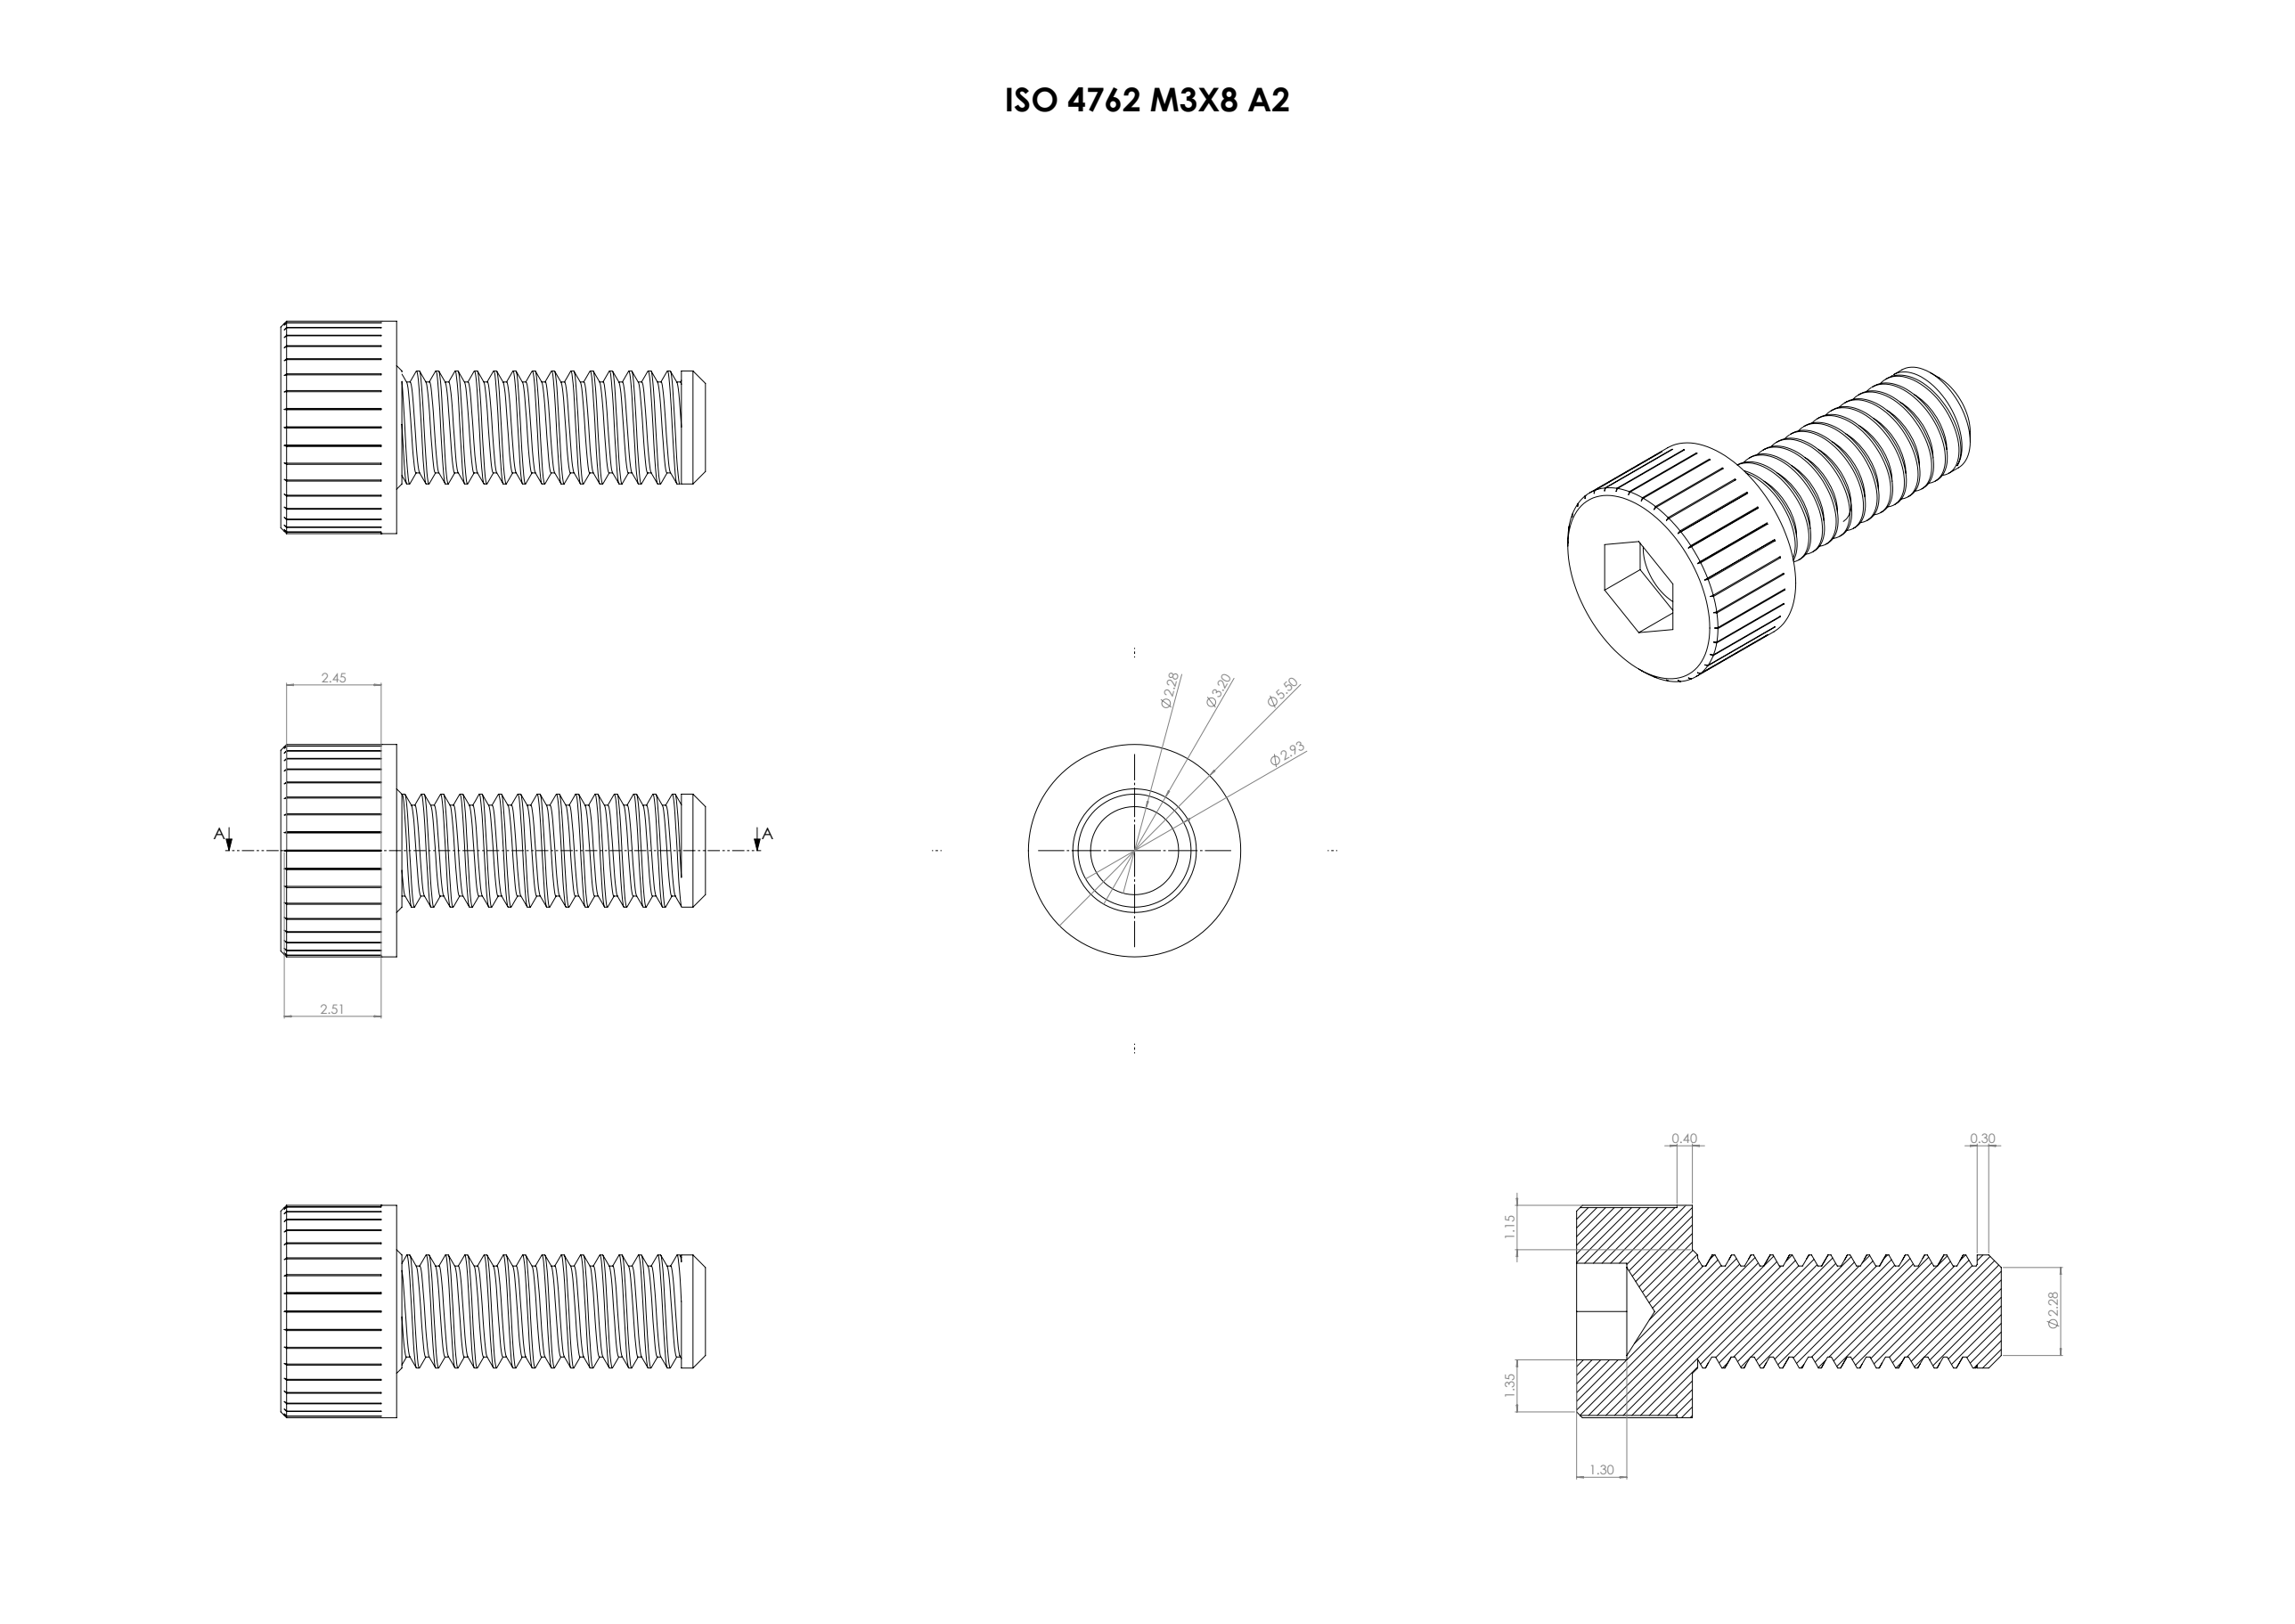
ISO-10303-21;
HEADER;
/* Generated by software containing ST-Developer
 * from STEP Tools, Inc. (www.steptools.com) 
 */

FILE_DESCRIPTION(
/* description */ (''),
/* implementation_level */ '2;1');

FILE_NAME(
/* name */ '14_ISO_4762_M3x8_A2.step',
/* time_stamp */ '2026-10-19T22:59:19-07:00',
/* author */ (''),
/* organization */ (''),
/* preprocessor_version */ 'ST-DEVELOPER v20.2',
/* originating_system */ 'Autodesk Translation Framework v15.15.0.0',
/* authorisation */ '');

FILE_SCHEMA (('AUTOMOTIVE_DESIGN { 1 0 10303 214 3 1 1 }'));
ENDSEC;

DATA;
#10=MECHANICAL_DESIGN_GEOMETRIC_PRESENTATION_REPRESENTATION('',(#924),#53650);
#147=(
BOUNDED_CURVE()
B_SPLINE_CURVE(2,(#40816,#40817,#40818),.UNSPECIFIED.,.F.,.F.)
B_SPLINE_CURVE_WITH_KNOTS((3,3),(0.,0.00848409808460555),.UNSPECIFIED.)
CURVE()
GEOMETRIC_REPRESENTATION_ITEM()
RATIONAL_B_SPLINE_CURVE((1.,1.00016582969981,1.00020138402525))
REPRESENTATION_ITEM('')
);
#148=(
BOUNDED_CURVE()
B_SPLINE_CURVE(2,(#40822,#40823,#40824),.UNSPECIFIED.,.F.,.F.)
B_SPLINE_CURVE_WITH_KNOTS((3,3),(0.0131150022108642,0.0215991002954745),
 .UNSPECIFIED.)
CURVE()
GEOMETRIC_REPRESENTATION_ITEM()
RATIONAL_B_SPLINE_CURVE((1.0002013840307,1.00016582970429,1.))
REPRESENTATION_ITEM('')
);
#149=(
BOUNDED_CURVE()
B_SPLINE_CURVE(2,(#40837,#40838,#40839),.UNSPECIFIED.,.F.,.F.)
B_SPLINE_CURVE_WITH_KNOTS((3,3),(0.,0.0084840980845983),.UNSPECIFIED.)
CURVE()
GEOMETRIC_REPRESENTATION_ITEM()
RATIONAL_B_SPLINE_CURVE((1.,1.00016582970166,1.00020138402749))
REPRESENTATION_ITEM('')
);
#150=(
BOUNDED_CURVE()
B_SPLINE_CURVE(2,(#40843,#40844,#40845),.UNSPECIFIED.,.F.,.F.)
B_SPLINE_CURVE_WITH_KNOTS((3,3),(0.0131150022108621,0.0215991002954745),
 .UNSPECIFIED.)
CURVE()
GEOMETRIC_REPRESENTATION_ITEM()
RATIONAL_B_SPLINE_CURVE((1.00020138404061,1.00016582971246,1.))
REPRESENTATION_ITEM('')
);
#151=(
BOUNDED_CURVE()
B_SPLINE_CURVE(2,(#40858,#40859,#40860),.UNSPECIFIED.,.F.,.F.)
B_SPLINE_CURVE_WITH_KNOTS((3,3),(0.,0.0084840980847528),.UNSPECIFIED.)
CURVE()
GEOMETRIC_REPRESENTATION_ITEM()
RATIONAL_B_SPLINE_CURVE((1.,1.00016582970549,1.00020138403215))
REPRESENTATION_ITEM('')
);
#152=(
BOUNDED_CURVE()
B_SPLINE_CURVE(2,(#40864,#40865,#40866),.UNSPECIFIED.,.F.,.F.)
B_SPLINE_CURVE_WITH_KNOTS((3,3),(0.0131150022108369,0.0215991002954744),
 .UNSPECIFIED.)
CURVE()
GEOMETRIC_REPRESENTATION_ITEM()
RATIONAL_B_SPLINE_CURVE((1.00020138403309,1.00016582970627,1.))
REPRESENTATION_ITEM('')
);
#153=(
BOUNDED_CURVE()
B_SPLINE_CURVE(2,(#40879,#40880,#40881),.UNSPECIFIED.,.F.,.F.)
B_SPLINE_CURVE_WITH_KNOTS((3,3),(0.,0.00848409808456441),.UNSPECIFIED.)
CURVE()
GEOMETRIC_REPRESENTATION_ITEM()
RATIONAL_B_SPLINE_CURVE((1.,1.00016582971128,1.00020138403918))
REPRESENTATION_ITEM('')
);
#154=(
BOUNDED_CURVE()
B_SPLINE_CURVE(2,(#40885,#40886,#40887),.UNSPECIFIED.,.F.,.F.)
B_SPLINE_CURVE_WITH_KNOTS((3,3),(0.0131150022107445,0.0215991002954745),
 .UNSPECIFIED.)
CURVE()
GEOMETRIC_REPRESENTATION_ITEM()
RATIONAL_B_SPLINE_CURVE((1.00020138401994,1.00016582969544,1.))
REPRESENTATION_ITEM('')
);
#155=(
BOUNDED_CURVE()
B_SPLINE_CURVE(2,(#40900,#40901,#40902),.UNSPECIFIED.,.F.,.F.)
B_SPLINE_CURVE_WITH_KNOTS((3,3),(0.,0.00848409808454028),.UNSPECIFIED.)
CURVE()
GEOMETRIC_REPRESENTATION_ITEM()
RATIONAL_B_SPLINE_CURVE((1.,1.00016582970383,1.00020138403013))
REPRESENTATION_ITEM('')
);
#156=(
BOUNDED_CURVE()
B_SPLINE_CURVE(2,(#40906,#40907,#40908),.UNSPECIFIED.,.F.,.F.)
B_SPLINE_CURVE_WITH_KNOTS((3,3),(0.0131150022108609,0.0215991002954744),
 .UNSPECIFIED.)
CURVE()
GEOMETRIC_REPRESENTATION_ITEM()
RATIONAL_B_SPLINE_CURVE((1.00020138403313,1.0001658297063,1.))
REPRESENTATION_ITEM('')
);
#157=(
BOUNDED_CURVE()
B_SPLINE_CURVE(2,(#40921,#40922,#40923),.UNSPECIFIED.,.F.,.F.)
B_SPLINE_CURVE_WITH_KNOTS((3,3),(0.,0.00848409808447202),.UNSPECIFIED.)
CURVE()
GEOMETRIC_REPRESENTATION_ITEM()
RATIONAL_B_SPLINE_CURVE((1.,1.00016582970768,1.00020138403481))
REPRESENTATION_ITEM('')
);
#158=(
BOUNDED_CURVE()
B_SPLINE_CURVE(2,(#40927,#40928,#40929),.UNSPECIFIED.,.F.,.F.)
B_SPLINE_CURVE_WITH_KNOTS((3,3),(0.0131150022108224,0.0215991002954744),
 .UNSPECIFIED.)
CURVE()
GEOMETRIC_REPRESENTATION_ITEM()
RATIONAL_B_SPLINE_CURVE((1.00020138403609,1.00016582970874,1.))
REPRESENTATION_ITEM('')
);
#159=(
BOUNDED_CURVE()
B_SPLINE_CURVE(2,(#40942,#40943,#40944),.UNSPECIFIED.,.F.,.F.)
B_SPLINE_CURVE_WITH_KNOTS((3,3),(0.,0.00848409808427833),.UNSPECIFIED.)
CURVE()
GEOMETRIC_REPRESENTATION_ITEM()
RATIONAL_B_SPLINE_CURVE((1.,1.00016582970634,1.00020138403319))
REPRESENTATION_ITEM('')
);
#160=(
BOUNDED_CURVE()
B_SPLINE_CURVE(2,(#40948,#40949,#40950),.UNSPECIFIED.,.F.,.F.)
B_SPLINE_CURVE_WITH_KNOTS((3,3),(0.013115002210556,0.0215991002954744),
 .UNSPECIFIED.)
CURVE()
GEOMETRIC_REPRESENTATION_ITEM()
RATIONAL_B_SPLINE_CURVE((1.00020138403007,1.00016582970378,1.))
REPRESENTATION_ITEM('')
);
#161=(
BOUNDED_CURVE()
B_SPLINE_CURVE(2,(#40963,#40964,#40965),.UNSPECIFIED.,.F.,.F.)
B_SPLINE_CURVE_WITH_KNOTS((3,3),(0.,0.00848409808441644),.UNSPECIFIED.)
CURVE()
GEOMETRIC_REPRESENTATION_ITEM()
RATIONAL_B_SPLINE_CURVE((1.,1.00016582971078,1.00020138403858))
REPRESENTATION_ITEM('')
);
#162=(
BOUNDED_CURVE()
B_SPLINE_CURVE(2,(#40969,#40970,#40971),.UNSPECIFIED.,.F.,.F.)
B_SPLINE_CURVE_WITH_KNOTS((3,3),(0.0131150022111809,0.0215991002954744),
 .UNSPECIFIED.)
CURVE()
GEOMETRIC_REPRESENTATION_ITEM()
RATIONAL_B_SPLINE_CURVE((1.00020138403856,1.00016582971077,1.))
REPRESENTATION_ITEM('')
);
#163=(
BOUNDED_CURVE()
B_SPLINE_CURVE(2,(#40984,#40985,#40986),.UNSPECIFIED.,.F.,.F.)
B_SPLINE_CURVE_WITH_KNOTS((3,3),(0.,0.00848409808461716),.UNSPECIFIED.)
CURVE()
GEOMETRIC_REPRESENTATION_ITEM()
RATIONAL_B_SPLINE_CURVE((1.,1.00016582970495,1.00020138403149))
REPRESENTATION_ITEM('')
);
#164=(
BOUNDED_CURVE()
B_SPLINE_CURVE(2,(#40990,#40991,#40992),.UNSPECIFIED.,.F.,.F.)
B_SPLINE_CURVE_WITH_KNOTS((3,3),(0.0131150022109262,0.0215991002954744),
 .UNSPECIFIED.)
CURVE()
GEOMETRIC_REPRESENTATION_ITEM()
RATIONAL_B_SPLINE_CURVE((1.00020138404239,1.00016582971392,1.))
REPRESENTATION_ITEM('')
);
#165=(
BOUNDED_CURVE()
B_SPLINE_CURVE(2,(#41005,#41006,#41007),.UNSPECIFIED.,.F.,.F.)
B_SPLINE_CURVE_WITH_KNOTS((3,3),(0.,0.00848409808431464),.UNSPECIFIED.)
CURVE()
GEOMETRIC_REPRESENTATION_ITEM()
RATIONAL_B_SPLINE_CURVE((1.,1.00016582970871,1.00020138403606))
REPRESENTATION_ITEM('')
);
#166=(
BOUNDED_CURVE()
B_SPLINE_CURVE(2,(#41011,#41012,#41013),.UNSPECIFIED.,.F.,.F.)
B_SPLINE_CURVE_WITH_KNOTS((3,3),(0.0131150022106601,0.0215991002954745),
 .UNSPECIFIED.)
CURVE()
GEOMETRIC_REPRESENTATION_ITEM()
RATIONAL_B_SPLINE_CURVE((1.00020138402617,1.00016582970057,1.))
REPRESENTATION_ITEM('')
);
#167=(
BOUNDED_CURVE()
B_SPLINE_CURVE(2,(#41026,#41027,#41028),.UNSPECIFIED.,.F.,.F.)
B_SPLINE_CURVE_WITH_KNOTS((3,3),(0.,0.00848409808479875),.UNSPECIFIED.)
CURVE()
GEOMETRIC_REPRESENTATION_ITEM()
RATIONAL_B_SPLINE_CURVE((1.,1.00016582970535,1.00020138403197))
REPRESENTATION_ITEM('')
);
#168=(
BOUNDED_CURVE()
B_SPLINE_CURVE(2,(#41032,#41033,#41034),.UNSPECIFIED.,.F.,.F.)
B_SPLINE_CURVE_WITH_KNOTS((3,3),(0.0131150022108306,0.0215991002954744),
 .UNSPECIFIED.)
CURVE()
GEOMETRIC_REPRESENTATION_ITEM()
RATIONAL_B_SPLINE_CURVE((1.00020138403405,1.00016582970706,1.))
REPRESENTATION_ITEM('')
);
#169=(
BOUNDED_CURVE()
B_SPLINE_CURVE(2,(#41047,#41048,#41049),.UNSPECIFIED.,.F.,.F.)
B_SPLINE_CURVE_WITH_KNOTS((3,3),(0.,0.0084840980847528),.UNSPECIFIED.)
CURVE()
GEOMETRIC_REPRESENTATION_ITEM()
RATIONAL_B_SPLINE_CURVE((1.,1.00016582970549,1.00020138403215))
REPRESENTATION_ITEM('')
);
#170=(
BOUNDED_CURVE()
B_SPLINE_CURVE(2,(#41053,#41054,#41055),.UNSPECIFIED.,.F.,.F.)
B_SPLINE_CURVE_WITH_KNOTS((3,3),(0.0131150022108369,0.0215991002954744),
 .UNSPECIFIED.)
CURVE()
GEOMETRIC_REPRESENTATION_ITEM()
RATIONAL_B_SPLINE_CURVE((1.00020138403309,1.00016582970627,1.))
REPRESENTATION_ITEM('')
);
#171=(
BOUNDED_CURVE()
B_SPLINE_CURVE(2,(#41068,#41069,#41070),.UNSPECIFIED.,.F.,.F.)
B_SPLINE_CURVE_WITH_KNOTS((3,3),(0.,0.0084840980842322),.UNSPECIFIED.)
CURVE()
GEOMETRIC_REPRESENTATION_ITEM()
RATIONAL_B_SPLINE_CURVE((1.,1.00016582971394,1.00020138404241))
REPRESENTATION_ITEM('')
);
#172=(
BOUNDED_CURVE()
B_SPLINE_CURVE(2,(#41074,#41075,#41076),.UNSPECIFIED.,.F.,.F.)
B_SPLINE_CURVE_WITH_KNOTS((3,3),(0.0131150022105481,0.0215991002954744),
 .UNSPECIFIED.)
CURVE()
GEOMETRIC_REPRESENTATION_ITEM()
RATIONAL_B_SPLINE_CURVE((1.00020138402709,1.00016582970133,1.))
REPRESENTATION_ITEM('')
);
#173=(
BOUNDED_CURVE()
B_SPLINE_CURVE(2,(#41089,#41090,#41091),.UNSPECIFIED.,.F.,.F.)
B_SPLINE_CURVE_WITH_KNOTS((3,3),(0.,0.00848409808414784),.UNSPECIFIED.)
CURVE()
GEOMETRIC_REPRESENTATION_ITEM()
RATIONAL_B_SPLINE_CURVE((1.,1.00016582970969,1.00020138403725))
REPRESENTATION_ITEM('')
);
#174=(
BOUNDED_CURVE()
B_SPLINE_CURVE(2,(#41095,#41096,#41097),.UNSPECIFIED.,.F.,.F.)
B_SPLINE_CURVE_WITH_KNOTS((3,3),(0.0131150022106295,0.0215991002954744),
 .UNSPECIFIED.)
CURVE()
GEOMETRIC_REPRESENTATION_ITEM()
RATIONAL_B_SPLINE_CURVE((1.00020138402686,1.00016582970114,1.))
REPRESENTATION_ITEM('')
);
#175=(
BOUNDED_CURVE()
B_SPLINE_CURVE(2,(#41110,#41111,#41112),.UNSPECIFIED.,.F.,.F.)
B_SPLINE_CURVE_WITH_KNOTS((3,3),(0.,0.00848409808445945),.UNSPECIFIED.)
CURVE()
GEOMETRIC_REPRESENTATION_ITEM()
RATIONAL_B_SPLINE_CURVE((1.,1.00016582971029,1.00020138403798))
REPRESENTATION_ITEM('')
);
#176=(
BOUNDED_CURVE()
B_SPLINE_CURVE(2,(#41116,#41117,#41118),.UNSPECIFIED.,.F.,.F.)
B_SPLINE_CURVE_WITH_KNOTS((3,3),(0.0131150022108553,0.0215991002954744),
 .UNSPECIFIED.)
CURVE()
GEOMETRIC_REPRESENTATION_ITEM()
RATIONAL_B_SPLINE_CURVE((1.00020138402807,1.00016582970213,1.))
REPRESENTATION_ITEM('')
);
#177=(
BOUNDED_CURVE()
B_SPLINE_CURVE(2,(#41131,#41132,#41133),.UNSPECIFIED.,.F.,.F.)
B_SPLINE_CURVE_WITH_KNOTS((3,3),(0.,0.00848409808448244),.UNSPECIFIED.)
CURVE()
GEOMETRIC_REPRESENTATION_ITEM()
RATIONAL_B_SPLINE_CURVE((1.,1.00016582970044,1.00020138402602))
REPRESENTATION_ITEM('')
);
#178=(
BOUNDED_CURVE()
B_SPLINE_CURVE(2,(#41137,#41138,#41139),.UNSPECIFIED.,.F.,.F.)
B_SPLINE_CURVE_WITH_KNOTS((3,3),(0.0131150022107,0.0215991002954745),
 .UNSPECIFIED.)
CURVE()
GEOMETRIC_REPRESENTATION_ITEM()
RATIONAL_B_SPLINE_CURVE((1.00020138402745,1.00016582970163,1.))
REPRESENTATION_ITEM('')
);
#179=(
BOUNDED_CURVE()
B_SPLINE_CURVE(2,(#41152,#41153,#41154),.UNSPECIFIED.,.F.,.F.)
B_SPLINE_CURVE_WITH_KNOTS((3,3),(0.,0.0084840980844404),.UNSPECIFIED.)
CURVE()
GEOMETRIC_REPRESENTATION_ITEM()
RATIONAL_B_SPLINE_CURVE((1.,1.00016582969984,1.00020138402529))
REPRESENTATION_ITEM('')
);
#180=(
BOUNDED_CURVE()
B_SPLINE_CURVE(2,(#41158,#41159,#41160),.UNSPECIFIED.,.F.,.F.)
B_SPLINE_CURVE_WITH_KNOTS((3,3),(0.0131150022109728,0.0215991002954744),
 .UNSPECIFIED.)
CURVE()
GEOMETRIC_REPRESENTATION_ITEM()
RATIONAL_B_SPLINE_CURVE((1.00020138403593,1.0001658297086,1.))
REPRESENTATION_ITEM('')
);
#181=(
BOUNDED_CURVE()
B_SPLINE_CURVE(2,(#41175,#41176,#41177),.UNSPECIFIED.,.F.,.F.)
B_SPLINE_CURVE_WITH_KNOTS((3,3),(0.,0.00848409808461716),.UNSPECIFIED.)
CURVE()
GEOMETRIC_REPRESENTATION_ITEM()
RATIONAL_B_SPLINE_CURVE((1.,1.00016582970494,1.00020138403149))
REPRESENTATION_ITEM('')
);
#182=(
BOUNDED_CURVE()
B_SPLINE_CURVE(2,(#41181,#41182,#41183),.UNSPECIFIED.,.F.,.F.)
B_SPLINE_CURVE_WITH_KNOTS((3,3),(0.0131150022107313,0.0215991002954744),
 .UNSPECIFIED.)
CURVE()
GEOMETRIC_REPRESENTATION_ITEM()
RATIONAL_B_SPLINE_CURVE((1.00020138404435,1.00016582971554,1.))
REPRESENTATION_ITEM('')
);
#183=(
BOUNDED_CURVE()
B_SPLINE_CURVE(2,(#41196,#41197,#41198),.UNSPECIFIED.,.F.,.F.)
B_SPLINE_CURVE_WITH_KNOTS((3,3),(0.,0.0084840980847339),.UNSPECIFIED.)
CURVE()
GEOMETRIC_REPRESENTATION_ITEM()
RATIONAL_B_SPLINE_CURVE((1.,1.00016582970597,1.00020138403273))
REPRESENTATION_ITEM('')
);
#184=(
BOUNDED_CURVE()
B_SPLINE_CURVE(2,(#41202,#41203,#41204),.UNSPECIFIED.,.F.,.F.)
B_SPLINE_CURVE_WITH_KNOTS((3,3),(0.0131150022106966,0.0215991002954744),
 .UNSPECIFIED.)
CURVE()
GEOMETRIC_REPRESENTATION_ITEM()
RATIONAL_B_SPLINE_CURVE((1.00020138403392,1.00016582970695,1.))
REPRESENTATION_ITEM('')
);
#185=(
BOUNDED_CURVE()
B_SPLINE_CURVE(2,(#41217,#41218,#41219),.UNSPECIFIED.,.F.,.F.)
B_SPLINE_CURVE_WITH_KNOTS((3,3),(0.,0.00848409808458664),.UNSPECIFIED.)
CURVE()
GEOMETRIC_REPRESENTATION_ITEM()
RATIONAL_B_SPLINE_CURVE((1.,1.00016582970477,1.00020138403127))
REPRESENTATION_ITEM('')
);
#186=(
BOUNDED_CURVE()
B_SPLINE_CURVE(2,(#41223,#41224,#41225),.UNSPECIFIED.,.F.,.F.)
B_SPLINE_CURVE_WITH_KNOTS((3,3),(0.0131150022108393,0.0215991002954745),
 .UNSPECIFIED.)
CURVE()
GEOMETRIC_REPRESENTATION_ITEM()
RATIONAL_B_SPLINE_CURVE((1.00020138403572,1.00016582970843,1.))
REPRESENTATION_ITEM('')
);
#187=(
BOUNDED_CURVE()
B_SPLINE_CURVE(2,(#41238,#41239,#41240),.UNSPECIFIED.,.F.,.F.)
B_SPLINE_CURVE_WITH_KNOTS((3,3),(0.,0.00848409808463718),.UNSPECIFIED.)
CURVE()
GEOMETRIC_REPRESENTATION_ITEM()
RATIONAL_B_SPLINE_CURVE((1.,1.00016582970055,1.00020138402615))
REPRESENTATION_ITEM('')
);
#188=(
BOUNDED_CURVE()
B_SPLINE_CURVE(2,(#41244,#41245,#41246),.UNSPECIFIED.,.F.,.F.)
B_SPLINE_CURVE_WITH_KNOTS((3,3),(0.013115002211021,0.0215991002954743),
 .UNSPECIFIED.)
CURVE()
GEOMETRIC_REPRESENTATION_ITEM()
RATIONAL_B_SPLINE_CURVE((1.00020138403351,1.00016582970661,1.))
REPRESENTATION_ITEM('')
);
#189=(
BOUNDED_CURVE()
B_SPLINE_CURVE(2,(#41259,#41260,#41261),.UNSPECIFIED.,.F.,.F.)
B_SPLINE_CURVE_WITH_KNOTS((3,3),(0.,0.0084840980842322),.UNSPECIFIED.)
CURVE()
GEOMETRIC_REPRESENTATION_ITEM()
RATIONAL_B_SPLINE_CURVE((1.,1.00016582971394,1.00020138404241))
REPRESENTATION_ITEM('')
);
#190=(
BOUNDED_CURVE()
B_SPLINE_CURVE(2,(#41265,#41266,#41267),.UNSPECIFIED.,.F.,.F.)
B_SPLINE_CURVE_WITH_KNOTS((3,3),(0.0131150022105481,0.0215991002954744),
 .UNSPECIFIED.)
CURVE()
GEOMETRIC_REPRESENTATION_ITEM()
RATIONAL_B_SPLINE_CURVE((1.00020138402709,1.00016582970133,1.))
REPRESENTATION_ITEM('')
);
#191=(
BOUNDED_CURVE()
B_SPLINE_CURVE(2,(#41280,#41281,#41282),.UNSPECIFIED.,.F.,.F.)
B_SPLINE_CURVE_WITH_KNOTS((3,3),(0.,0.00848409808456074),.UNSPECIFIED.)
CURVE()
GEOMETRIC_REPRESENTATION_ITEM()
RATIONAL_B_SPLINE_CURVE((1.,1.00016582970947,1.00020138403699))
REPRESENTATION_ITEM('')
);
#192=(
BOUNDED_CURVE()
B_SPLINE_CURVE(2,(#41286,#41287,#41288),.UNSPECIFIED.,.F.,.F.)
B_SPLINE_CURVE_WITH_KNOTS((3,3),(0.0131150022109338,0.0215991002954745),
 .UNSPECIFIED.)
CURVE()
GEOMETRIC_REPRESENTATION_ITEM()
RATIONAL_B_SPLINE_CURVE((1.00020138403466,1.00016582970756,1.))
REPRESENTATION_ITEM('')
);
#193=(
BOUNDED_CURVE()
B_SPLINE_CURVE(2,(#41301,#41302,#41303),.UNSPECIFIED.,.F.,.F.)
B_SPLINE_CURVE_WITH_KNOTS((3,3),(0.,0.00848409808446819),.UNSPECIFIED.)
CURVE()
GEOMETRIC_REPRESENTATION_ITEM()
RATIONAL_B_SPLINE_CURVE((1.,1.00016582970737,1.00020138403444))
REPRESENTATION_ITEM('')
);
#194=(
BOUNDED_CURVE()
B_SPLINE_CURVE(2,(#41307,#41308,#41309),.UNSPECIFIED.,.F.,.F.)
B_SPLINE_CURVE_WITH_KNOTS((3,3),(0.0131150022107308,0.0215991002954744),
 .UNSPECIFIED.)
CURVE()
GEOMETRIC_REPRESENTATION_ITEM()
RATIONAL_B_SPLINE_CURVE((1.00020138402973,1.0001658297035,1.))
REPRESENTATION_ITEM('')
);
#195=(
BOUNDED_CURVE()
B_SPLINE_CURVE(2,(#41322,#41323,#41324),.UNSPECIFIED.,.F.,.F.)
B_SPLINE_CURVE_WITH_KNOTS((3,3),(0.,0.00848409808448244),.UNSPECIFIED.)
CURVE()
GEOMETRIC_REPRESENTATION_ITEM()
RATIONAL_B_SPLINE_CURVE((1.,1.00016582970044,1.00020138402602))
REPRESENTATION_ITEM('')
);
#196=(
BOUNDED_CURVE()
B_SPLINE_CURVE(2,(#41328,#41329,#41330),.UNSPECIFIED.,.F.,.F.)
B_SPLINE_CURVE_WITH_KNOTS((3,3),(0.0131150022107,0.0215991002954745),
 .UNSPECIFIED.)
CURVE()
GEOMETRIC_REPRESENTATION_ITEM()
RATIONAL_B_SPLINE_CURVE((1.00020138402745,1.00016582970163,1.))
REPRESENTATION_ITEM('')
);
#197=(
BOUNDED_CURVE()
B_SPLINE_CURVE(2,(#41343,#41344,#41345),.UNSPECIFIED.,.F.,.F.)
B_SPLINE_CURVE_WITH_KNOTS((3,3),(0.,0.00848409808441086),.UNSPECIFIED.)
CURVE()
GEOMETRIC_REPRESENTATION_ITEM()
RATIONAL_B_SPLINE_CURVE((1.,1.00016582971069,1.00020138403846))
REPRESENTATION_ITEM('')
);
#198=(
BOUNDED_CURVE()
B_SPLINE_CURVE(2,(#41349,#41350,#41351),.UNSPECIFIED.,.F.,.F.)
B_SPLINE_CURVE_WITH_KNOTS((3,3),(0.0131150022109839,0.0215991002954745),
 .UNSPECIFIED.)
CURVE()
GEOMETRIC_REPRESENTATION_ITEM()
RATIONAL_B_SPLINE_CURVE((1.00020138402514,1.00016582969972,1.))
REPRESENTATION_ITEM('')
);
#199=(
BOUNDED_CURVE()
B_SPLINE_CURVE(2,(#41364,#41365,#41366),.UNSPECIFIED.,.F.,.F.)
B_SPLINE_CURVE_WITH_KNOTS((3,3),(0.,0.00848409808461089),.UNSPECIFIED.)
CURVE()
GEOMETRIC_REPRESENTATION_ITEM()
RATIONAL_B_SPLINE_CURVE((1.,1.00016582970996,1.00020138403757))
REPRESENTATION_ITEM('')
);
#200=(
BOUNDED_CURVE()
B_SPLINE_CURVE(2,(#41370,#41371,#41372),.UNSPECIFIED.,.F.,.F.)
B_SPLINE_CURVE_WITH_KNOTS((3,3),(0.0131150022107081,0.0215991002954744),
 .UNSPECIFIED.)
CURVE()
GEOMETRIC_REPRESENTATION_ITEM()
RATIONAL_B_SPLINE_CURVE((1.00020138403464,1.00016582970754,1.))
REPRESENTATION_ITEM('')
);
#201=(
BOUNDED_CURVE()
B_SPLINE_CURVE(2,(#41385,#41386,#41387),.UNSPECIFIED.,.F.,.F.)
B_SPLINE_CURVE_WITH_KNOTS((3,3),(0.,0.00848409808429742),.UNSPECIFIED.)
CURVE()
GEOMETRIC_REPRESENTATION_ITEM()
RATIONAL_B_SPLINE_CURVE((1.,1.00016582971405,1.00020138404255))
REPRESENTATION_ITEM('')
);
#202=(
BOUNDED_CURVE()
B_SPLINE_CURVE(2,(#41391,#41392,#41393),.UNSPECIFIED.,.F.,.F.)
B_SPLINE_CURVE_WITH_KNOTS((3,3),(0.0131150022109026,0.0215991002954744),
 .UNSPECIFIED.)
CURVE()
GEOMETRIC_REPRESENTATION_ITEM()
RATIONAL_B_SPLINE_CURVE((1.00020138403953,1.00016582971157,1.))
REPRESENTATION_ITEM('')
);
#203=(
BOUNDED_CURVE()
B_SPLINE_CURVE(2,(#41406,#41407,#41408),.UNSPECIFIED.,.F.,.F.)
B_SPLINE_CURVE_WITH_KNOTS((3,3),(0.,0.00848409808458664),.UNSPECIFIED.)
CURVE()
GEOMETRIC_REPRESENTATION_ITEM()
RATIONAL_B_SPLINE_CURVE((1.,1.00016582970477,1.00020138403127))
REPRESENTATION_ITEM('')
);
#204=(
BOUNDED_CURVE()
B_SPLINE_CURVE(2,(#41412,#41413,#41414),.UNSPECIFIED.,.F.,.F.)
B_SPLINE_CURVE_WITH_KNOTS((3,3),(0.0131150022108393,0.0215991002954745),
 .UNSPECIFIED.)
CURVE()
GEOMETRIC_REPRESENTATION_ITEM()
RATIONAL_B_SPLINE_CURVE((1.00020138403572,1.00016582970843,1.))
REPRESENTATION_ITEM('')
);
#205=(
BOUNDED_CURVE()
B_SPLINE_CURVE(2,(#41427,#41428,#41429),.UNSPECIFIED.,.F.,.F.)
B_SPLINE_CURVE_WITH_KNOTS((3,3),(0.,0.00848409808472772),.UNSPECIFIED.)
CURVE()
GEOMETRIC_REPRESENTATION_ITEM()
RATIONAL_B_SPLINE_CURVE((1.,1.00016582970133,1.0002013840271))
REPRESENTATION_ITEM('')
);
#206=(
BOUNDED_CURVE()
B_SPLINE_CURVE(2,(#41433,#41434,#41435),.UNSPECIFIED.,.F.,.F.)
B_SPLINE_CURVE_WITH_KNOTS((3,3),(0.0131150022106421,0.0215991002954744),
 .UNSPECIFIED.)
CURVE()
GEOMETRIC_REPRESENTATION_ITEM()
RATIONAL_B_SPLINE_CURVE((1.00020138403214,1.00016582970549,1.))
REPRESENTATION_ITEM('')
);
#207=(
BOUNDED_CURVE()
B_SPLINE_CURVE(2,(#41448,#41449,#41450),.UNSPECIFIED.,.F.,.F.)
B_SPLINE_CURVE_WITH_KNOTS((3,3),(0.,0.00848409808461495),.UNSPECIFIED.)
CURVE()
GEOMETRIC_REPRESENTATION_ITEM()
RATIONAL_B_SPLINE_CURVE((1.,1.00016582970949,1.000201384037))
REPRESENTATION_ITEM('')
);
#208=(
BOUNDED_CURVE()
B_SPLINE_CURVE(2,(#41454,#41455,#41456),.UNSPECIFIED.,.F.,.F.)
B_SPLINE_CURVE_WITH_KNOTS((3,3),(0.0131150022109445,0.0215991002954744),
 .UNSPECIFIED.)
CURVE()
GEOMETRIC_REPRESENTATION_ITEM()
RATIONAL_B_SPLINE_CURVE((1.00020138402523,1.00016582969979,1.))
REPRESENTATION_ITEM('')
);
#209=(
BOUNDED_CURVE()
B_SPLINE_CURVE(2,(#41469,#41470,#41471),.UNSPECIFIED.,.F.,.F.)
B_SPLINE_CURVE_WITH_KNOTS((3,3),(0.,0.00848409808414784),.UNSPECIFIED.)
CURVE()
GEOMETRIC_REPRESENTATION_ITEM()
RATIONAL_B_SPLINE_CURVE((1.,1.00016582970969,1.00020138403725))
REPRESENTATION_ITEM('')
);
#210=(
BOUNDED_CURVE()
B_SPLINE_CURVE(2,(#41475,#41476,#41477),.UNSPECIFIED.,.F.,.F.)
B_SPLINE_CURVE_WITH_KNOTS((3,3),(0.0131150022106295,0.0215991002954744),
 .UNSPECIFIED.)
CURVE()
GEOMETRIC_REPRESENTATION_ITEM()
RATIONAL_B_SPLINE_CURVE((1.00020138402686,1.00016582970114,1.))
REPRESENTATION_ITEM('')
);
#211=(
BOUNDED_CURVE()
B_SPLINE_CURVE(2,(#41490,#41491,#41492),.UNSPECIFIED.,.F.,.F.)
B_SPLINE_CURVE_WITH_KNOTS((3,3),(0.,0.00848409808467215),.UNSPECIFIED.)
CURVE()
GEOMETRIC_REPRESENTATION_ITEM()
RATIONAL_B_SPLINE_CURVE((1.,1.00016582970831,1.00020138403558))
REPRESENTATION_ITEM('')
);
#212=(
BOUNDED_CURVE()
B_SPLINE_CURVE(2,(#41496,#41497,#41498),.UNSPECIFIED.,.F.,.F.)
B_SPLINE_CURVE_WITH_KNOTS((3,3),(0.0131150022106657,0.0215991002954744),
 .UNSPECIFIED.)
CURVE()
GEOMETRIC_REPRESENTATION_ITEM()
RATIONAL_B_SPLINE_CURVE((1.00020138402665,1.00016582970096,1.))
REPRESENTATION_ITEM('')
);
#213=(
BOUNDED_CURVE()
B_SPLINE_CURVE(2,(#41511,#41512,#41513),.UNSPECIFIED.,.F.,.F.)
B_SPLINE_CURVE_WITH_KNOTS((3,3),(0.,0.00848409808448244),.UNSPECIFIED.)
CURVE()
GEOMETRIC_REPRESENTATION_ITEM()
RATIONAL_B_SPLINE_CURVE((1.,1.00016582970044,1.00020138402602))
REPRESENTATION_ITEM('')
);
#214=(
BOUNDED_CURVE()
B_SPLINE_CURVE(2,(#41517,#41518,#41519),.UNSPECIFIED.,.F.,.F.)
B_SPLINE_CURVE_WITH_KNOTS((3,3),(0.0131150022107,0.0215991002954745),
 .UNSPECIFIED.)
CURVE()
GEOMETRIC_REPRESENTATION_ITEM()
RATIONAL_B_SPLINE_CURVE((1.00020138402745,1.00016582970163,1.))
REPRESENTATION_ITEM('')
);
#215=(
BOUNDED_CURVE()
B_SPLINE_CURVE(2,(#41532,#41533,#41534),.UNSPECIFIED.,.F.,.F.)
B_SPLINE_CURVE_WITH_KNOTS((3,3),(0.,0.00848409808462521),.UNSPECIFIED.)
CURVE()
GEOMETRIC_REPRESENTATION_ITEM()
RATIONAL_B_SPLINE_CURVE((1.,1.00016582970203,1.00020138402795))
REPRESENTATION_ITEM('')
);
#216=(
BOUNDED_CURVE()
B_SPLINE_CURVE(2,(#41538,#41539,#41540),.UNSPECIFIED.,.F.,.F.)
B_SPLINE_CURVE_WITH_KNOTS((3,3),(0.0131150022109901,0.0215991002954744),
 .UNSPECIFIED.)
CURVE()
GEOMETRIC_REPRESENTATION_ITEM()
RATIONAL_B_SPLINE_CURVE((1.00020138403892,1.00016582971107,1.))
REPRESENTATION_ITEM('')
);
#217=(
BOUNDED_CURVE()
B_SPLINE_CURVE(2,(#41593,#41594,#41595),.UNSPECIFIED.,.F.,.F.)
B_SPLINE_CURVE_WITH_KNOTS((3,3),(0.,0.0084840980844225),.UNSPECIFIED.)
CURVE()
GEOMETRIC_REPRESENTATION_ITEM()
RATIONAL_B_SPLINE_CURVE((1.,1.00016582970633,1.00020138403317))
REPRESENTATION_ITEM('')
);
#218=(
BOUNDED_CURVE()
B_SPLINE_CURVE(2,(#41597,#41598,#41599),.UNSPECIFIED.,.F.,.F.)
B_SPLINE_CURVE_WITH_KNOTS((3,3),(0.0131150022108769,0.0215991002954744),
 .UNSPECIFIED.)
CURVE()
GEOMETRIC_REPRESENTATION_ITEM()
RATIONAL_B_SPLINE_CURVE((1.00020138402781,1.00016582970192,1.))
REPRESENTATION_ITEM('')
);
#367=B_SPLINE_SURFACE_WITH_KNOTS('',3,3,((#39875,#39876,#39877,#39878,#39879,
#39880,#39881,#39882,#39883,#39884,#39885,#39886,#39887,#39888,#39889,#39890,
#39891,#39892,#39893,#39894,#39895,#39896,#39897,#39898,#39899,#39900,#39901,
#39902,#39903,#39904,#39905,#39906,#39907,#39908,#39909,#39910,#39911,#39912,
#39913,#39914,#39915,#39916,#39917,#39918,#39919,#39920,#39921,#39922,#39923,
#39924,#39925,#39926,#39927,#39928,#39929,#39930,#39931,#39932,#39933,#39934,
#39935,#39936,#39937,#39938,#39939,#39940,#39941,#39942,#39943,#39944,#39945,
#39946,#39947,#39948,#39949,#39950,#39951,#39952,#39953,#39954,#39955,#39956,
#39957,#39958,#39959,#39960,#39961,#39962,#39963,#39964,#39965,#39966,#39967,
#39968,#39969,#39970,#39971),(#39972,#39973,#39974,#39975,#39976,#39977,
#39978,#39979,#39980,#39981,#39982,#39983,#39984,#39985,#39986,#39987,#39988,
#39989,#39990,#39991,#39992,#39993,#39994,#39995,#39996,#39997,#39998,#39999,
#40000,#40001,#40002,#40003,#40004,#40005,#40006,#40007,#40008,#40009,#40010,
#40011,#40012,#40013,#40014,#40015,#40016,#40017,#40018,#40019,#40020,#40021,
#40022,#40023,#40024,#40025,#40026,#40027,#40028,#40029,#40030,#40031,#40032,
#40033,#40034,#40035,#40036,#40037,#40038,#40039,#40040,#40041,#40042,#40043,
#40044,#40045,#40046,#40047,#40048,#40049,#40050,#40051,#40052,#40053,#40054,
#40055,#40056,#40057,#40058,#40059,#40060,#40061,#40062,#40063,#40064,#40065,
#40066,#40067,#40068),(#40069,#40070,#40071,#40072,#40073,#40074,#40075,
#40076,#40077,#40078,#40079,#40080,#40081,#40082,#40083,#40084,#40085,#40086,
#40087,#40088,#40089,#40090,#40091,#40092,#40093,#40094,#40095,#40096,#40097,
#40098,#40099,#40100,#40101,#40102,#40103,#40104,#40105,#40106,#40107,#40108,
#40109,#40110,#40111,#40112,#40113,#40114,#40115,#40116,#40117,#40118,#40119,
#40120,#40121,#40122,#40123,#40124,#40125,#40126,#40127,#40128,#40129,#40130,
#40131,#40132,#40133,#40134,#40135,#40136,#40137,#40138,#40139,#40140,#40141,
#40142,#40143,#40144,#40145,#40146,#40147,#40148,#40149,#40150,#40151,#40152,
#40153,#40154,#40155,#40156,#40157,#40158,#40159,#40160,#40161,#40162,#40163,
#40164,#40165),(#40166,#40167,#40168,#40169,#40170,#40171,#40172,#40173,
#40174,#40175,#40176,#40177,#40178,#40179,#40180,#40181,#40182,#40183,#40184,
#40185,#40186,#40187,#40188,#40189,#40190,#40191,#40192,#40193,#40194,#40195,
#40196,#40197,#40198,#40199,#40200,#40201,#40202,#40203,#40204,#40205,#40206,
#40207,#40208,#40209,#40210,#40211,#40212,#40213,#40214,#40215,#40216,#40217,
#40218,#40219,#40220,#40221,#40222,#40223,#40224,#40225,#40226,#40227,#40228,
#40229,#40230,#40231,#40232,#40233,#40234,#40235,#40236,#40237,#40238,#40239,
#40240,#40241,#40242,#40243,#40244,#40245,#40246,#40247,#40248,#40249,#40250,
#40251,#40252,#40253,#40254,#40255,#40256,#40257,#40258,#40259,#40260,#40261,
#40262)),.UNSPECIFIED.,.F.,.F.,.F.,(4,4),(4,1,1,1,1,1,1,1,1,1,1,1,1,1,1,
1,1,1,1,1,1,1,1,1,1,1,1,1,1,1,1,1,1,1,1,1,1,1,1,1,1,1,1,1,1,1,1,1,1,1,1,
1,1,1,1,1,1,1,1,1,1,1,1,1,1,1,1,1,1,1,1,1,1,1,1,1,1,1,1,1,1,1,1,1,1,1,1,
1,1,1,1,1,1,1,4),(0.,0.0329955678841871),(12.071947338616,13.0618802739488,
14.0518132092816,15.0417461446143,16.0316790799471,17.0216120152799,18.0115449506126,
19.0014778859454,19.9914108212782,20.981343756611,21.9712766919437,22.9612096272765,
23.9511425626093,24.941075497942,25.9310084332748,26.9209413686076,27.9108743039403,
28.9008072392731,29.8907401746059,30.8806731099386,31.8706060452714,32.8605389806042,
33.8504719159369,34.8404048512697,35.8303377866025,36.8202707219352,37.810203657268,
38.8001365926008,39.7900695279335,40.7800024632663,41.7699353985991,42.7598683339318,
43.7498012692646,44.7397342045974,45.7296671399301,46.7196000752629,47.7095330105957,
48.6994659459284,49.6893988812612,50.679331816594,51.6692647519267,52.6591976872595,
53.6491306225923,54.639063557925,55.6289964932578,56.6189294285906,57.6088623639234,
58.5987952992561,59.5887282345889,60.5786611699216,61.5685941052544,62.5585270405872,
63.54845997592,64.5383929112527,65.5283258465855,66.5182587819182,67.508191717251,
68.4981246525838,69.4880575879166,70.4779905232493,71.4679234585821,72.4578563939149,
73.4477893292476,74.4377222645804,75.4276551999132,76.4175881352459,77.4075210705787,
78.3974540059115,79.3873869412442,80.377319876577,81.3672528119098,82.3571857472425,
83.3471186825753,84.3370516179081,85.3269845532408,86.3169174885736,87.3068504239064,
88.2967833592391,89.2867162945719,90.2766492299047,91.2665821652374,92.2565151005702,
93.246448035903,94.2363809712357,95.2263139065685,96.2162468419013,97.206179777234,
98.1961127125668,99.1860456478996,100.175978583232,101.165911518565,102.155844453898,
103.145777389231,104.135710324563,105.125643259896),.UNSPECIFIED.);
#368=B_SPLINE_SURFACE_WITH_KNOTS('',3,3,((#40400,#40401,#40402,#40403,#40404,
#40405,#40406,#40407,#40408,#40409,#40410,#40411,#40412,#40413,#40414,#40415,
#40416,#40417,#40418,#40419,#40420,#40421,#40422,#40423,#40424,#40425,#40426,
#40427,#40428,#40429,#40430,#40431,#40432,#40433,#40434,#40435,#40436,#40437,
#40438,#40439,#40440,#40441,#40442,#40443,#40444,#40445,#40446,#40447,#40448,
#40449,#40450,#40451,#40452,#40453,#40454,#40455,#40456,#40457,#40458,#40459,
#40460,#40461,#40462,#40463,#40464,#40465,#40466,#40467,#40468,#40469,#40470,
#40471,#40472,#40473,#40474,#40475,#40476,#40477,#40478,#40479,#40480,#40481,
#40482,#40483,#40484,#40485,#40486,#40487,#40488,#40489,#40490,#40491,#40492,
#40493,#40494,#40495,#40496),(#40497,#40498,#40499,#40500,#40501,#40502,
#40503,#40504,#40505,#40506,#40507,#40508,#40509,#40510,#40511,#40512,#40513,
#40514,#40515,#40516,#40517,#40518,#40519,#40520,#40521,#40522,#40523,#40524,
#40525,#40526,#40527,#40528,#40529,#40530,#40531,#40532,#40533,#40534,#40535,
#40536,#40537,#40538,#40539,#40540,#40541,#40542,#40543,#40544,#40545,#40546,
#40547,#40548,#40549,#40550,#40551,#40552,#40553,#40554,#40555,#40556,#40557,
#40558,#40559,#40560,#40561,#40562,#40563,#40564,#40565,#40566,#40567,#40568,
#40569,#40570,#40571,#40572,#40573,#40574,#40575,#40576,#40577,#40578,#40579,
#40580,#40581,#40582,#40583,#40584,#40585,#40586,#40587,#40588,#40589,#40590,
#40591,#40592,#40593),(#40594,#40595,#40596,#40597,#40598,#40599,#40600,
#40601,#40602,#40603,#40604,#40605,#40606,#40607,#40608,#40609,#40610,#40611,
#40612,#40613,#40614,#40615,#40616,#40617,#40618,#40619,#40620,#40621,#40622,
#40623,#40624,#40625,#40626,#40627,#40628,#40629,#40630,#40631,#40632,#40633,
#40634,#40635,#40636,#40637,#40638,#40639,#40640,#40641,#40642,#40643,#40644,
#40645,#40646,#40647,#40648,#40649,#40650,#40651,#40652,#40653,#40654,#40655,
#40656,#40657,#40658,#40659,#40660,#40661,#40662,#40663,#40664,#40665,#40666,
#40667,#40668,#40669,#40670,#40671,#40672,#40673,#40674,#40675,#40676,#40677,
#40678,#40679,#40680,#40681,#40682,#40683,#40684,#40685,#40686,#40687,#40688,
#40689,#40690),(#40691,#40692,#40693,#40694,#40695,#40696,#40697,#40698,
#40699,#40700,#40701,#40702,#40703,#40704,#40705,#40706,#40707,#40708,#40709,
#40710,#40711,#40712,#40713,#40714,#40715,#40716,#40717,#40718,#40719,#40720,
#40721,#40722,#40723,#40724,#40725,#40726,#40727,#40728,#40729,#40730,#40731,
#40732,#40733,#40734,#40735,#40736,#40737,#40738,#40739,#40740,#40741,#40742,
#40743,#40744,#40745,#40746,#40747,#40748,#40749,#40750,#40751,#40752,#40753,
#40754,#40755,#40756,#40757,#40758,#40759,#40760,#40761,#40762,#40763,#40764,
#40765,#40766,#40767,#40768,#40769,#40770,#40771,#40772,#40773,#40774,#40775,
#40776,#40777,#40778,#40779,#40780,#40781,#40782,#40783,#40784,#40785,#40786,
#40787)),.UNSPECIFIED.,.F.,.F.,.F.,(4,4),(4,1,1,1,1,1,1,1,1,1,1,1,1,1,1,
1,1,1,1,1,1,1,1,1,1,1,1,1,1,1,1,1,1,1,1,1,1,1,1,1,1,1,1,1,1,1,1,1,1,1,1,
1,1,1,1,1,1,1,1,1,1,1,1,1,1,1,1,1,1,1,1,1,1,1,1,1,1,1,1,1,1,1,1,1,1,1,1,
1,1,1,1,1,1,1,4),(0.,0.0329955678841871),(15.3858509318081,16.3757838671408,
17.3657168024736,18.3556497378064,19.3455826731391,20.3355156084719,21.3254485438047,
22.3153814791375,23.3053144144702,24.295247349803,25.2851802851358,26.2751132204685,
27.2650461558013,28.2549790911341,29.2449120264668,30.2348449617996,31.2247778971324,
32.2147108324651,33.2046437677979,34.1945767031307,35.1845096384634,36.1744425737962,
37.164375509129,38.1543084444617,39.1442413797945,40.1341743151273,41.12410725046,
42.1140401857928,43.1039731211256,44.0939060564583,45.0838389917911,46.0737719271239,
47.0637048624566,48.0536377977894,49.0435707331222,50.0335036684549,51.0234366037877,
52.0133695391205,53.0033024744532,53.993235409786,54.9831683451188,55.9731012804516,
56.9630342157843,57.9529671511171,58.9429000864499,59.9328330217826,60.9227659571154,
61.9126988924482,62.9026318277809,63.8925647631137,64.8824976984465,65.8724306337792,
66.862363569112,67.8522965044448,68.8422294397775,69.8321623751103,70.8220953104431,
71.8120282457758,72.8019611811086,73.7918941164414,74.7818270517741,75.7717599871069,
76.7616929224397,77.7516258577724,78.7415587931052,79.731491728438,80.7214246637707,
81.7113575991035,82.7012905344363,83.6912234697691,84.6811564051018,85.6710893404346,
86.6610222757674,87.6509552111001,88.6408881464329,89.6308210817657,90.6207540170984,
91.6106869524312,92.600619887764,93.5905528230967,94.5804857584295,95.5704186937623,
96.560351629095,97.5502845644278,98.5402174997606,99.5301504350933,100.520083370426,
101.510016305759,102.499949241092,103.489882176424,104.479815111757,105.46974804709,
106.459680982423,107.449613917755,108.439546853088),.UNSPECIFIED.);
#489=B_SPLINE_CURVE_WITH_KNOTS('',3,(#38711,#38712,#38713,#38714,#38715,
#38716,#38717,#38718,#38719,#38720,#38721,#38722,#38723,#38724,#38725,#38726),
 .UNSPECIFIED.,.F.,.F.,(4,3,3,3,3,4),(-6.60529764332039,-5.93959761199661,
-4.94966467666384,-3.95973174133107,-2.9697988059983,-2.07317267331972),
 .UNSPECIFIED.);
#490=B_SPLINE_CURVE_WITH_KNOTS('',3,(#38734,#38735,#38736,#38737,#38738,
#38739,#38740,#38741,#38742,#38743,#38744,#38745,#38746),.UNSPECIFIED.,
 .F.,.F.,(4,3,3,3,4),(0.,0.989932935332755,1.97986587066553,2.9697988059983,
3.63601592933276),.UNSPECIFIED.);
#491=B_SPLINE_CURVE_WITH_KNOTS('',3,(#38751,#38752,#38753,#38754,#38755,
#38756,#38757,#38758,#38759,#38760,#38761,#38762,#38763,#38764,#38765,#38766,
#38767,#38768,#38769,#38770,#38771,#38772,#38773,#38774,#38775),
 .UNSPECIFIED.,.F.,.F.,(4,3,3,3,3,3,3,3,4),(-12.8884829505,-12.869128159326,
-11.8791952239932,-10.8892622886604,-9.89932935332768,-8.90939641799491,
-7.91946348266214,-6.92953054732937,-6.60529764332039),.UNSPECIFIED.);
#492=B_SPLINE_CURVE_WITH_KNOTS('',3,(#38776,#38777,#38778,#38779,#38780,
#38781,#38782,#38783,#38784,#38785,#38786,#38787,#38788,#38789,#38790,#38791,
#38792,#38793,#38794,#38795,#38796,#38797,#38798,#38799,#38800),
 .UNSPECIFIED.,.F.,.F.,(4,3,3,3,3,3,3,3,4),(3.63601592933276,3.95973174133107,
4.94966467666384,5.93959761199661,6.92953054732937,7.91946348266214,8.90939641799491,
9.89932935332767,9.91920123651235),.UNSPECIFIED.);
#493=B_SPLINE_CURVE_WITH_KNOTS('',3,(#38805,#38806,#38807,#38808,#38809,
#38810,#38811,#38812,#38813,#38814,#38815,#38816,#38817,#38818,#38819,#38820,
#38821,#38822,#38823,#38824,#38825,#38826),.UNSPECIFIED.,.F.,.F.,(4,3,3,
3,3,3,3,4),(-19.1716682576796,-18.8087257713226,-17.8187928359898,-16.8288599006571,
-15.8389269653243,-14.8489940299915,-13.8590610946588,-12.8884829505),
 .UNSPECIFIED.);
#494=B_SPLINE_CURVE_WITH_KNOTS('',3,(#38827,#38828,#38829,#38830,#38831,
#38832,#38833,#38834,#38835,#38836,#38837,#38838,#38839,#38840,#38841,#38842,
#38843,#38844,#38845,#38846,#38847,#38848),.UNSPECIFIED.,.F.,.F.,(4,3,3,
3,3,3,3,4),(9.91920123651235,10.8892622886604,11.8791952239932,12.869128159326,
13.8590610946587,14.8489940299915,15.8389269653243,16.2023865436919),
 .UNSPECIFIED.);
#495=B_SPLINE_CURVE_WITH_KNOTS('',3,(#38853,#38854,#38855,#38856,#38857,
#38858,#38859,#38860,#38861,#38862,#38863,#38864,#38865,#38866,#38867,#38868,
#38869,#38870,#38871,#38872,#38873,#38874),.UNSPECIFIED.,.F.,.F.,(4,3,3,
3,3,3,3,4),(-25.4548535648592,-24.7483233833192,-23.7583904479864,-22.7684575126537,
-21.7785245773209,-20.7885916419881,-19.7986587066553,-19.1716682576796),
 .UNSPECIFIED.);
#496=B_SPLINE_CURVE_WITH_KNOTS('',3,(#38875,#38876,#38877,#38878,#38879,
#38880,#38881,#38882,#38883,#38884,#38885,#38886,#38887,#38888,#38889,#38890,
#38891,#38892,#38893,#38894,#38895,#38896),.UNSPECIFIED.,.F.,.F.,(4,3,3,
3,3,3,3,4),(16.2023865436919,16.828859900657,17.8187928359898,18.8087257713226,
19.7986587066553,20.7885916419881,21.7785245773209,22.4855718508715),
 .UNSPECIFIED.);
#497=B_SPLINE_CURVE_WITH_KNOTS('',3,(#38901,#38902,#38903,#38904,#38905,
#38906,#38907,#38908,#38909,#38910,#38911,#38912,#38913,#38914,#38915,#38916,
#38917,#38918,#38919,#38920,#38921,#38922,#38923,#38924,#38925),
 .UNSPECIFIED.,.F.,.F.,(4,3,3,3,3,3,3,3,4),(-31.7380388720387,-31.6778539306486,
-30.6879209953158,-29.697988059983,-28.7080551246503,-27.7181221893175,
-26.7281892539847,-25.738256318652,-25.4548535648592),.UNSPECIFIED.);
#498=B_SPLINE_CURVE_WITH_KNOTS('',3,(#38926,#38927,#38928,#38929,#38930,
#38931,#38932,#38933,#38934,#38935,#38936,#38937,#38938,#38939,#38940,#38941,
#38942,#38943,#38944,#38945,#38946,#38947,#38948,#38949,#38950),
 .UNSPECIFIED.,.F.,.F.,(4,3,3,3,3,3,3,3,4),(22.4855718508715,22.7684575126537,
23.7583904479864,24.7483233833192,25.738256318652,26.7281892539847,27.7181221893175,
28.7080551246503,28.7687571580511),.UNSPECIFIED.);
#499=B_SPLINE_CURVE_WITH_KNOTS('',3,(#38955,#38956,#38957,#38958,#38959,
#38960,#38961,#38962,#38963,#38964,#38965,#38966,#38967,#38968,#38969,#38970,
#38971,#38972,#38973,#38974,#38975,#38976),.UNSPECIFIED.,.F.,.F.,(4,3,3,
3,3,3,3,4),(-38.0212241792183,-37.6174515426452,-36.6275186073124,-35.6375856719796,
-34.6476527366469,-33.6577198013141,-32.6677868659813,-31.7380388720387),
 .UNSPECIFIED.);
#500=B_SPLINE_CURVE_WITH_KNOTS('',3,(#38977,#38978,#38979,#38980,#38981,
#38982,#38983,#38984,#38985,#38986,#38987,#38988,#38989,#38990,#38991,#38992,
#38993,#38994,#38995,#38996,#38997,#38998),.UNSPECIFIED.,.F.,.F.,(4,3,3,
3,3,3,3,4),(28.7687571580511,29.697988059983,30.6879209953158,31.6778539306486,
32.6677868659813,33.6577198013141,34.6476527366469,35.0519424652307),
 .UNSPECIFIED.);
#501=B_SPLINE_CURVE_WITH_KNOTS('',3,(#39003,#39004,#39005,#39006,#39007,
#39008,#39009,#39010,#39011,#39012,#39013,#39014,#39015,#39016,#39017,#39018,
#39019,#39020,#39021,#39022,#39023,#39024),.UNSPECIFIED.,.F.,.F.,(4,3,3,
3,3,3,3,4),(-44.3044094863979,-43.5570491546418,-42.567116219309,-41.5771832839762,
-40.5872503486435,-39.5973174133107,-38.6073844779779,-38.0212241792183),
 .UNSPECIFIED.);
#502=B_SPLINE_CURVE_WITH_KNOTS('',3,(#39025,#39026,#39027,#39028,#39029,
#39030,#39031,#39032,#39033,#39034,#39035,#39036,#39037,#39038,#39039,#39040,
#39041,#39042,#39043,#39044,#39045,#39046),.UNSPECIFIED.,.F.,.F.,(4,3,3,
3,3,3,3,4),(35.0519424652307,35.6375856719796,36.6275186073124,37.6174515426452,
38.6073844779779,39.5973174133107,40.5872503486435,41.3351277724103),
 .UNSPECIFIED.);
#503=B_SPLINE_CURVE_WITH_KNOTS('',3,(#39051,#39052,#39053,#39054,#39055,
#39056,#39057,#39058,#39059,#39060,#39061,#39062,#39063,#39064,#39065,#39066,
#39067,#39068,#39069,#39070,#39071,#39072,#39073,#39074,#39075),
 .UNSPECIFIED.,.F.,.F.,(4,3,3,3,3,3,3,3,4),(-50.5875947935775,-50.4865797019712,
-49.4966467666384,-48.5067138313056,-47.5167808959729,-46.5268479606401,
-45.5369150253073,-44.5469820899746,-44.3044094863979),.UNSPECIFIED.);
#504=B_SPLINE_CURVE_WITH_KNOTS('',3,(#39076,#39077,#39078,#39079,#39080,
#39081,#39082,#39083,#39084,#39085,#39086,#39087,#39088,#39089,#39090,#39091,
#39092,#39093,#39094,#39095,#39096,#39097,#39098,#39099,#39100),
 .UNSPECIFIED.,.F.,.F.,(4,3,3,3,3,3,3,3,4),(41.3351277724103,41.5771832839762,
42.567116219309,43.5570491546418,44.5469820899745,45.5369150253073,46.5268479606401,
47.5167808959728,47.6183130795899),.UNSPECIFIED.);
#505=B_SPLINE_CURVE_WITH_KNOTS('',3,(#39105,#39106,#39107,#39108,#39109,
#39110,#39111,#39112,#39113,#39114,#39115,#39116,#39117,#39118,#39119,#39120,
#39121,#39122,#39123,#39124,#39125,#39126),.UNSPECIFIED.,.F.,.F.,(4,3,3,
3,3,3,3,4),(-56.8707801007571,-56.4261773139678,-55.436244378635,-54.4463114433022,
-53.4563785079695,-52.4664455726367,-51.4765126373039,-50.5875947935775),
 .UNSPECIFIED.);
#506=B_SPLINE_CURVE_WITH_KNOTS('',3,(#39127,#39128,#39129,#39130,#39131,
#39132,#39133,#39134,#39135,#39136,#39137,#39138,#39139,#39140,#39141,#39142,
#39143,#39144,#39145,#39146,#39147,#39148),.UNSPECIFIED.,.F.,.F.,(4,3,3,
3,3,3,3,4),(47.6183130795899,48.5067138313056,49.4966467666384,50.4865797019711,
51.4765126373039,52.4664455726367,53.4563785079694,53.9014983867695),
 .UNSPECIFIED.);
#507=B_SPLINE_CURVE_WITH_KNOTS('',3,(#39153,#39154,#39155,#39156,#39157,
#39158,#39159,#39160,#39161,#39162,#39163,#39164,#39165,#39166,#39167,#39168,
#39169,#39170,#39171,#39172,#39173,#39174),.UNSPECIFIED.,.F.,.F.,(4,3,3,
3,3,3,3,4),(-63.1539654079367,-62.3657749259644,-61.3758419906316,-60.3859090552988,
-59.3959761199661,-58.4060431846333,-57.4161102493005,-56.8707801007571),
 .UNSPECIFIED.);
#508=B_SPLINE_CURVE_WITH_KNOTS('',3,(#39175,#39176,#39177,#39178,#39179,
#39180,#39181,#39182,#39183,#39184,#39185,#39186,#39187,#39188,#39189,#39190,
#39191,#39192,#39193,#39194,#39195,#39196),.UNSPECIFIED.,.F.,.F.,(4,3,3,
3,3,3,3,4),(53.9014983867695,54.4463114433022,55.436244378635,56.4261773139677,
57.4161102493005,58.4060431846333,59.3959761199661,60.1846836939491),
 .UNSPECIFIED.);
#509=B_SPLINE_CURVE_WITH_KNOTS('',3,(#39201,#39202,#39203,#39204,#39205,
#39206,#39207,#39208,#39209,#39210,#39211,#39212,#39213,#39214,#39215,#39216,
#39217,#39218,#39219,#39220,#39221,#39222,#39223,#39224,#39225),
 .UNSPECIFIED.,.F.,.F.,(4,3,3,3,3,3,3,3,4),(-69.4371507151163,-69.2953054732937,
-68.305372537961,-67.3154396026282,-66.3255066672954,-65.3355737319627,
-64.3456407966299,-63.3557078612971,-63.1539654079367),.UNSPECIFIED.);
#510=B_SPLINE_CURVE_WITH_KNOTS('',3,(#39226,#39227,#39228,#39229,#39230,
#39231,#39232,#39233,#39234,#39235,#39236,#39237,#39238,#39239,#39240,#39241,
#39242,#39243,#39244,#39245,#39246,#39247,#39248,#39249,#39250),
 .UNSPECIFIED.,.F.,.F.,(4,3,3,3,3,3,3,3,4),(60.1846836939491,60.3859090552988,
61.3758419906316,62.3657749259644,63.3557078612971,64.3456407966299,65.3355737319627,
66.3255066672954,66.4678690011287),.UNSPECIFIED.);
#511=B_SPLINE_CURVE_WITH_KNOTS('',3,(#39255,#39256,#39257,#39258,#39259,
#39260,#39261,#39262,#39263,#39264,#39265,#39266,#39267,#39268,#39269,#39270,
#39271,#39272,#39273,#39274,#39275,#39276),.UNSPECIFIED.,.F.,.F.,(4,3,3,
3,3,3,3,4),(-75.7203360222959,-75.2349030852904,-74.2449701499576,-73.2550372146248,
-72.2651042792921,-71.2751713439593,-70.2852384086265,-69.4371507151163),
 .UNSPECIFIED.);
#512=B_SPLINE_CURVE_WITH_KNOTS('',3,(#39277,#39278,#39279,#39280,#39281,
#39282,#39283,#39284,#39285,#39286,#39287,#39288,#39289,#39290,#39291,#39292,
#39293,#39294,#39295,#39296,#39297,#39298),.UNSPECIFIED.,.F.,.F.,(4,3,3,
3,3,3,3,4),(66.4678690011287,67.3154396026282,68.3053725379609,69.2953054732937,
70.2852384086265,71.2751713439593,72.265104279292,72.7510543083083),
 .UNSPECIFIED.);
#513=B_SPLINE_CURVE_WITH_KNOTS('',3,(#39303,#39304,#39305,#39306,#39307,
#39308,#39309,#39310,#39311,#39312,#39313,#39314,#39315,#39316,#39317,#39318,
#39319,#39320,#39321,#39322,#39323,#39324),.UNSPECIFIED.,.F.,.F.,(4,3,3,
3,3,3,3,4),(-82.0035213294755,-81.174500697287,-80.1845677619542,-79.1946348266214,
-78.2047018912887,-77.2147689559559,-76.2248360206231,-75.7203360222959),
 .UNSPECIFIED.);
#514=B_SPLINE_CURVE_WITH_KNOTS('',3,(#39325,#39326,#39327,#39328,#39329,
#39330,#39331,#39332,#39333,#39334,#39335,#39336,#39337,#39338,#39339,#39340,
#39341,#39342,#39343,#39344,#39345,#39346),.UNSPECIFIED.,.F.,.F.,(4,3,3,
3,3,3,3,4),(72.7510543083083,73.2550372146248,74.2449701499576,75.2349030852903,
76.2248360206231,77.2147689559559,78.2047018912886,79.0342396154878),
 .UNSPECIFIED.);
#515=B_SPLINE_CURVE_WITH_KNOTS('',3,(#39351,#39352,#39353,#39354,#39355,
#39356,#39357,#39358,#39359,#39360,#39361,#39362,#39363,#39364,#39365,#39366,
#39367,#39368,#39369,#39370,#39371,#39372,#39373,#39374,#39375),
 .UNSPECIFIED.,.F.,.F.,(4,3,3,3,3,3,3,3,4),(-88.2867066366551,-88.1040312446163,
-87.1140983092836,-86.1241653739508,-85.134232438618,-84.1442995032853,
-83.1543665679525,-82.1644336326197,-82.0035213294755),.UNSPECIFIED.);
#516=B_SPLINE_CURVE_WITH_KNOTS('',3,(#39376,#39377,#39378,#39379,#39380,
#39381,#39382,#39383,#39384,#39385,#39386,#39387,#39388,#39389,#39390,#39391,
#39392,#39393,#39394,#39395,#39396,#39397,#39398,#39399,#39400),
 .UNSPECIFIED.,.F.,.F.,(4,3,3,3,3,3,3,3,4),(79.0342396154878,79.1946348266214,
80.1845677619542,81.1745006972869,82.1644336326197,83.1543665679525,84.1442995032852,
85.134232438618,85.3174249226674),.UNSPECIFIED.);
#517=B_SPLINE_CURVE_WITH_KNOTS('',3,(#39406,#39407,#39408,#39409,#39410,
#39411),.UNSPECIFIED.,.F.,.F.,(4,1,1,4),(103.672557568463,104.479815111757,
105.46974804709,106.366374179769),.UNSPECIFIED.);
#518=B_SPLINE_CURVE_WITH_KNOTS('',3,(#39414,#39415,#39416,#39417,#39418),
 .UNSPECIFIED.,.F.,.F.,(4,1,4),(103.672557568463,104.135710324563,105.125643259896),
 .UNSPECIFIED.);
#519=B_SPLINE_CURVE_WITH_KNOTS('',3,(#39423,#39424,#39425,#39426,#39427,
#39428,#39429,#39430,#39431,#39432,#39433),.UNSPECIFIED.,.F.,.F.,(4,1,1,
1,1,1,1,1,4),(97.3893722612836,97.5502845644278,98.5402174997606,99.5301504350933,
100.520083370426,101.510016305759,102.499949241092,103.489882176424,103.672557568463),
 .UNSPECIFIED.);
#520=B_SPLINE_CURVE_WITH_KNOTS('',3,(#39434,#39435,#39436,#39437,#39438,
#39439,#39440,#39441,#39442,#39443),.UNSPECIFIED.,.F.,.F.,(4,1,1,1,1,1,
1,4),(97.3893722612836,98.1961127125668,99.1860456478996,100.175978583232,
101.165911518565,102.155844453898,103.145777389231,103.672557568463),
 .UNSPECIFIED.);
#521=B_SPLINE_CURVE_WITH_KNOTS('',3,(#39448,#39449,#39450,#39451,#39452,
#39453,#39454,#39455,#39456,#39457),.UNSPECIFIED.,.F.,.F.,(4,1,1,1,1,1,
1,4),(91.106186954104,91.6106869524312,92.600619887764,93.5905528230967,
94.5804857584295,95.5704186937623,96.560351629095,97.3893722612836),
 .UNSPECIFIED.);
#522=B_SPLINE_CURVE_WITH_KNOTS('',3,(#39458,#39459,#39460,#39461,#39462,
#39463,#39464,#39465,#39466,#39467,#39468),.UNSPECIFIED.,.F.,.F.,(4,1,1,
1,1,1,1,1,4),(91.106186954104,91.2665821652374,92.2565151005702,93.246448035903,
94.2363809712357,95.2263139065685,96.2162468419013,97.206179777234,97.3893722612836),
 .UNSPECIFIED.);
#523=B_SPLINE_CURVE_WITH_KNOTS('',3,(#39473,#39474,#39475,#39476,#39477,
#39478,#39479,#39480,#39481,#39482),.UNSPECIFIED.,.F.,.F.,(4,1,1,1,1,1,
1,4),(84.8230016469244,85.6710893404346,86.6610222757674,87.6509552111001,
88.6408881464329,89.6308210817657,90.6207540170984,91.106186954104),
 .UNSPECIFIED.);
#524=B_SPLINE_CURVE_WITH_KNOTS('',3,(#39483,#39484,#39485,#39486,#39487,
#39488,#39489,#39490,#39491,#39492),.UNSPECIFIED.,.F.,.F.,(4,1,1,1,1,1,
1,4),(84.8230016469244,85.3269845532408,86.3169174885736,87.3068504239064,
88.2967833592391,89.2867162945719,90.2766492299047,91.106186954104),
 .UNSPECIFIED.);
#525=B_SPLINE_CURVE_WITH_KNOTS('',3,(#39497,#39498,#39499,#39500,#39501,
#39502,#39503,#39504,#39505,#39506,#39507),.UNSPECIFIED.,.F.,.F.,(4,1,1,
1,1,1,1,1,4),(78.5398163397448,78.7415587931052,79.731491728438,80.7214246637707,
81.7113575991035,82.7012905344363,83.6912234697691,84.6811564051018,84.8230016469244),
 .UNSPECIFIED.);
#526=B_SPLINE_CURVE_WITH_KNOTS('',3,(#39508,#39509,#39510,#39511,#39512,
#39513,#39514,#39515,#39516,#39517),.UNSPECIFIED.,.F.,.F.,(4,1,1,1,1,1,
1,4),(78.5398163397448,79.3873869412442,80.377319876577,81.3672528119098,
82.3571857472425,83.3471186825753,84.3370516179081,84.8230016469244),
 .UNSPECIFIED.);
#527=B_SPLINE_CURVE_WITH_KNOTS('',3,(#39522,#39523,#39524,#39525,#39526,
#39527,#39528,#39529,#39530,#39531),.UNSPECIFIED.,.F.,.F.,(4,1,1,1,1,1,
1,4),(72.2566310325652,72.8019611811086,73.7918941164414,74.7818270517741,
75.7717599871069,76.7616929224397,77.7516258577724,78.5398163397448),
 .UNSPECIFIED.);
#528=B_SPLINE_CURVE_WITH_KNOTS('',3,(#39532,#39533,#39534,#39535,#39536,
#39537,#39538,#39539,#39540,#39541,#39542),.UNSPECIFIED.,.F.,.F.,(4,1,1,
1,1,1,1,1,4),(72.2566310325652,72.4578563939149,73.4477893292476,74.4377222645804,
75.4276551999132,76.4175881352459,77.4075210705787,78.3974540059115,78.5398163397448),
 .UNSPECIFIED.);
#529=B_SPLINE_CURVE_WITH_KNOTS('',3,(#39547,#39548,#39549,#39550,#39551,
#39552,#39553,#39554,#39555,#39556),.UNSPECIFIED.,.F.,.F.,(4,1,1,1,1,1,
1,4),(65.9734457253856,66.862363569112,67.8522965044448,68.8422294397775,
69.8321623751103,70.8220953104431,71.8120282457758,72.2566310325652),
 .UNSPECIFIED.);
#530=B_SPLINE_CURVE_WITH_KNOTS('',3,(#39557,#39558,#39559,#39560,#39561,
#39562,#39563,#39564,#39565,#39566),.UNSPECIFIED.,.F.,.F.,(4,1,1,1,1,1,
1,4),(65.9734457253856,66.5182587819182,67.508191717251,68.4981246525838,
69.4880575879166,70.4779905232493,71.4679234585821,72.2566310325652),
 .UNSPECIFIED.);
#531=B_SPLINE_CURVE_WITH_KNOTS('',3,(#39571,#39572,#39573,#39574,#39575,
#39576,#39577,#39578,#39579,#39580,#39581),.UNSPECIFIED.,.F.,.F.,(4,1,1,
1,1,1,1,1,4),(59.690260418206,59.9328330217826,60.9227659571154,61.9126988924482,
62.9026318277809,63.8925647631137,64.8824976984465,65.8724306337792,65.9734457253856),
 .UNSPECIFIED.);
#532=B_SPLINE_CURVE_WITH_KNOTS('',3,(#39582,#39583,#39584,#39585,#39586,
#39587,#39588,#39589,#39590,#39591),.UNSPECIFIED.,.F.,.F.,(4,1,1,1,1,1,
1,4),(59.690260418206,60.5786611699216,61.5685941052544,62.5585270405872,
63.54845997592,64.5383929112527,65.5283258465855,65.9734457253856),
 .UNSPECIFIED.);
#533=B_SPLINE_CURVE_WITH_KNOTS('',3,(#39596,#39597,#39598,#39599,#39600,
#39601,#39602,#39603,#39604,#39605),.UNSPECIFIED.,.F.,.F.,(4,1,1,1,1,1,
1,4),(53.4070751110264,53.993235409786,54.9831683451188,55.9731012804516,
56.9630342157843,57.9529671511171,58.9429000864499,59.690260418206),
 .UNSPECIFIED.);
#534=B_SPLINE_CURVE_WITH_KNOTS('',3,(#39606,#39607,#39608,#39609,#39610,
#39611,#39612,#39613,#39614,#39615,#39616),.UNSPECIFIED.,.F.,.F.,(4,1,1,
1,1,1,1,1,4),(53.4070751110264,53.6491306225923,54.639063557925,55.6289964932578,
56.6189294285906,57.6088623639234,58.5987952992561,59.5887282345889,59.690260418206),
 .UNSPECIFIED.);
#535=B_SPLINE_CURVE_WITH_KNOTS('',3,(#39621,#39622,#39623,#39624,#39625,
#39626,#39627,#39628,#39629,#39630),.UNSPECIFIED.,.F.,.F.,(4,1,1,1,1,1,
1,4),(47.1238898038469,48.0536377977894,49.0435707331222,50.0335036684549,
51.0234366037877,52.0133695391205,53.0033024744532,53.4070751110264),
 .UNSPECIFIED.);
#536=B_SPLINE_CURVE_WITH_KNOTS('',3,(#39631,#39632,#39633,#39634,#39635,
#39636,#39637,#39638,#39639,#39640),.UNSPECIFIED.,.F.,.F.,(4,1,1,1,1,1,
1,4),(47.1238898038468,47.7095330105957,48.6994659459284,49.6893988812612,
50.679331816594,51.6692647519267,52.6591976872595,53.4070751110264),
 .UNSPECIFIED.);
#537=B_SPLINE_CURVE_WITH_KNOTS('',3,(#39645,#39646,#39647,#39648,#39649,
#39650,#39651,#39652,#39653,#39654,#39655),.UNSPECIFIED.,.F.,.F.,(4,1,1,
1,1,1,1,1,4),(40.8407044966673,41.12410725046,42.1140401857928,43.1039731211256,
44.0939060564583,45.0838389917911,46.0737719271239,47.0637048624566,47.1238898038469),
 .UNSPECIFIED.);
#538=B_SPLINE_CURVE_WITH_KNOTS('',3,(#39656,#39657,#39658,#39659,#39660,
#39661,#39662,#39663,#39664,#39665),.UNSPECIFIED.,.F.,.F.,(4,1,1,1,1,1,
1,4),(40.8407044966672,41.7699353985991,42.7598683339318,43.7498012692646,
44.7397342045974,45.7296671399301,46.7196000752629,47.1238898038468),
 .UNSPECIFIED.);
#539=B_SPLINE_CURVE_WITH_KNOTS('',3,(#39670,#39671,#39672,#39673,#39674,
#39675,#39676,#39677,#39678,#39679),.UNSPECIFIED.,.F.,.F.,(4,1,1,1,1,1,
1,4),(34.5575191894877,35.1845096384634,36.1744425737962,37.164375509129,
38.1543084444617,39.1442413797945,40.1341743151273,40.8407044966673),
 .UNSPECIFIED.);
#540=B_SPLINE_CURVE_WITH_KNOTS('',3,(#39680,#39681,#39682,#39683,#39684,
#39685,#39686,#39687,#39688,#39689,#39690),.UNSPECIFIED.,.F.,.F.,(4,1,1,
1,1,1,1,1,4),(34.5575191894876,34.8404048512697,35.8303377866025,36.8202707219352,
37.810203657268,38.8001365926008,39.7900695279335,40.7800024632663,40.8407044966672),
 .UNSPECIFIED.);
#541=B_SPLINE_CURVE_WITH_KNOTS('',3,(#39695,#39696,#39697,#39698,#39699,
#39700,#39701,#39702,#39703,#39704),.UNSPECIFIED.,.F.,.F.,(4,1,1,1,1,1,
1,4),(28.2743338823081,29.2449120264668,30.2348449617996,31.2247778971324,
32.2147108324651,33.2046437677979,34.1945767031307,34.5575191894877),
 .UNSPECIFIED.);
#542=B_SPLINE_CURVE_WITH_KNOTS('',3,(#39705,#39706,#39707,#39708,#39709,
#39710,#39711,#39712,#39713,#39714),.UNSPECIFIED.,.F.,.F.,(4,1,1,1,1,1,
1,4),(28.2743338823081,28.9008072392731,29.8907401746059,30.8806731099386,
31.8706060452714,32.8605389806042,33.8504719159369,34.5575191894876),
 .UNSPECIFIED.);
#543=B_SPLINE_CURVE_WITH_KNOTS('',3,(#39719,#39720,#39721,#39722,#39723,
#39724,#39725,#39726,#39727,#39728,#39729),.UNSPECIFIED.,.F.,.F.,(4,1,1,
1,1,1,1,1,4),(21.9911485751285,22.3153814791375,23.3053144144702,24.295247349803,
25.2851802851358,26.2751132204685,27.2650461558013,28.2549790911341,28.2743338823081),
 .UNSPECIFIED.);
#544=B_SPLINE_CURVE_WITH_KNOTS('',3,(#39730,#39731,#39732,#39733,#39734,
#39735,#39736,#39737,#39738,#39739),.UNSPECIFIED.,.F.,.F.,(4,1,1,1,1,1,
1,4),(21.9911485751285,22.9612096272765,23.9511425626093,24.941075497942,
25.9310084332748,26.9209413686076,27.9108743039403,28.2743338823081),
 .UNSPECIFIED.);
#545=B_SPLINE_CURVE_WITH_KNOTS('',3,(#39744,#39745,#39746,#39747,#39748,
#39749,#39750,#39751,#39752,#39753),.UNSPECIFIED.,.F.,.F.,(4,1,1,1,1,1,
1,4),(15.7079632679489,16.3757838671408,17.3657168024736,18.3556497378064,
19.3455826731391,20.3355156084719,21.3254485438047,21.9911485751285),
 .UNSPECIFIED.);
#546=B_SPLINE_CURVE_WITH_KNOTS('',3,(#39754,#39755,#39756,#39757,#39758,
#39759,#39760,#39761,#39762,#39763,#39764),.UNSPECIFIED.,.F.,.F.,(4,1,1,
1,1,1,1,1,4),(15.7079632679489,16.0316790799471,17.0216120152799,18.0115449506126,
19.0014778859454,19.9914108212782,20.981343756611,21.9712766919437,21.9911485751285),
 .UNSPECIFIED.);
#547=B_SPLINE_CURVE_WITH_KNOTS('',3,(#39767,#39768,#39769,#39770,#39771,
#39772,#39773,#39774,#39775,#39776,#39777,#39778,#39779,#39780,#39781,#39782,
#39783,#39784,#39785,#39786,#39787,#39788,#39789,#39790,#39791,#39792,#39793,
#39794,#39795,#39796,#39797,#39798,#39799,#39800,#39801,#39802,#39803,#39804,
#39805,#39806,#39807,#39808,#39809,#39810,#39811,#39812,#39813,#39814,#39815,
#39816,#39817,#39818),.UNSPECIFIED.,.F.,.F.,(4,3,3,3,3,3,3,3,3,3,3,3,3,
3,3,3,3,4),(-0.276631791712713,-0.265450615480059,-0.249264708457004,-0.237962300703026,
-0.216900919589401,-0.204366916455402,-0.175872487121073,-0.164709026212586,
-0.155425879325222,-0.139389331983085,-0.119813112264589,-0.110539977009441,
-0.100714351836302,-0.0755357638772264,-0.0587460506531512,-0.0492722354456899,
-0.0182560868482527,0.),.UNSPECIFIED.);
#548=B_SPLINE_CURVE_WITH_KNOTS('',3,(#39823,#39824,#39825,#39826,#39827,
#39828,#39829,#39830,#39831,#39832,#39833,#39834,#39835,#39836,#39837,#39838,
#39839,#39840,#39841,#39842,#39843,#39844,#39845,#39846,#39847,#39848,#39849,
#39850,#39851,#39852,#39853,#39854,#39855,#39856,#39857,#39858,#39859,#39860,
#39861,#39862,#39863,#39864,#39865,#39866,#39867,#39868,#39869,#39870,#39871,
#39872,#39873,#39874),.UNSPECIFIED.,.F.,.F.,(4,3,3,3,3,3,3,3,3,3,3,3,3,
3,3,3,3,4),(-0.275362278356883,-0.261744724725805,-0.238870913782049,-0.228431829105,
-0.208394802250592,-0.19788610598297,-0.168242095210859,-0.148132070239196,
-0.139871540977981,-0.124344332175051,-0.106149246467418,-0.0967155779587869,
-0.0875515981565891,-0.0656636986174418,-0.0485611810495529,-0.0406387966505317,
-0.0143836439341371,0.),.UNSPECIFIED.);
#549=B_SPLINE_CURVE_WITH_KNOTS('',3,(#40263,#40264,#40265,#40266,#40267,
#40268,#40269,#40270,#40271,#40272,#40273,#40274,#40275,#40276,#40277,#40278,
#40279,#40280,#40281),.UNSPECIFIED.,.F.,.F.,(4,3,3,3,3,3,4),(85.3174249226674,
86.1241653739508,87.1140983092835,88.1040312446163,89.0939641799491,90.0838971152818,
90.9805232479604),.UNSPECIFIED.);
#550=B_SPLINE_CURVE_WITH_KNOTS('',3,(#40283,#40284,#40285,#40286,#40287,
#40288,#40289,#40290,#40291,#40292,#40293,#40294,#40295,#40296,#40297,#40298,
#40299,#40300,#40301,#40302,#40303,#40304,#40305,#40306,#40307,#40308,#40309,
#40310,#40311,#40312,#40313,#40314,#40315,#40316,#40317,#40318,#40319,#40320,
#40321,#40322,#40323,#40324,#40325,#40326,#40327,#40328,#40329,#40330,#40331,
#40332,#40333,#40334),.UNSPECIFIED.,.F.,.F.,(4,3,3,3,3,3,3,3,3,3,3,3,3,
3,3,3,3,4),(-0.276631791712722,-0.265450615480067,-0.249264709520642,-0.237962301509632,
-0.216900855800476,-0.204366904493779,-0.175872475394542,-0.164708998571383,
-0.15542586941425,-0.139389331983089,-0.119813107263836,-0.110539960157763,
-0.100714348698858,-0.0755357615241436,-0.0587460364870724,-0.0492722247833334,
-0.0182560727479066,0.),.UNSPECIFIED.);
#551=B_SPLINE_CURVE_WITH_KNOTS('',3,(#40335,#40336,#40337,#40338,#40339),
 .UNSPECIFIED.,.F.,.F.,(4,1,4),(14.1451200119358,15.0417461446143,15.7079632679489),
 .UNSPECIFIED.);
#552=B_SPLINE_CURVE_WITH_KNOTS('',3,(#40342,#40343,#40344,#40345,#40346,
#40347,#40348,#40349,#40350,#40351,#40352,#40353,#40354,#40355,#40356,#40357,
#40358,#40359,#40360,#40361,#40362,#40363,#40364,#40365,#40366,#40367,#40368,
#40369,#40370,#40371,#40372,#40373,#40374,#40375,#40376,#40377,#40378,#40379,
#40380,#40381,#40382,#40383,#40384,#40385,#40386,#40387,#40388,#40389,#40390,
#40391,#40392,#40393),.UNSPECIFIED.,.F.,.F.,(4,3,3,3,3,3,3,3,3,3,3,3,3,
3,3,3,3,4),(-0.275362278356887,-0.261744724725805,-0.238870910786292,-0.228431821713149,
-0.208394774728337,-0.197886061305117,-0.168242048891388,-0.148131926718763,
-0.139871336754713,-0.124344332175047,-0.106149407076155,-0.0967158838367153,
-0.0875520936665209,-0.0656640702498907,-0.0485622287413132,-0.0406402635470369,
-0.0143850804576057,0.),.UNSPECIFIED.);
#553=B_SPLINE_CURVE_WITH_KNOTS('',3,(#40396,#40397,#40398,#40399),
 .UNSPECIFIED.,.F.,.F.,(4,4),(15.3858509318081,15.7079632679489),
 .UNSPECIFIED.);
#554=B_SPLINE_CURVE_WITH_KNOTS('',3,(#40788,#40789,#40790,#40791,#40792,
#40793,#40794,#40795,#40796,#40797,#40798,#40799,#40800,#40801,#40802,#40803),
 .UNSPECIFIED.,.F.,.F.,(4,3,3,3,3,4),(-93.0536959212802,-92.0637629859474,
-91.0738300506146,-90.0838971152819,-89.0939641799491,-88.2867066366551),
 .UNSPECIFIED.);
#892=SHAPE_REPRESENTATION_RELATIONSHIP('SRR','None',#53737,#908);
#908=ADVANCED_BREP_SHAPE_REPRESENTATION('',(#940),#53647);
#924=STYLED_ITEM('',(#53965),#940);
#940=MANIFOLD_SOLID_BREP('ISO_4762_M3x8_A2',#23316);
#1085=CYLINDRICAL_SURFACE('',#24796,0.14635);
#1086=CYLINDRICAL_SURFACE('',#24800,0.14635);
#1087=CYLINDRICAL_SURFACE('',#24801,0.14635);
#1088=CYLINDRICAL_SURFACE('',#24802,0.14635);
#1089=CYLINDRICAL_SURFACE('',#24803,0.14635);
#1090=CYLINDRICAL_SURFACE('',#24804,0.14635);
#1091=CYLINDRICAL_SURFACE('',#24805,0.14635);
#1092=CYLINDRICAL_SURFACE('',#24806,0.14635);
#1093=CYLINDRICAL_SURFACE('',#24807,0.14635);
#1094=CYLINDRICAL_SURFACE('',#24808,0.14635);
#1095=CYLINDRICAL_SURFACE('',#24809,0.14635);
#1096=CYLINDRICAL_SURFACE('',#24810,0.14635);
#1097=CYLINDRICAL_SURFACE('',#24811,0.14635);
#1098=CYLINDRICAL_SURFACE('',#24812,0.14635);
#1099=CYLINDRICAL_SURFACE('',#24813,0.117775);
#1100=CYLINDRICAL_SURFACE('',#24815,0.117775);
#1101=CYLINDRICAL_SURFACE('',#24816,0.117775);
#1102=CYLINDRICAL_SURFACE('',#24817,0.117775);
#1103=CYLINDRICAL_SURFACE('',#24818,0.117775);
#1104=CYLINDRICAL_SURFACE('',#24819,0.117775);
#1105=CYLINDRICAL_SURFACE('',#24820,0.117775);
#1106=CYLINDRICAL_SURFACE('',#24821,0.117775);
#1107=CYLINDRICAL_SURFACE('',#24822,0.117775);
#1108=CYLINDRICAL_SURFACE('',#24823,0.117775);
#1109=CYLINDRICAL_SURFACE('',#24824,0.117775);
#1110=CYLINDRICAL_SURFACE('',#24825,0.117775);
#1111=CYLINDRICAL_SURFACE('',#24826,0.117775);
#1112=CYLINDRICAL_SURFACE('',#24827,0.117775);
#1113=CYLINDRICAL_SURFACE('',#24828,0.117775);
#1114=CYLINDRICAL_SURFACE('',#24834,0.117775);
#1115=CYLINDRICAL_SURFACE('',#24976,0.275);
#1116=CYLINDRICAL_SURFACE('',#25032,0.14635);
#1439=FACE_BOUND('',#4636,.T.);
#1440=FACE_BOUND('',#4642,.T.);
#1441=FACE_BOUND('',#4644,.T.);
#1876=PLANE('',#24829);
#1877=PLANE('',#24832);
#1878=PLANE('',#24835);
#1879=PLANE('',#24837);
#1880=PLANE('',#24838);
#1881=PLANE('',#24839);
#1882=PLANE('',#24841);
#1883=PLANE('',#24842);
#1884=PLANE('',#24843);
#1885=PLANE('',#24845);
#1886=PLANE('',#24846);
#1887=PLANE('',#24847);
#1888=PLANE('',#24849);
#1889=PLANE('',#24850);
#1890=PLANE('',#24851);
#1891=PLANE('',#24853);
#1892=PLANE('',#24854);
#1893=PLANE('',#24855);
#1894=PLANE('',#24857);
#1895=PLANE('',#24858);
#1896=PLANE('',#24859);
#1897=PLANE('',#24861);
#1898=PLANE('',#24862);
#1899=PLANE('',#24863);
#1900=PLANE('',#24865);
#1901=PLANE('',#24866);
#1902=PLANE('',#24867);
#1903=PLANE('',#24869);
#1904=PLANE('',#24870);
#1905=PLANE('',#24871);
#1906=PLANE('',#24873);
#1907=PLANE('',#24874);
#1908=PLANE('',#24875);
#1909=PLANE('',#24877);
#1910=PLANE('',#24878);
#1911=PLANE('',#24879);
#1912=PLANE('',#24881);
#1913=PLANE('',#24882);
#1914=PLANE('',#24883);
#1915=PLANE('',#24885);
#1916=PLANE('',#24886);
#1917=PLANE('',#24887);
#1918=PLANE('',#24889);
#1919=PLANE('',#24890);
#1920=PLANE('',#24891);
#1921=PLANE('',#24893);
#1922=PLANE('',#24894);
#1923=PLANE('',#24895);
#1924=PLANE('',#24897);
#1925=PLANE('',#24898);
#1926=PLANE('',#24899);
#1927=PLANE('',#24901);
#1928=PLANE('',#24902);
#1929=PLANE('',#24903);
#1930=PLANE('',#24906);
#1931=PLANE('',#24907);
#1932=PLANE('',#24908);
#1933=PLANE('',#24910);
#1934=PLANE('',#24911);
#1935=PLANE('',#24912);
#1936=PLANE('',#24914);
#1937=PLANE('',#24915);
#1938=PLANE('',#24916);
#1939=PLANE('',#24918);
#1940=PLANE('',#24919);
#1941=PLANE('',#24920);
#1942=PLANE('',#24922);
#1943=PLANE('',#24923);
#1944=PLANE('',#24924);
#1945=PLANE('',#24926);
#1946=PLANE('',#24927);
#1947=PLANE('',#24928);
#1948=PLANE('',#24930);
#1949=PLANE('',#24931);
#1950=PLANE('',#24932);
#1951=PLANE('',#24934);
#1952=PLANE('',#24935);
#1953=PLANE('',#24936);
#1954=PLANE('',#24938);
#1955=PLANE('',#24939);
#1956=PLANE('',#24940);
#1957=PLANE('',#24942);
#1958=PLANE('',#24943);
#1959=PLANE('',#24944);
#1960=PLANE('',#24946);
#1961=PLANE('',#24947);
#1962=PLANE('',#24948);
#1963=PLANE('',#24950);
#1964=PLANE('',#24951);
#1965=PLANE('',#24952);
#1966=PLANE('',#24954);
#1967=PLANE('',#24955);
#1968=PLANE('',#24956);
#1969=PLANE('',#24958);
#1970=PLANE('',#24959);
#1971=PLANE('',#24960);
#1972=PLANE('',#24962);
#1973=PLANE('',#24963);
#1974=PLANE('',#24964);
#1975=PLANE('',#24966);
#1976=PLANE('',#24967);
#1977=PLANE('',#24968);
#1978=PLANE('',#24970);
#1979=PLANE('',#24971);
#1980=PLANE('',#24972);
#1981=PLANE('',#24974);
#1982=PLANE('',#24975);
#1983=PLANE('',#25015);
#1984=PLANE('',#25016);
#1985=PLANE('',#25017);
#1986=PLANE('',#25022);
#1987=PLANE('',#25023);
#1988=PLANE('',#25024);
#1989=PLANE('',#25025);
#1990=PLANE('',#25026);
#1991=PLANE('',#25027);
#1992=PLANE('',#25028);
#1993=PLANE('',#25029);
#1994=PLANE('',#25036);
#1995=PLANE('',#25037);
#2994=FACE_OUTER_BOUND('',#4484,.T.);
#2995=FACE_OUTER_BOUND('',#4485,.T.);
#2996=FACE_OUTER_BOUND('',#4486,.T.);
#2997=FACE_OUTER_BOUND('',#4487,.T.);
#2998=FACE_OUTER_BOUND('',#4488,.T.);
#2999=FACE_OUTER_BOUND('',#4489,.T.);
#3000=FACE_OUTER_BOUND('',#4490,.T.);
#3001=FACE_OUTER_BOUND('',#4491,.T.);
#3002=FACE_OUTER_BOUND('',#4492,.T.);
#3003=FACE_OUTER_BOUND('',#4493,.T.);
#3004=FACE_OUTER_BOUND('',#4494,.T.);
#3005=FACE_OUTER_BOUND('',#4495,.T.);
#3006=FACE_OUTER_BOUND('',#4496,.T.);
#3007=FACE_OUTER_BOUND('',#4497,.T.);
#3008=FACE_OUTER_BOUND('',#4498,.T.);
#3009=FACE_OUTER_BOUND('',#4499,.T.);
#3010=FACE_OUTER_BOUND('',#4500,.T.);
#3011=FACE_OUTER_BOUND('',#4501,.T.);
#3012=FACE_OUTER_BOUND('',#4502,.T.);
#3013=FACE_OUTER_BOUND('',#4503,.T.);
#3014=FACE_OUTER_BOUND('',#4504,.T.);
#3015=FACE_OUTER_BOUND('',#4505,.T.);
#3016=FACE_OUTER_BOUND('',#4506,.T.);
#3017=FACE_OUTER_BOUND('',#4507,.T.);
#3018=FACE_OUTER_BOUND('',#4508,.T.);
#3019=FACE_OUTER_BOUND('',#4509,.T.);
#3020=FACE_OUTER_BOUND('',#4510,.T.);
#3021=FACE_OUTER_BOUND('',#4511,.T.);
#3022=FACE_OUTER_BOUND('',#4512,.T.);
#3023=FACE_OUTER_BOUND('',#4513,.T.);
#3024=FACE_OUTER_BOUND('',#4514,.T.);
#3025=FACE_OUTER_BOUND('',#4515,.T.);
#3026=FACE_OUTER_BOUND('',#4516,.T.);
#3027=FACE_OUTER_BOUND('',#4517,.T.);
#3028=FACE_OUTER_BOUND('',#4518,.T.);
#3029=FACE_OUTER_BOUND('',#4519,.T.);
#3030=FACE_OUTER_BOUND('',#4520,.T.);
#3031=FACE_OUTER_BOUND('',#4521,.T.);
#3032=FACE_OUTER_BOUND('',#4522,.T.);
#3033=FACE_OUTER_BOUND('',#4523,.T.);
#3034=FACE_OUTER_BOUND('',#4524,.T.);
#3035=FACE_OUTER_BOUND('',#4525,.T.);
#3036=FACE_OUTER_BOUND('',#4526,.T.);
#3037=FACE_OUTER_BOUND('',#4527,.T.);
#3038=FACE_OUTER_BOUND('',#4528,.T.);
#3039=FACE_OUTER_BOUND('',#4529,.T.);
#3040=FACE_OUTER_BOUND('',#4530,.T.);
#3041=FACE_OUTER_BOUND('',#4531,.T.);
#3042=FACE_OUTER_BOUND('',#4532,.T.);
#3043=FACE_OUTER_BOUND('',#4533,.T.);
#3044=FACE_OUTER_BOUND('',#4534,.T.);
#3045=FACE_OUTER_BOUND('',#4535,.T.);
#3046=FACE_OUTER_BOUND('',#4536,.T.);
#3047=FACE_OUTER_BOUND('',#4537,.T.);
#3048=FACE_OUTER_BOUND('',#4538,.T.);
#3049=FACE_OUTER_BOUND('',#4539,.T.);
#3050=FACE_OUTER_BOUND('',#4540,.T.);
#3051=FACE_OUTER_BOUND('',#4541,.T.);
#3052=FACE_OUTER_BOUND('',#4542,.T.);
#3053=FACE_OUTER_BOUND('',#4543,.T.);
#3054=FACE_OUTER_BOUND('',#4544,.T.);
#3055=FACE_OUTER_BOUND('',#4545,.T.);
#3056=FACE_OUTER_BOUND('',#4546,.T.);
#3057=FACE_OUTER_BOUND('',#4547,.T.);
#3058=FACE_OUTER_BOUND('',#4548,.T.);
#3059=FACE_OUTER_BOUND('',#4549,.T.);
#3060=FACE_OUTER_BOUND('',#4550,.T.);
#3061=FACE_OUTER_BOUND('',#4551,.T.);
#3062=FACE_OUTER_BOUND('',#4552,.T.);
#3063=FACE_OUTER_BOUND('',#4553,.T.);
#3064=FACE_OUTER_BOUND('',#4554,.T.);
#3065=FACE_OUTER_BOUND('',#4555,.T.);
#3066=FACE_OUTER_BOUND('',#4556,.T.);
#3067=FACE_OUTER_BOUND('',#4557,.T.);
#3068=FACE_OUTER_BOUND('',#4558,.T.);
#3069=FACE_OUTER_BOUND('',#4559,.T.);
#3070=FACE_OUTER_BOUND('',#4560,.T.);
#3071=FACE_OUTER_BOUND('',#4561,.T.);
#3072=FACE_OUTER_BOUND('',#4562,.T.);
#3073=FACE_OUTER_BOUND('',#4563,.T.);
#3074=FACE_OUTER_BOUND('',#4564,.T.);
#3075=FACE_OUTER_BOUND('',#4565,.T.);
#3076=FACE_OUTER_BOUND('',#4566,.T.);
#3077=FACE_OUTER_BOUND('',#4567,.T.);
#3078=FACE_OUTER_BOUND('',#4568,.T.);
#3079=FACE_OUTER_BOUND('',#4569,.T.);
#3080=FACE_OUTER_BOUND('',#4570,.T.);
#3081=FACE_OUTER_BOUND('',#4571,.T.);
#3082=FACE_OUTER_BOUND('',#4572,.T.);
#3083=FACE_OUTER_BOUND('',#4573,.T.);
#3084=FACE_OUTER_BOUND('',#4574,.T.);
#3085=FACE_OUTER_BOUND('',#4575,.T.);
#3086=FACE_OUTER_BOUND('',#4576,.T.);
#3087=FACE_OUTER_BOUND('',#4577,.T.);
#3088=FACE_OUTER_BOUND('',#4578,.T.);
#3089=FACE_OUTER_BOUND('',#4579,.T.);
#3090=FACE_OUTER_BOUND('',#4580,.T.);
#3091=FACE_OUTER_BOUND('',#4581,.T.);
#3092=FACE_OUTER_BOUND('',#4582,.T.);
#3093=FACE_OUTER_BOUND('',#4583,.T.);
#3094=FACE_OUTER_BOUND('',#4584,.T.);
#3095=FACE_OUTER_BOUND('',#4585,.T.);
#3096=FACE_OUTER_BOUND('',#4586,.T.);
#3097=FACE_OUTER_BOUND('',#4587,.T.);
#3098=FACE_OUTER_BOUND('',#4588,.T.);
#3099=FACE_OUTER_BOUND('',#4589,.T.);
#3100=FACE_OUTER_BOUND('',#4590,.T.);
#3101=FACE_OUTER_BOUND('',#4591,.T.);
#3102=FACE_OUTER_BOUND('',#4592,.T.);
#3103=FACE_OUTER_BOUND('',#4593,.T.);
#3104=FACE_OUTER_BOUND('',#4594,.T.);
#3105=FACE_OUTER_BOUND('',#4595,.T.);
#3106=FACE_OUTER_BOUND('',#4596,.T.);
#3107=FACE_OUTER_BOUND('',#4597,.T.);
#3108=FACE_OUTER_BOUND('',#4598,.T.);
#3109=FACE_OUTER_BOUND('',#4599,.T.);
#3110=FACE_OUTER_BOUND('',#4600,.T.);
#3111=FACE_OUTER_BOUND('',#4601,.T.);
#3112=FACE_OUTER_BOUND('',#4602,.T.);
#3113=FACE_OUTER_BOUND('',#4603,.T.);
#3114=FACE_OUTER_BOUND('',#4604,.T.);
#3115=FACE_OUTER_BOUND('',#4605,.T.);
#3116=FACE_OUTER_BOUND('',#4606,.T.);
#3117=FACE_OUTER_BOUND('',#4607,.T.);
#3118=FACE_OUTER_BOUND('',#4608,.T.);
#3119=FACE_OUTER_BOUND('',#4609,.T.);
#3120=FACE_OUTER_BOUND('',#4610,.T.);
#3121=FACE_OUTER_BOUND('',#4611,.T.);
#3122=FACE_OUTER_BOUND('',#4612,.T.);
#3123=FACE_OUTER_BOUND('',#4613,.T.);
#3124=FACE_OUTER_BOUND('',#4614,.T.);
#3125=FACE_OUTER_BOUND('',#4615,.T.);
#3126=FACE_OUTER_BOUND('',#4616,.T.);
#3127=FACE_OUTER_BOUND('',#4617,.T.);
#3128=FACE_OUTER_BOUND('',#4618,.T.);
#3129=FACE_OUTER_BOUND('',#4619,.T.);
#3130=FACE_OUTER_BOUND('',#4620,.T.);
#3131=FACE_OUTER_BOUND('',#4621,.T.);
#3132=FACE_OUTER_BOUND('',#4622,.T.);
#3133=FACE_OUTER_BOUND('',#4623,.T.);
#3134=FACE_OUTER_BOUND('',#4624,.T.);
#3135=FACE_OUTER_BOUND('',#4625,.T.);
#3136=FACE_OUTER_BOUND('',#4626,.T.);
#3137=FACE_OUTER_BOUND('',#4627,.T.);
#3138=FACE_OUTER_BOUND('',#4628,.T.);
#3139=FACE_OUTER_BOUND('',#4629,.T.);
#3140=FACE_OUTER_BOUND('',#4630,.T.);
#3141=FACE_OUTER_BOUND('',#4631,.T.);
#3142=FACE_OUTER_BOUND('',#4632,.T.);
#3143=FACE_OUTER_BOUND('',#4633,.T.);
#3144=FACE_OUTER_BOUND('',#4634,.T.);
#3145=FACE_OUTER_BOUND('',#4635,.T.);
#3146=FACE_OUTER_BOUND('',#4637,.T.);
#3147=FACE_OUTER_BOUND('',#4638,.T.);
#3148=FACE_OUTER_BOUND('',#4639,.T.);
#3149=FACE_OUTER_BOUND('',#4640,.T.);
#3150=FACE_OUTER_BOUND('',#4641,.T.);
#3151=FACE_OUTER_BOUND('',#4643,.T.);
#4484=EDGE_LOOP('',(#18461,#18462,#18463,#18464,#18465,#18466,#18467,#18468));
#4485=EDGE_LOOP('',(#18469,#18470,#18471,#18472));
#4486=EDGE_LOOP('',(#18473,#18474,#18475,#18476));
#4487=EDGE_LOOP('',(#18477,#18478,#18479,#18480));
#4488=EDGE_LOOP('',(#18481,#18482,#18483,#18484));
#4489=EDGE_LOOP('',(#18485,#18486,#18487,#18488));
#4490=EDGE_LOOP('',(#18489,#18490,#18491,#18492));
#4491=EDGE_LOOP('',(#18493,#18494,#18495,#18496));
#4492=EDGE_LOOP('',(#18497,#18498,#18499,#18500));
#4493=EDGE_LOOP('',(#18501,#18502,#18503,#18504));
#4494=EDGE_LOOP('',(#18505,#18506,#18507,#18508));
#4495=EDGE_LOOP('',(#18509,#18510,#18511,#18512));
#4496=EDGE_LOOP('',(#18513,#18514,#18515,#18516));
#4497=EDGE_LOOP('',(#18517,#18518,#18519,#18520));
#4498=EDGE_LOOP('',(#18521,#18522,#18523,#18524));
#4499=EDGE_LOOP('',(#18525,#18526,#18527,#18528));
#4500=EDGE_LOOP('',(#18529,#18530,#18531,#18532));
#4501=EDGE_LOOP('',(#18533,#18534,#18535,#18536));
#4502=EDGE_LOOP('',(#18537,#18538,#18539,#18540));
#4503=EDGE_LOOP('',(#18541,#18542,#18543,#18544));
#4504=EDGE_LOOP('',(#18545,#18546,#18547,#18548));
#4505=EDGE_LOOP('',(#18549,#18550,#18551,#18552));
#4506=EDGE_LOOP('',(#18553,#18554,#18555,#18556));
#4507=EDGE_LOOP('',(#18557,#18558,#18559,#18560));
#4508=EDGE_LOOP('',(#18561,#18562,#18563,#18564));
#4509=EDGE_LOOP('',(#18565,#18566,#18567,#18568));
#4510=EDGE_LOOP('',(#18569,#18570,#18571,#18572));
#4511=EDGE_LOOP('',(#18573,#18574,#18575,#18576));
#4512=EDGE_LOOP('',(#18577,#18578,#18579,#18580));
#4513=EDGE_LOOP('',(#18581,#18582,#18583,#18584,#18585));
#4514=EDGE_LOOP('',(#18586,#18587,#18588,#18589,#18590,#18591,#18592,#18593,
#18594,#18595,#18596,#18597,#18598,#18599,#18600,#18601,#18602,#18603,#18604,
#18605,#18606,#18607,#18608,#18609,#18610,#18611,#18612,#18613,#18614,#18615,
#18616,#18617,#18618));
#4515=EDGE_LOOP('',(#18619,#18620,#18621,#18622,#18623));
#4516=EDGE_LOOP('',(#18624,#18625,#18626,#18627));
#4517=EDGE_LOOP('',(#18628,#18629,#18630,#18631,#18632,#18633,#18634,#18635,
#18636,#18637,#18638,#18639,#18640,#18641,#18642,#18643,#18644,#18645,#18646,
#18647,#18648,#18649,#18650,#18651,#18652,#18653,#18654,#18655,#18656,#18657,
#18658,#18659,#18660));
#4518=EDGE_LOOP('',(#18661,#18662,#18663));
#4519=EDGE_LOOP('',(#18664,#18665,#18666,#18667));
#4520=EDGE_LOOP('',(#18668,#18669,#18670,#18671));
#4521=EDGE_LOOP('',(#18672,#18673,#18674));
#4522=EDGE_LOOP('',(#18675,#18676,#18677,#18678));
#4523=EDGE_LOOP('',(#18679,#18680,#18681,#18682));
#4524=EDGE_LOOP('',(#18683,#18684,#18685));
#4525=EDGE_LOOP('',(#18686,#18687,#18688,#18689));
#4526=EDGE_LOOP('',(#18690,#18691,#18692,#18693));
#4527=EDGE_LOOP('',(#18694,#18695,#18696));
#4528=EDGE_LOOP('',(#18697,#18698,#18699,#18700));
#4529=EDGE_LOOP('',(#18701,#18702,#18703,#18704));
#4530=EDGE_LOOP('',(#18705,#18706,#18707));
#4531=EDGE_LOOP('',(#18708,#18709,#18710,#18711));
#4532=EDGE_LOOP('',(#18712,#18713,#18714,#18715));
#4533=EDGE_LOOP('',(#18716,#18717,#18718));
#4534=EDGE_LOOP('',(#18719,#18720,#18721,#18722));
#4535=EDGE_LOOP('',(#18723,#18724,#18725,#18726));
#4536=EDGE_LOOP('',(#18727,#18728,#18729));
#4537=EDGE_LOOP('',(#18730,#18731,#18732,#18733));
#4538=EDGE_LOOP('',(#18734,#18735,#18736,#18737));
#4539=EDGE_LOOP('',(#18738,#18739,#18740));
#4540=EDGE_LOOP('',(#18741,#18742,#18743,#18744));
#4541=EDGE_LOOP('',(#18745,#18746,#18747,#18748));
#4542=EDGE_LOOP('',(#18749,#18750,#18751));
#4543=EDGE_LOOP('',(#18752,#18753,#18754,#18755));
#4544=EDGE_LOOP('',(#18756,#18757,#18758,#18759));
#4545=EDGE_LOOP('',(#18760,#18761,#18762));
#4546=EDGE_LOOP('',(#18763,#18764,#18765,#18766));
#4547=EDGE_LOOP('',(#18767,#18768,#18769,#18770));
#4548=EDGE_LOOP('',(#18771,#18772,#18773));
#4549=EDGE_LOOP('',(#18774,#18775,#18776,#18777));
#4550=EDGE_LOOP('',(#18778,#18779,#18780,#18781));
#4551=EDGE_LOOP('',(#18782,#18783,#18784));
#4552=EDGE_LOOP('',(#18785,#18786,#18787,#18788));
#4553=EDGE_LOOP('',(#18789,#18790,#18791,#18792));
#4554=EDGE_LOOP('',(#18793,#18794,#18795));
#4555=EDGE_LOOP('',(#18796,#18797,#18798,#18799));
#4556=EDGE_LOOP('',(#18800,#18801,#18802,#18803));
#4557=EDGE_LOOP('',(#18804,#18805,#18806));
#4558=EDGE_LOOP('',(#18807,#18808,#18809,#18810));
#4559=EDGE_LOOP('',(#18811,#18812,#18813,#18814));
#4560=EDGE_LOOP('',(#18815,#18816,#18817));
#4561=EDGE_LOOP('',(#18818,#18819,#18820,#18821));
#4562=EDGE_LOOP('',(#18822,#18823,#18824,#18825));
#4563=EDGE_LOOP('',(#18826,#18827,#18828));
#4564=EDGE_LOOP('',(#18829,#18830,#18831,#18832));
#4565=EDGE_LOOP('',(#18833,#18834,#18835,#18836));
#4566=EDGE_LOOP('',(#18837,#18838,#18839));
#4567=EDGE_LOOP('',(#18840,#18841,#18842,#18843));
#4568=EDGE_LOOP('',(#18844,#18845,#18846,#18847));
#4569=EDGE_LOOP('',(#18848,#18849,#18850,#18851));
#4570=EDGE_LOOP('',(#18852,#18853,#18854,#18855));
#4571=EDGE_LOOP('',(#18856,#18857,#18858,#18859));
#4572=EDGE_LOOP('',(#18860,#18861,#18862));
#4573=EDGE_LOOP('',(#18863,#18864,#18865,#18866));
#4574=EDGE_LOOP('',(#18867,#18868,#18869,#18870));
#4575=EDGE_LOOP('',(#18871,#18872,#18873));
#4576=EDGE_LOOP('',(#18874,#18875,#18876,#18877));
#4577=EDGE_LOOP('',(#18878,#18879,#18880,#18881));
#4578=EDGE_LOOP('',(#18882,#18883,#18884));
#4579=EDGE_LOOP('',(#18885,#18886,#18887,#18888));
#4580=EDGE_LOOP('',(#18889,#18890,#18891,#18892));
#4581=EDGE_LOOP('',(#18893,#18894,#18895));
#4582=EDGE_LOOP('',(#18896,#18897,#18898,#18899));
#4583=EDGE_LOOP('',(#18900,#18901,#18902,#18903));
#4584=EDGE_LOOP('',(#18904,#18905,#18906));
#4585=EDGE_LOOP('',(#18907,#18908,#18909,#18910));
#4586=EDGE_LOOP('',(#18911,#18912,#18913,#18914));
#4587=EDGE_LOOP('',(#18915,#18916,#18917));
#4588=EDGE_LOOP('',(#18918,#18919,#18920,#18921));
#4589=EDGE_LOOP('',(#18922,#18923,#18924,#18925));
#4590=EDGE_LOOP('',(#18926,#18927,#18928));
#4591=EDGE_LOOP('',(#18929,#18930,#18931,#18932));
#4592=EDGE_LOOP('',(#18933,#18934,#18935,#18936));
#4593=EDGE_LOOP('',(#18937,#18938,#18939));
#4594=EDGE_LOOP('',(#18940,#18941,#18942,#18943));
#4595=EDGE_LOOP('',(#18944,#18945,#18946,#18947));
#4596=EDGE_LOOP('',(#18948,#18949,#18950));
#4597=EDGE_LOOP('',(#18951,#18952,#18953,#18954));
#4598=EDGE_LOOP('',(#18955,#18956,#18957,#18958));
#4599=EDGE_LOOP('',(#18959,#18960,#18961));
#4600=EDGE_LOOP('',(#18962,#18963,#18964,#18965));
#4601=EDGE_LOOP('',(#18966,#18967,#18968,#18969));
#4602=EDGE_LOOP('',(#18970,#18971,#18972));
#4603=EDGE_LOOP('',(#18973,#18974,#18975,#18976));
#4604=EDGE_LOOP('',(#18977,#18978,#18979,#18980));
#4605=EDGE_LOOP('',(#18981,#18982,#18983));
#4606=EDGE_LOOP('',(#18984,#18985,#18986,#18987));
#4607=EDGE_LOOP('',(#18988,#18989,#18990,#18991));
#4608=EDGE_LOOP('',(#18992,#18993,#18994));
#4609=EDGE_LOOP('',(#18995,#18996,#18997,#18998));
#4610=EDGE_LOOP('',(#18999,#19000,#19001,#19002));
#4611=EDGE_LOOP('',(#19003,#19004,#19005));
#4612=EDGE_LOOP('',(#19006,#19007,#19008,#19009));
#4613=EDGE_LOOP('',(#19010,#19011,#19012,#19013));
#4614=EDGE_LOOP('',(#19014,#19015,#19016));
#4615=EDGE_LOOP('',(#19017,#19018,#19019,#19020));
#4616=EDGE_LOOP('',(#19021,#19022,#19023,#19024));
#4617=EDGE_LOOP('',(#19025,#19026,#19027));
#4618=EDGE_LOOP('',(#19028,#19029,#19030,#19031));
#4619=EDGE_LOOP('',(#19032,#19033,#19034,#19035));
#4620=EDGE_LOOP('',(#19036,#19037,#19038));
#4621=EDGE_LOOP('',(#19039,#19040,#19041,#19042));
#4622=EDGE_LOOP('',(#19043,#19044,#19045,#19046));
#4623=EDGE_LOOP('',(#19047,#19048,#19049,#19050,#19051,#19052,#19053,#19054,
#19055,#19056,#19057,#19058,#19059,#19060,#19061,#19062,#19063,#19064,#19065,
#19066,#19067,#19068,#19069,#19070,#19071,#19072,#19073,#19074,#19075,#19076,
#19077,#19078,#19079,#19080,#19081,#19082,#19083,#19084,#19085,#19086,#19087,
#19088,#19089,#19090,#19091,#19092,#19093,#19094,#19095,#19096,#19097,#19098,
#19099,#19100,#19101,#19102,#19103,#19104,#19105,#19106,#19107,#19108,#19109,
#19110,#19111,#19112,#19113,#19114,#19115,#19116,#19117,#19118,#19119,#19120,
#19121,#19122,#19123,#19124,#19125,#19126,#19127,#19128,#19129,#19130,#19131,
#19132,#19133,#19134,#19135,#19136,#19137,#19138,#19139,#19140,#19141,#19142,
#19143,#19144,#19145,#19146,#19147,#19148,#19149,#19150,#19151,#19152,#19153,
#19154,#19155,#19156,#19157,#19158,#19159,#19160,#19161,#19162,#19163,#19164,
#19165,#19166,#19167,#19168,#19169,#19170,#19171,#19172,#19173,#19174,#19175,
#19176,#19177,#19178,#19179,#19180,#19181,#19182,#19183,#19184,#19185,#19186,
#19187,#19188,#19189,#19190,#19191,#19192,#19193,#19194));
#4624=EDGE_LOOP('',(#19195,#19196,#19197,#19198));
#4625=EDGE_LOOP('',(#19199,#19200,#19201,#19202));
#4626=EDGE_LOOP('',(#19203,#19204,#19205));
#4627=EDGE_LOOP('',(#19206,#19207,#19208,#19209,#19210,#19211,#19212,#19213,
#19214,#19215,#19216,#19217,#19218,#19219,#19220,#19221,#19222,#19223,#19224,
#19225,#19226,#19227,#19228,#19229,#19230,#19231,#19232,#19233,#19234,#19235,
#19236,#19237,#19238,#19239,#19240,#19241,#19242,#19243,#19244,#19245,#19246,
#19247,#19248,#19249,#19250,#19251,#19252,#19253,#19254,#19255,#19256,#19257,
#19258,#19259,#19260,#19261,#19262,#19263,#19264,#19265,#19266,#19267,#19268,
#19269,#19270,#19271,#19272,#19273,#19274,#19275,#19276,#19277,#19278,#19279,
#19280,#19281,#19282,#19283,#19284,#19285,#19286,#19287,#19288,#19289,#19290,
#19291,#19292,#19293,#19294,#19295,#19296,#19297,#19298,#19299,#19300,#19301,
#19302,#19303,#19304,#19305,#19306,#19307,#19308,#19309,#19310,#19311,#19312,
#19313,#19314,#19315,#19316));
#4628=EDGE_LOOP('',(#19317,#19318,#19319));
#4629=EDGE_LOOP('',(#19320,#19321,#19322,#19323));
#4630=EDGE_LOOP('',(#19324,#19325,#19326,#19327));
#4631=EDGE_LOOP('',(#19328,#19329,#19330,#19331));
#4632=EDGE_LOOP('',(#19332,#19333,#19334,#19335));
#4633=EDGE_LOOP('',(#19336,#19337,#19338,#19339));
#4634=EDGE_LOOP('',(#19340,#19341,#19342,#19343));
#4635=EDGE_LOOP('',(#19344,#19345,#19346,#19347,#19348,#19349));
#4636=EDGE_LOOP('',(#19350));
#4637=EDGE_LOOP('',(#19351));
#4638=EDGE_LOOP('',(#19352,#19353,#19354,#19355));
#4639=EDGE_LOOP('',(#19356,#19357,#19358,#19359));
#4640=EDGE_LOOP('',(#19360,#19361,#19362,#19363,#19364,#19365));
#4641=EDGE_LOOP('',(#19366));
#4642=EDGE_LOOP('',(#19367));
#4643=EDGE_LOOP('',(#19368));
#4644=EDGE_LOOP('',(#19369,#19370,#19371,#19372,#19373,#19374));
#5594=CIRCLE('',#24797,0.14635);
#5595=CIRCLE('',#24798,0.14635);
#5596=CIRCLE('',#24799,0.14635);
#5597=CIRCLE('',#24814,0.117775);
#5598=CIRCLE('',#24830,0.14635);
#5599=CIRCLE('',#24831,0.14635);
#5600=CIRCLE('',#24833,0.117775);
#5601=CIRCLE('',#24836,0.275);
#5602=CIRCLE('',#24840,0.275);
#5603=CIRCLE('',#24844,0.275);
#5604=CIRCLE('',#24848,0.275);
#5605=CIRCLE('',#24852,0.275);
#5606=CIRCLE('',#24856,0.275);
#5607=CIRCLE('',#24860,0.275);
#5608=CIRCLE('',#24864,0.275);
#5609=CIRCLE('',#24868,0.275);
#5610=CIRCLE('',#24872,0.275);
#5611=CIRCLE('',#24876,0.275);
#5612=CIRCLE('',#24880,0.275);
#5613=CIRCLE('',#24884,0.275);
#5614=CIRCLE('',#24888,0.275);
#5615=CIRCLE('',#24892,0.275);
#5616=CIRCLE('',#24896,0.275);
#5617=CIRCLE('',#24900,0.275);
#5618=CIRCLE('',#24904,0.275);
#5619=CIRCLE('',#24905,0.275);
#5620=CIRCLE('',#24909,0.275);
#5621=CIRCLE('',#24913,0.275);
#5622=CIRCLE('',#24917,0.275);
#5623=CIRCLE('',#24921,0.275);
#5624=CIRCLE('',#24925,0.275);
#5625=CIRCLE('',#24929,0.275);
#5626=CIRCLE('',#24933,0.275);
#5627=CIRCLE('',#24937,0.275);
#5628=CIRCLE('',#24941,0.275);
#5629=CIRCLE('',#24945,0.275);
#5630=CIRCLE('',#24949,0.275);
#5631=CIRCLE('',#24953,0.275);
#5632=CIRCLE('',#24957,0.275);
#5633=CIRCLE('',#24961,0.275);
#5634=CIRCLE('',#24965,0.275);
#5635=CIRCLE('',#24969,0.275);
#5636=CIRCLE('',#24973,0.275);
#5637=CIRCLE('',#24977,0.275);
#5638=CIRCLE('',#24978,0.275);
#5639=CIRCLE('',#24979,0.275);
#5640=CIRCLE('',#24980,0.275);
#5641=CIRCLE('',#24981,0.275);
#5642=CIRCLE('',#24982,0.275);
#5643=CIRCLE('',#24983,0.275);
#5644=CIRCLE('',#24984,0.275);
#5645=CIRCLE('',#24985,0.275);
#5646=CIRCLE('',#24986,0.275);
#5647=CIRCLE('',#24987,0.275);
#5648=CIRCLE('',#24988,0.275);
#5649=CIRCLE('',#24989,0.275);
#5650=CIRCLE('',#24990,0.275);
#5651=CIRCLE('',#24991,0.275);
#5652=CIRCLE('',#24992,0.275);
#5653=CIRCLE('',#24993,0.275);
#5654=CIRCLE('',#24994,0.275);
#5655=CIRCLE('',#24995,0.275);
#5656=CIRCLE('',#24996,0.275);
#5657=CIRCLE('',#24997,0.275);
#5658=CIRCLE('',#24998,0.275);
#5659=CIRCLE('',#24999,0.275);
#5660=CIRCLE('',#25000,0.275);
#5661=CIRCLE('',#25001,0.275);
#5662=CIRCLE('',#25002,0.275);
#5663=CIRCLE('',#25003,0.275);
#5664=CIRCLE('',#25004,0.275);
#5665=CIRCLE('',#25005,0.275);
#5666=CIRCLE('',#25006,0.275);
#5667=CIRCLE('',#25007,0.275);
#5668=CIRCLE('',#25008,0.275);
#5669=CIRCLE('',#25009,0.275);
#5670=CIRCLE('',#25010,0.275);
#5671=CIRCLE('',#25011,0.275);
#5672=CIRCLE('',#25012,0.275);
#5673=CIRCLE('',#25013,0.275);
#5674=CIRCLE('',#25014,0.275);
#5675=CIRCLE('',#25019,0.26);
#5676=CIRCLE('',#25021,0.113891921086774);
#5677=CIRCLE('',#25030,0.114);
#5678=CIRCLE('',#25033,0.14635);
#5679=CIRCLE('',#25035,0.16);
#6902=LINE('',#38709,#8747);
#6903=LINE('',#38730,#8748);
#6904=LINE('',#38750,#8749);
#6905=LINE('',#38804,#8750);
#6906=LINE('',#38852,#8751);
#6907=LINE('',#38900,#8752);
#6908=LINE('',#38954,#8753);
#6909=LINE('',#39002,#8754);
#6910=LINE('',#39050,#8755);
#6911=LINE('',#39104,#8756);
#6912=LINE('',#39152,#8757);
#6913=LINE('',#39200,#8758);
#6914=LINE('',#39254,#8759);
#6915=LINE('',#39302,#8760);
#6916=LINE('',#39350,#8761);
#6917=LINE('',#39404,#8762);
#6918=LINE('',#39422,#8763);
#6919=LINE('',#39447,#8764);
#6920=LINE('',#39472,#8765);
#6921=LINE('',#39496,#8766);
#6922=LINE('',#39521,#8767);
#6923=LINE('',#39546,#8768);
#6924=LINE('',#39570,#8769);
#6925=LINE('',#39595,#8770);
#6926=LINE('',#39620,#8771);
#6927=LINE('',#39644,#8772);
#6928=LINE('',#39669,#8773);
#6929=LINE('',#39694,#8774);
#6930=LINE('',#39718,#8775);
#6931=LINE('',#39743,#8776);
#6932=LINE('',#40809,#8777);
#6933=LINE('',#40810,#8778);
#6934=LINE('',#40813,#8779);
#6935=LINE('',#40815,#8780);
#6936=LINE('',#40821,#8781);
#6937=LINE('',#40830,#8782);
#6938=LINE('',#40831,#8783);
#6939=LINE('',#40834,#8784);
#6940=LINE('',#40836,#8785);
#6941=LINE('',#40842,#8786);
#6942=LINE('',#40851,#8787);
#6943=LINE('',#40852,#8788);
#6944=LINE('',#40855,#8789);
#6945=LINE('',#40857,#8790);
#6946=LINE('',#40863,#8791);
#6947=LINE('',#40872,#8792);
#6948=LINE('',#40873,#8793);
#6949=LINE('',#40876,#8794);
#6950=LINE('',#40878,#8795);
#6951=LINE('',#40884,#8796);
#6952=LINE('',#40893,#8797);
#6953=LINE('',#40894,#8798);
#6954=LINE('',#40897,#8799);
#6955=LINE('',#40899,#8800);
#6956=LINE('',#40905,#8801);
#6957=LINE('',#40914,#8802);
#6958=LINE('',#40915,#8803);
#6959=LINE('',#40918,#8804);
#6960=LINE('',#40920,#8805);
#6961=LINE('',#40926,#8806);
#6962=LINE('',#40935,#8807);
#6963=LINE('',#40936,#8808);
#6964=LINE('',#40939,#8809);
#6965=LINE('',#40941,#8810);
#6966=LINE('',#40947,#8811);
#6967=LINE('',#40956,#8812);
#6968=LINE('',#40957,#8813);
#6969=LINE('',#40960,#8814);
#6970=LINE('',#40962,#8815);
#6971=LINE('',#40968,#8816);
#6972=LINE('',#40977,#8817);
#6973=LINE('',#40978,#8818);
#6974=LINE('',#40981,#8819);
#6975=LINE('',#40983,#8820);
#6976=LINE('',#40989,#8821);
#6977=LINE('',#40998,#8822);
#6978=LINE('',#40999,#8823);
#6979=LINE('',#41002,#8824);
#6980=LINE('',#41004,#8825);
#6981=LINE('',#41010,#8826);
#6982=LINE('',#41019,#8827);
#6983=LINE('',#41020,#8828);
#6984=LINE('',#41023,#8829);
#6985=LINE('',#41025,#8830);
#6986=LINE('',#41031,#8831);
#6987=LINE('',#41040,#8832);
#6988=LINE('',#41041,#8833);
#6989=LINE('',#41044,#8834);
#6990=LINE('',#41046,#8835);
#6991=LINE('',#41052,#8836);
#6992=LINE('',#41061,#8837);
#6993=LINE('',#41062,#8838);
#6994=LINE('',#41065,#8839);
#6995=LINE('',#41067,#8840);
#6996=LINE('',#41073,#8841);
#6997=LINE('',#41082,#8842);
#6998=LINE('',#41083,#8843);
#6999=LINE('',#41086,#8844);
#7000=LINE('',#41088,#8845);
#7001=LINE('',#41094,#8846);
#7002=LINE('',#41103,#8847);
#7003=LINE('',#41104,#8848);
#7004=LINE('',#41107,#8849);
#7005=LINE('',#41109,#8850);
#7006=LINE('',#41115,#8851);
#7007=LINE('',#41124,#8852);
#7008=LINE('',#41125,#8853);
#7009=LINE('',#41128,#8854);
#7010=LINE('',#41130,#8855);
#7011=LINE('',#41136,#8856);
#7012=LINE('',#41145,#8857);
#7013=LINE('',#41146,#8858);
#7014=LINE('',#41149,#8859);
#7015=LINE('',#41151,#8860);
#7016=LINE('',#41157,#8861);
#7017=LINE('',#41166,#8862);
#7018=LINE('',#41168,#8863);
#7019=LINE('',#41172,#8864);
#7020=LINE('',#41174,#8865);
#7021=LINE('',#41180,#8866);
#7022=LINE('',#41189,#8867);
#7023=LINE('',#41190,#8868);
#7024=LINE('',#41193,#8869);
#7025=LINE('',#41195,#8870);
#7026=LINE('',#41201,#8871);
#7027=LINE('',#41210,#8872);
#7028=LINE('',#41211,#8873);
#7029=LINE('',#41214,#8874);
#7030=LINE('',#41216,#8875);
#7031=LINE('',#41222,#8876);
#7032=LINE('',#41231,#8877);
#7033=LINE('',#41232,#8878);
#7034=LINE('',#41235,#8879);
#7035=LINE('',#41237,#8880);
#7036=LINE('',#41243,#8881);
#7037=LINE('',#41252,#8882);
#7038=LINE('',#41253,#8883);
#7039=LINE('',#41256,#8884);
#7040=LINE('',#41258,#8885);
#7041=LINE('',#41264,#8886);
#7042=LINE('',#41273,#8887);
#7043=LINE('',#41274,#8888);
#7044=LINE('',#41277,#8889);
#7045=LINE('',#41279,#8890);
#7046=LINE('',#41285,#8891);
#7047=LINE('',#41294,#8892);
#7048=LINE('',#41295,#8893);
#7049=LINE('',#41298,#8894);
#7050=LINE('',#41300,#8895);
#7051=LINE('',#41306,#8896);
#7052=LINE('',#41315,#8897);
#7053=LINE('',#41316,#8898);
#7054=LINE('',#41319,#8899);
#7055=LINE('',#41321,#8900);
#7056=LINE('',#41327,#8901);
#7057=LINE('',#41336,#8902);
#7058=LINE('',#41337,#8903);
#7059=LINE('',#41340,#8904);
#7060=LINE('',#41342,#8905);
#7061=LINE('',#41348,#8906);
#7062=LINE('',#41357,#8907);
#7063=LINE('',#41358,#8908);
#7064=LINE('',#41361,#8909);
#7065=LINE('',#41363,#8910);
#7066=LINE('',#41369,#8911);
#7067=LINE('',#41378,#8912);
#7068=LINE('',#41379,#8913);
#7069=LINE('',#41382,#8914);
#7070=LINE('',#41384,#8915);
#7071=LINE('',#41390,#8916);
#7072=LINE('',#41399,#8917);
#7073=LINE('',#41400,#8918);
#7074=LINE('',#41403,#8919);
#7075=LINE('',#41405,#8920);
#7076=LINE('',#41411,#8921);
#7077=LINE('',#41420,#8922);
#7078=LINE('',#41421,#8923);
#7079=LINE('',#41424,#8924);
#7080=LINE('',#41426,#8925);
#7081=LINE('',#41432,#8926);
#7082=LINE('',#41441,#8927);
#7083=LINE('',#41442,#8928);
#7084=LINE('',#41445,#8929);
#7085=LINE('',#41447,#8930);
#7086=LINE('',#41453,#8931);
#7087=LINE('',#41462,#8932);
#7088=LINE('',#41463,#8933);
#7089=LINE('',#41466,#8934);
#7090=LINE('',#41468,#8935);
#7091=LINE('',#41474,#8936);
#7092=LINE('',#41483,#8937);
#7093=LINE('',#41484,#8938);
#7094=LINE('',#41487,#8939);
#7095=LINE('',#41489,#8940);
#7096=LINE('',#41495,#8941);
#7097=LINE('',#41504,#8942);
#7098=LINE('',#41505,#8943);
#7099=LINE('',#41508,#8944);
#7100=LINE('',#41510,#8945);
#7101=LINE('',#41516,#8946);
#7102=LINE('',#41525,#8947);
#7103=LINE('',#41526,#8948);
#7104=LINE('',#41529,#8949);
#7105=LINE('',#41531,#8950);
#7106=LINE('',#41537,#8951);
#7107=LINE('',#41560,#8952);
#7108=LINE('',#41582,#8953);
#7109=LINE('',#41586,#8954);
#7110=LINE('',#41590,#8955);
#7111=LINE('',#41592,#8956);
#7112=LINE('',#41600,#8957);
#7113=LINE('',#41605,#8958);
#7114=LINE('',#41609,#8959);
#7115=LINE('',#41614,#8960);
#7116=LINE('',#41616,#8961);
#7117=LINE('',#41618,#8962);
#7118=LINE('',#41619,#8963);
#7119=LINE('',#41622,#8964);
#7120=LINE('',#41624,#8965);
#7121=LINE('',#41625,#8966);
#7122=LINE('',#41628,#8967);
#7123=LINE('',#41630,#8968);
#7124=LINE('',#41631,#8969);
#7125=LINE('',#41634,#8970);
#7126=LINE('',#41636,#8971);
#7127=LINE('',#41637,#8972);
#7128=LINE('',#41640,#8973);
#7129=LINE('',#41642,#8974);
#7130=LINE('',#41643,#8975);
#7131=LINE('',#41645,#8976);
#7132=LINE('',#41646,#8977);
#7133=LINE('',#41652,#8978);
#7134=LINE('',#41658,#8979);
#8747=VECTOR('',#29306,0.15);
#8748=VECTOR('',#29309,0.15);
#8749=VECTOR('',#29316,0.15);
#8750=VECTOR('',#29319,0.15);
#8751=VECTOR('',#29322,0.15);
#8752=VECTOR('',#29325,0.15);
#8753=VECTOR('',#29328,0.15);
#8754=VECTOR('',#29331,0.15);
#8755=VECTOR('',#29334,0.15);
#8756=VECTOR('',#29337,0.15);
#8757=VECTOR('',#29340,0.15);
#8758=VECTOR('',#29343,0.15);
#8759=VECTOR('',#29346,0.15);
#8760=VECTOR('',#29349,0.15);
#8761=VECTOR('',#29352,0.15);
#8762=VECTOR('',#29355,0.117775);
#8763=VECTOR('',#29360,0.117775);
#8764=VECTOR('',#29363,0.117775);
#8765=VECTOR('',#29366,0.117775);
#8766=VECTOR('',#29369,0.117775);
#8767=VECTOR('',#29372,0.117775);
#8768=VECTOR('',#29375,0.117775);
#8769=VECTOR('',#29378,0.117775);
#8770=VECTOR('',#29381,0.117775);
#8771=VECTOR('',#29384,0.117775);
#8772=VECTOR('',#29387,0.117775);
#8773=VECTOR('',#29390,0.117775);
#8774=VECTOR('',#29393,0.117775);
#8775=VECTOR('',#29396,0.117775);
#8776=VECTOR('',#29399,0.117775);
#8777=VECTOR('',#29416,1.);
#8778=VECTOR('',#29417,1.);
#8779=VECTOR('',#29420,1.);
#8780=VECTOR('',#29421,1.);
#8781=VECTOR('',#29424,1.);
#8782=VECTOR('',#29429,1.);
#8783=VECTOR('',#29430,1.);
#8784=VECTOR('',#29433,1.);
#8785=VECTOR('',#29434,1.);
#8786=VECTOR('',#29437,1.);
#8787=VECTOR('',#29442,1.);
#8788=VECTOR('',#29443,1.);
#8789=VECTOR('',#29446,1.);
#8790=VECTOR('',#29447,1.);
#8791=VECTOR('',#29450,1.);
#8792=VECTOR('',#29455,1.);
#8793=VECTOR('',#29456,1.);
#8794=VECTOR('',#29459,1.);
#8795=VECTOR('',#29460,1.);
#8796=VECTOR('',#29463,1.);
#8797=VECTOR('',#29468,1.);
#8798=VECTOR('',#29469,1.);
#8799=VECTOR('',#29472,1.);
#8800=VECTOR('',#29473,1.);
#8801=VECTOR('',#29476,1.);
#8802=VECTOR('',#29481,1.);
#8803=VECTOR('',#29482,1.);
#8804=VECTOR('',#29485,1.);
#8805=VECTOR('',#29486,1.);
#8806=VECTOR('',#29489,1.);
#8807=VECTOR('',#29494,1.);
#8808=VECTOR('',#29495,1.);
#8809=VECTOR('',#29498,1.);
#8810=VECTOR('',#29499,1.);
#8811=VECTOR('',#29502,1.);
#8812=VECTOR('',#29507,1.);
#8813=VECTOR('',#29508,1.);
#8814=VECTOR('',#29511,1.);
#8815=VECTOR('',#29512,1.);
#8816=VECTOR('',#29515,1.);
#8817=VECTOR('',#29520,1.);
#8818=VECTOR('',#29521,1.);
#8819=VECTOR('',#29524,1.);
#8820=VECTOR('',#29525,1.);
#8821=VECTOR('',#29528,1.);
#8822=VECTOR('',#29533,1.);
#8823=VECTOR('',#29534,1.);
#8824=VECTOR('',#29537,1.);
#8825=VECTOR('',#29538,1.);
#8826=VECTOR('',#29541,1.);
#8827=VECTOR('',#29546,1.);
#8828=VECTOR('',#29547,1.);
#8829=VECTOR('',#29550,1.);
#8830=VECTOR('',#29551,1.);
#8831=VECTOR('',#29554,1.);
#8832=VECTOR('',#29559,1.);
#8833=VECTOR('',#29560,1.);
#8834=VECTOR('',#29563,1.);
#8835=VECTOR('',#29564,1.);
#8836=VECTOR('',#29567,1.);
#8837=VECTOR('',#29572,1.);
#8838=VECTOR('',#29573,1.);
#8839=VECTOR('',#29576,1.);
#8840=VECTOR('',#29577,1.);
#8841=VECTOR('',#29580,1.);
#8842=VECTOR('',#29585,1.);
#8843=VECTOR('',#29586,1.);
#8844=VECTOR('',#29589,1.);
#8845=VECTOR('',#29590,1.);
#8846=VECTOR('',#29593,1.);
#8847=VECTOR('',#29598,1.);
#8848=VECTOR('',#29599,1.);
#8849=VECTOR('',#29602,1.);
#8850=VECTOR('',#29603,1.);
#8851=VECTOR('',#29606,1.);
#8852=VECTOR('',#29611,1.);
#8853=VECTOR('',#29612,1.);
#8854=VECTOR('',#29615,1.);
#8855=VECTOR('',#29616,1.);
#8856=VECTOR('',#29619,1.);
#8857=VECTOR('',#29624,1.);
#8858=VECTOR('',#29625,1.);
#8859=VECTOR('',#29628,1.);
#8860=VECTOR('',#29629,1.);
#8861=VECTOR('',#29632,1.);
#8862=VECTOR('',#29637,1.);
#8863=VECTOR('',#29638,1.);
#8864=VECTOR('',#29643,1.);
#8865=VECTOR('',#29644,1.);
#8866=VECTOR('',#29647,1.);
#8867=VECTOR('',#29652,1.);
#8868=VECTOR('',#29653,1.);
#8869=VECTOR('',#29656,1.);
#8870=VECTOR('',#29657,1.);
#8871=VECTOR('',#29660,1.);
#8872=VECTOR('',#29665,1.);
#8873=VECTOR('',#29666,1.);
#8874=VECTOR('',#29669,1.);
#8875=VECTOR('',#29670,1.);
#8876=VECTOR('',#29673,1.);
#8877=VECTOR('',#29678,1.);
#8878=VECTOR('',#29679,1.);
#8879=VECTOR('',#29682,1.);
#8880=VECTOR('',#29683,1.);
#8881=VECTOR('',#29686,1.);
#8882=VECTOR('',#29691,1.);
#8883=VECTOR('',#29692,1.);
#8884=VECTOR('',#29695,1.);
#8885=VECTOR('',#29696,1.);
#8886=VECTOR('',#29699,1.);
#8887=VECTOR('',#29704,1.);
#8888=VECTOR('',#29705,1.);
#8889=VECTOR('',#29708,1.);
#8890=VECTOR('',#29709,1.);
#8891=VECTOR('',#29712,1.);
#8892=VECTOR('',#29717,1.);
#8893=VECTOR('',#29718,1.);
#8894=VECTOR('',#29721,1.);
#8895=VECTOR('',#29722,1.);
#8896=VECTOR('',#29725,1.);
#8897=VECTOR('',#29730,1.);
#8898=VECTOR('',#29731,1.);
#8899=VECTOR('',#29734,1.);
#8900=VECTOR('',#29735,1.);
#8901=VECTOR('',#29738,1.);
#8902=VECTOR('',#29743,1.);
#8903=VECTOR('',#29744,1.);
#8904=VECTOR('',#29747,1.);
#8905=VECTOR('',#29748,1.);
#8906=VECTOR('',#29751,1.);
#8907=VECTOR('',#29756,1.);
#8908=VECTOR('',#29757,1.);
#8909=VECTOR('',#29760,1.);
#8910=VECTOR('',#29761,1.);
#8911=VECTOR('',#29764,1.);
#8912=VECTOR('',#29769,1.);
#8913=VECTOR('',#29770,1.);
#8914=VECTOR('',#29773,1.);
#8915=VECTOR('',#29774,1.);
#8916=VECTOR('',#29777,1.);
#8917=VECTOR('',#29782,1.);
#8918=VECTOR('',#29783,1.);
#8919=VECTOR('',#29786,1.);
#8920=VECTOR('',#29787,1.);
#8921=VECTOR('',#29790,1.);
#8922=VECTOR('',#29795,1.);
#8923=VECTOR('',#29796,1.);
#8924=VECTOR('',#29799,1.);
#8925=VECTOR('',#29800,1.);
#8926=VECTOR('',#29803,1.);
#8927=VECTOR('',#29808,1.);
#8928=VECTOR('',#29809,1.);
#8929=VECTOR('',#29812,1.);
#8930=VECTOR('',#29813,1.);
#8931=VECTOR('',#29816,1.);
#8932=VECTOR('',#29821,1.);
#8933=VECTOR('',#29822,1.);
#8934=VECTOR('',#29825,1.);
#8935=VECTOR('',#29826,1.);
#8936=VECTOR('',#29829,1.);
#8937=VECTOR('',#29834,1.);
#8938=VECTOR('',#29835,1.);
#8939=VECTOR('',#29838,1.);
#8940=VECTOR('',#29839,1.);
#8941=VECTOR('',#29842,1.);
#8942=VECTOR('',#29847,1.);
#8943=VECTOR('',#29848,1.);
#8944=VECTOR('',#29851,1.);
#8945=VECTOR('',#29852,1.);
#8946=VECTOR('',#29855,1.);
#8947=VECTOR('',#29860,1.);
#8948=VECTOR('',#29861,1.);
#8949=VECTOR('',#29864,1.);
#8950=VECTOR('',#29865,1.);
#8951=VECTOR('',#29868,1.);
#8952=VECTOR('',#29905,0.275);
#8953=VECTOR('',#29944,1.);
#8954=VECTOR('',#29947,1.);
#8955=VECTOR('',#29952,1.);
#8956=VECTOR('',#29953,1.);
#8957=VECTOR('',#29956,1.);
#8958=VECTOR('',#29963,0.2675);
#8959=VECTOR('',#29966,0.0577350269189626);
#8960=VECTOR('',#29971,1.);
#8961=VECTOR('',#29972,1.);
#8962=VECTOR('',#29973,1.);
#8963=VECTOR('',#29974,1.);
#8964=VECTOR('',#29977,1.);
#8965=VECTOR('',#29978,1.);
#8966=VECTOR('',#29979,1.);
#8967=VECTOR('',#29982,1.);
#8968=VECTOR('',#29983,1.);
#8969=VECTOR('',#29984,1.);
#8970=VECTOR('',#29987,1.);
#8971=VECTOR('',#29988,1.);
#8972=VECTOR('',#29989,1.);
#8973=VECTOR('',#29992,1.);
#8974=VECTOR('',#29993,1.);
#8975=VECTOR('',#29994,1.);
#8976=VECTOR('',#29997,1.);
#8977=VECTOR('',#29998,1.);
#8978=VECTOR('',#30007,0.132);
#8979=VECTOR('',#30016,0.155);
#10607=VERTEX_POINT('',#38707);
#10608=VERTEX_POINT('',#38708);
#10609=VERTEX_POINT('',#38710);
#10610=VERTEX_POINT('',#38727);
#10611=VERTEX_POINT('',#38729);
#10612=VERTEX_POINT('',#38732);
#10613=VERTEX_POINT('',#38748);
#10614=VERTEX_POINT('',#38749);
#10615=VERTEX_POINT('',#38802);
#10616=VERTEX_POINT('',#38803);
#10617=VERTEX_POINT('',#38850);
#10618=VERTEX_POINT('',#38851);
#10619=VERTEX_POINT('',#38898);
#10620=VERTEX_POINT('',#38899);
#10621=VERTEX_POINT('',#38952);
#10622=VERTEX_POINT('',#38953);
#10623=VERTEX_POINT('',#39000);
#10624=VERTEX_POINT('',#39001);
#10625=VERTEX_POINT('',#39048);
#10626=VERTEX_POINT('',#39049);
#10627=VERTEX_POINT('',#39102);
#10628=VERTEX_POINT('',#39103);
#10629=VERTEX_POINT('',#39150);
#10630=VERTEX_POINT('',#39151);
#10631=VERTEX_POINT('',#39198);
#10632=VERTEX_POINT('',#39199);
#10633=VERTEX_POINT('',#39252);
#10634=VERTEX_POINT('',#39253);
#10635=VERTEX_POINT('',#39300);
#10636=VERTEX_POINT('',#39301);
#10637=VERTEX_POINT('',#39348);
#10638=VERTEX_POINT('',#39349);
#10639=VERTEX_POINT('',#39402);
#10640=VERTEX_POINT('',#39403);
#10641=VERTEX_POINT('',#39405);
#10642=VERTEX_POINT('',#39412);
#10643=VERTEX_POINT('',#39420);
#10644=VERTEX_POINT('',#39421);
#10645=VERTEX_POINT('',#39445);
#10646=VERTEX_POINT('',#39446);
#10647=VERTEX_POINT('',#39470);
#10648=VERTEX_POINT('',#39471);
#10649=VERTEX_POINT('',#39494);
#10650=VERTEX_POINT('',#39495);
#10651=VERTEX_POINT('',#39519);
#10652=VERTEX_POINT('',#39520);
#10653=VERTEX_POINT('',#39544);
#10654=VERTEX_POINT('',#39545);
#10655=VERTEX_POINT('',#39568);
#10656=VERTEX_POINT('',#39569);
#10657=VERTEX_POINT('',#39593);
#10658=VERTEX_POINT('',#39594);
#10659=VERTEX_POINT('',#39618);
#10660=VERTEX_POINT('',#39619);
#10661=VERTEX_POINT('',#39642);
#10662=VERTEX_POINT('',#39643);
#10663=VERTEX_POINT('',#39667);
#10664=VERTEX_POINT('',#39668);
#10665=VERTEX_POINT('',#39692);
#10666=VERTEX_POINT('',#39693);
#10667=VERTEX_POINT('',#39716);
#10668=VERTEX_POINT('',#39717);
#10669=VERTEX_POINT('',#39741);
#10670=VERTEX_POINT('',#39742);
#10671=VERTEX_POINT('',#39766);
#10672=VERTEX_POINT('',#39819);
#10673=VERTEX_POINT('',#39821);
#10674=VERTEX_POINT('',#40282);
#10675=VERTEX_POINT('',#40341);
#10676=VERTEX_POINT('',#40805);
#10677=VERTEX_POINT('',#40806);
#10678=VERTEX_POINT('',#40808);
#10679=VERTEX_POINT('',#40812);
#10680=VERTEX_POINT('',#40814);
#10681=VERTEX_POINT('',#40820);
#10682=VERTEX_POINT('',#40826);
#10683=VERTEX_POINT('',#40827);
#10684=VERTEX_POINT('',#40829);
#10685=VERTEX_POINT('',#40833);
#10686=VERTEX_POINT('',#40835);
#10687=VERTEX_POINT('',#40841);
#10688=VERTEX_POINT('',#40847);
#10689=VERTEX_POINT('',#40848);
#10690=VERTEX_POINT('',#40850);
#10691=VERTEX_POINT('',#40854);
#10692=VERTEX_POINT('',#40856);
#10693=VERTEX_POINT('',#40862);
#10694=VERTEX_POINT('',#40868);
#10695=VERTEX_POINT('',#40869);
#10696=VERTEX_POINT('',#40871);
#10697=VERTEX_POINT('',#40875);
#10698=VERTEX_POINT('',#40877);
#10699=VERTEX_POINT('',#40883);
#10700=VERTEX_POINT('',#40889);
#10701=VERTEX_POINT('',#40890);
#10702=VERTEX_POINT('',#40892);
#10703=VERTEX_POINT('',#40896);
#10704=VERTEX_POINT('',#40898);
#10705=VERTEX_POINT('',#40904);
#10706=VERTEX_POINT('',#40910);
#10707=VERTEX_POINT('',#40911);
#10708=VERTEX_POINT('',#40913);
#10709=VERTEX_POINT('',#40917);
#10710=VERTEX_POINT('',#40919);
#10711=VERTEX_POINT('',#40925);
#10712=VERTEX_POINT('',#40931);
#10713=VERTEX_POINT('',#40932);
#10714=VERTEX_POINT('',#40934);
#10715=VERTEX_POINT('',#40938);
#10716=VERTEX_POINT('',#40940);
#10717=VERTEX_POINT('',#40946);
#10718=VERTEX_POINT('',#40952);
#10719=VERTEX_POINT('',#40953);
#10720=VERTEX_POINT('',#40955);
#10721=VERTEX_POINT('',#40959);
#10722=VERTEX_POINT('',#40961);
#10723=VERTEX_POINT('',#40967);
#10724=VERTEX_POINT('',#40973);
#10725=VERTEX_POINT('',#40974);
#10726=VERTEX_POINT('',#40976);
#10727=VERTEX_POINT('',#40980);
#10728=VERTEX_POINT('',#40982);
#10729=VERTEX_POINT('',#40988);
#10730=VERTEX_POINT('',#40994);
#10731=VERTEX_POINT('',#40995);
#10732=VERTEX_POINT('',#40997);
#10733=VERTEX_POINT('',#41001);
#10734=VERTEX_POINT('',#41003);
#10735=VERTEX_POINT('',#41009);
#10736=VERTEX_POINT('',#41015);
#10737=VERTEX_POINT('',#41016);
#10738=VERTEX_POINT('',#41018);
#10739=VERTEX_POINT('',#41022);
#10740=VERTEX_POINT('',#41024);
#10741=VERTEX_POINT('',#41030);
#10742=VERTEX_POINT('',#41036);
#10743=VERTEX_POINT('',#41037);
#10744=VERTEX_POINT('',#41039);
#10745=VERTEX_POINT('',#41043);
#10746=VERTEX_POINT('',#41045);
#10747=VERTEX_POINT('',#41051);
#10748=VERTEX_POINT('',#41057);
#10749=VERTEX_POINT('',#41058);
#10750=VERTEX_POINT('',#41060);
#10751=VERTEX_POINT('',#41064);
#10752=VERTEX_POINT('',#41066);
#10753=VERTEX_POINT('',#41072);
#10754=VERTEX_POINT('',#41078);
#10755=VERTEX_POINT('',#41079);
#10756=VERTEX_POINT('',#41081);
#10757=VERTEX_POINT('',#41085);
#10758=VERTEX_POINT('',#41087);
#10759=VERTEX_POINT('',#41093);
#10760=VERTEX_POINT('',#41099);
#10761=VERTEX_POINT('',#41100);
#10762=VERTEX_POINT('',#41102);
#10763=VERTEX_POINT('',#41106);
#10764=VERTEX_POINT('',#41108);
#10765=VERTEX_POINT('',#41114);
#10766=VERTEX_POINT('',#41120);
#10767=VERTEX_POINT('',#41121);
#10768=VERTEX_POINT('',#41123);
#10769=VERTEX_POINT('',#41127);
#10770=VERTEX_POINT('',#41129);
#10771=VERTEX_POINT('',#41135);
#10772=VERTEX_POINT('',#41141);
#10773=VERTEX_POINT('',#41142);
#10774=VERTEX_POINT('',#41144);
#10775=VERTEX_POINT('',#41148);
#10776=VERTEX_POINT('',#41150);
#10777=VERTEX_POINT('',#41156);
#10778=VERTEX_POINT('',#41162);
#10779=VERTEX_POINT('',#41163);
#10780=VERTEX_POINT('',#41165);
#10781=VERTEX_POINT('',#41167);
#10782=VERTEX_POINT('',#41171);
#10783=VERTEX_POINT('',#41173);
#10784=VERTEX_POINT('',#41179);
#10785=VERTEX_POINT('',#41185);
#10786=VERTEX_POINT('',#41186);
#10787=VERTEX_POINT('',#41188);
#10788=VERTEX_POINT('',#41192);
#10789=VERTEX_POINT('',#41194);
#10790=VERTEX_POINT('',#41200);
#10791=VERTEX_POINT('',#41206);
#10792=VERTEX_POINT('',#41207);
#10793=VERTEX_POINT('',#41209);
#10794=VERTEX_POINT('',#41213);
#10795=VERTEX_POINT('',#41215);
#10796=VERTEX_POINT('',#41221);
#10797=VERTEX_POINT('',#41227);
#10798=VERTEX_POINT('',#41228);
#10799=VERTEX_POINT('',#41230);
#10800=VERTEX_POINT('',#41234);
#10801=VERTEX_POINT('',#41236);
#10802=VERTEX_POINT('',#41242);
#10803=VERTEX_POINT('',#41248);
#10804=VERTEX_POINT('',#41249);
#10805=VERTEX_POINT('',#41251);
#10806=VERTEX_POINT('',#41255);
#10807=VERTEX_POINT('',#41257);
#10808=VERTEX_POINT('',#41263);
#10809=VERTEX_POINT('',#41269);
#10810=VERTEX_POINT('',#41270);
#10811=VERTEX_POINT('',#41272);
#10812=VERTEX_POINT('',#41276);
#10813=VERTEX_POINT('',#41278);
#10814=VERTEX_POINT('',#41284);
#10815=VERTEX_POINT('',#41290);
#10816=VERTEX_POINT('',#41291);
#10817=VERTEX_POINT('',#41293);
#10818=VERTEX_POINT('',#41297);
#10819=VERTEX_POINT('',#41299);
#10820=VERTEX_POINT('',#41305);
#10821=VERTEX_POINT('',#41311);
#10822=VERTEX_POINT('',#41312);
#10823=VERTEX_POINT('',#41314);
#10824=VERTEX_POINT('',#41318);
#10825=VERTEX_POINT('',#41320);
#10826=VERTEX_POINT('',#41326);
#10827=VERTEX_POINT('',#41332);
#10828=VERTEX_POINT('',#41333);
#10829=VERTEX_POINT('',#41335);
#10830=VERTEX_POINT('',#41339);
#10831=VERTEX_POINT('',#41341);
#10832=VERTEX_POINT('',#41347);
#10833=VERTEX_POINT('',#41353);
#10834=VERTEX_POINT('',#41354);
#10835=VERTEX_POINT('',#41356);
#10836=VERTEX_POINT('',#41360);
#10837=VERTEX_POINT('',#41362);
#10838=VERTEX_POINT('',#41368);
#10839=VERTEX_POINT('',#41374);
#10840=VERTEX_POINT('',#41375);
#10841=VERTEX_POINT('',#41377);
#10842=VERTEX_POINT('',#41381);
#10843=VERTEX_POINT('',#41383);
#10844=VERTEX_POINT('',#41389);
#10845=VERTEX_POINT('',#41395);
#10846=VERTEX_POINT('',#41396);
#10847=VERTEX_POINT('',#41398);
#10848=VERTEX_POINT('',#41402);
#10849=VERTEX_POINT('',#41404);
#10850=VERTEX_POINT('',#41410);
#10851=VERTEX_POINT('',#41416);
#10852=VERTEX_POINT('',#41417);
#10853=VERTEX_POINT('',#41419);
#10854=VERTEX_POINT('',#41423);
#10855=VERTEX_POINT('',#41425);
#10856=VERTEX_POINT('',#41431);
#10857=VERTEX_POINT('',#41437);
#10858=VERTEX_POINT('',#41438);
#10859=VERTEX_POINT('',#41440);
#10860=VERTEX_POINT('',#41444);
#10861=VERTEX_POINT('',#41446);
#10862=VERTEX_POINT('',#41452);
#10863=VERTEX_POINT('',#41458);
#10864=VERTEX_POINT('',#41459);
#10865=VERTEX_POINT('',#41461);
#10866=VERTEX_POINT('',#41465);
#10867=VERTEX_POINT('',#41467);
#10868=VERTEX_POINT('',#41473);
#10869=VERTEX_POINT('',#41479);
#10870=VERTEX_POINT('',#41480);
#10871=VERTEX_POINT('',#41482);
#10872=VERTEX_POINT('',#41486);
#10873=VERTEX_POINT('',#41488);
#10874=VERTEX_POINT('',#41494);
#10875=VERTEX_POINT('',#41500);
#10876=VERTEX_POINT('',#41501);
#10877=VERTEX_POINT('',#41503);
#10878=VERTEX_POINT('',#41507);
#10879=VERTEX_POINT('',#41509);
#10880=VERTEX_POINT('',#41515);
#10881=VERTEX_POINT('',#41521);
#10882=VERTEX_POINT('',#41522);
#10883=VERTEX_POINT('',#41524);
#10884=VERTEX_POINT('',#41528);
#10885=VERTEX_POINT('',#41530);
#10886=VERTEX_POINT('',#41536);
#10887=VERTEX_POINT('',#41559);
#10888=VERTEX_POINT('',#41579);
#10889=VERTEX_POINT('',#41581);
#10890=VERTEX_POINT('',#41583);
#10891=VERTEX_POINT('',#41585);
#10892=VERTEX_POINT('',#41589);
#10893=VERTEX_POINT('',#41591);
#10894=VERTEX_POINT('',#41603);
#10895=VERTEX_POINT('',#41607);
#10896=VERTEX_POINT('',#41608);
#10897=VERTEX_POINT('',#41612);
#10898=VERTEX_POINT('',#41613);
#10899=VERTEX_POINT('',#41615);
#10900=VERTEX_POINT('',#41617);
#10901=VERTEX_POINT('',#41621);
#10902=VERTEX_POINT('',#41623);
#10903=VERTEX_POINT('',#41627);
#10904=VERTEX_POINT('',#41629);
#10905=VERTEX_POINT('',#41633);
#10906=VERTEX_POINT('',#41635);
#10907=VERTEX_POINT('',#41639);
#10908=VERTEX_POINT('',#41641);
#10909=VERTEX_POINT('',#41649);
#10910=VERTEX_POINT('',#41656);
#13408=EDGE_CURVE('',#10607,#10608,#6902,.T.);
#13409=EDGE_CURVE('',#10607,#10609,#489,.T.);
#13410=EDGE_CURVE('',#10609,#10610,#5594,.T.);
#13411=EDGE_CURVE('',#10610,#10611,#6903,.T.);
#13412=EDGE_CURVE('',#10611,#10611,#5595,.T.);
#13413=EDGE_CURVE('',#10610,#10612,#5596,.T.);
#13414=EDGE_CURVE('',#10612,#10608,#490,.T.);
#13415=EDGE_CURVE('',#10613,#10614,#6904,.T.);
#13416=EDGE_CURVE('',#10613,#10607,#491,.T.);
#13417=EDGE_CURVE('',#10608,#10614,#492,.T.);
#13418=EDGE_CURVE('',#10615,#10616,#6905,.T.);
#13419=EDGE_CURVE('',#10615,#10613,#493,.T.);
#13420=EDGE_CURVE('',#10614,#10616,#494,.T.);
#13421=EDGE_CURVE('',#10617,#10618,#6906,.T.);
#13422=EDGE_CURVE('',#10617,#10615,#495,.T.);
#13423=EDGE_CURVE('',#10616,#10618,#496,.T.);
#13424=EDGE_CURVE('',#10619,#10620,#6907,.T.);
#13425=EDGE_CURVE('',#10619,#10617,#497,.T.);
#13426=EDGE_CURVE('',#10618,#10620,#498,.T.);
#13427=EDGE_CURVE('',#10621,#10622,#6908,.T.);
#13428=EDGE_CURVE('',#10621,#10619,#499,.T.);
#13429=EDGE_CURVE('',#10620,#10622,#500,.T.);
#13430=EDGE_CURVE('',#10623,#10624,#6909,.T.);
#13431=EDGE_CURVE('',#10623,#10621,#501,.T.);
#13432=EDGE_CURVE('',#10622,#10624,#502,.T.);
#13433=EDGE_CURVE('',#10625,#10626,#6910,.T.);
#13434=EDGE_CURVE('',#10625,#10623,#503,.T.);
#13435=EDGE_CURVE('',#10624,#10626,#504,.T.);
#13436=EDGE_CURVE('',#10627,#10628,#6911,.T.);
#13437=EDGE_CURVE('',#10627,#10625,#505,.T.);
#13438=EDGE_CURVE('',#10626,#10628,#506,.T.);
#13439=EDGE_CURVE('',#10629,#10630,#6912,.T.);
#13440=EDGE_CURVE('',#10629,#10627,#507,.T.);
#13441=EDGE_CURVE('',#10628,#10630,#508,.T.);
#13442=EDGE_CURVE('',#10631,#10632,#6913,.T.);
#13443=EDGE_CURVE('',#10631,#10629,#509,.T.);
#13444=EDGE_CURVE('',#10630,#10632,#510,.T.);
#13445=EDGE_CURVE('',#10633,#10634,#6914,.T.);
#13446=EDGE_CURVE('',#10633,#10631,#511,.T.);
#13447=EDGE_CURVE('',#10632,#10634,#512,.T.);
#13448=EDGE_CURVE('',#10635,#10636,#6915,.T.);
#13449=EDGE_CURVE('',#10635,#10633,#513,.T.);
#13450=EDGE_CURVE('',#10634,#10636,#514,.T.);
#13451=EDGE_CURVE('',#10637,#10638,#6916,.T.);
#13452=EDGE_CURVE('',#10637,#10635,#515,.T.);
#13453=EDGE_CURVE('',#10636,#10638,#516,.T.);
#13454=EDGE_CURVE('',#10639,#10640,#6917,.T.);
#13455=EDGE_CURVE('',#10639,#10641,#517,.T.);
#13456=EDGE_CURVE('',#10642,#10641,#5597,.T.);
#13457=EDGE_CURVE('',#10640,#10642,#518,.T.);
#13458=EDGE_CURVE('',#10643,#10644,#6918,.T.);
#13459=EDGE_CURVE('',#10643,#10639,#519,.T.);
#13460=EDGE_CURVE('',#10644,#10640,#520,.T.);
#13461=EDGE_CURVE('',#10645,#10646,#6919,.T.);
#13462=EDGE_CURVE('',#10645,#10643,#521,.T.);
#13463=EDGE_CURVE('',#10646,#10644,#522,.T.);
#13464=EDGE_CURVE('',#10647,#10648,#6920,.T.);
#13465=EDGE_CURVE('',#10647,#10645,#523,.T.);
#13466=EDGE_CURVE('',#10648,#10646,#524,.T.);
#13467=EDGE_CURVE('',#10649,#10650,#6921,.T.);
#13468=EDGE_CURVE('',#10649,#10647,#525,.T.);
#13469=EDGE_CURVE('',#10650,#10648,#526,.T.);
#13470=EDGE_CURVE('',#10651,#10652,#6922,.T.);
#13471=EDGE_CURVE('',#10651,#10649,#527,.T.);
#13472=EDGE_CURVE('',#10652,#10650,#528,.T.);
#13473=EDGE_CURVE('',#10653,#10654,#6923,.T.);
#13474=EDGE_CURVE('',#10653,#10651,#529,.T.);
#13475=EDGE_CURVE('',#10654,#10652,#530,.T.);
#13476=EDGE_CURVE('',#10655,#10656,#6924,.T.);
#13477=EDGE_CURVE('',#10655,#10653,#531,.T.);
#13478=EDGE_CURVE('',#10656,#10654,#532,.T.);
#13479=EDGE_CURVE('',#10657,#10658,#6925,.T.);
#13480=EDGE_CURVE('',#10657,#10655,#533,.T.);
#13481=EDGE_CURVE('',#10658,#10656,#534,.T.);
#13482=EDGE_CURVE('',#10659,#10660,#6926,.T.);
#13483=EDGE_CURVE('',#10659,#10657,#535,.T.);
#13484=EDGE_CURVE('',#10660,#10658,#536,.T.);
#13485=EDGE_CURVE('',#10661,#10662,#6927,.T.);
#13486=EDGE_CURVE('',#10661,#10659,#537,.T.);
#13487=EDGE_CURVE('',#10662,#10660,#538,.T.);
#13488=EDGE_CURVE('',#10663,#10664,#6928,.T.);
#13489=EDGE_CURVE('',#10663,#10661,#539,.T.);
#13490=EDGE_CURVE('',#10664,#10662,#540,.T.);
#13491=EDGE_CURVE('',#10665,#10666,#6929,.T.);
#13492=EDGE_CURVE('',#10665,#10663,#541,.T.);
#13493=EDGE_CURVE('',#10666,#10664,#542,.T.);
#13494=EDGE_CURVE('',#10667,#10668,#6930,.T.);
#13495=EDGE_CURVE('',#10667,#10665,#543,.T.);
#13496=EDGE_CURVE('',#10668,#10666,#544,.T.);
#13497=EDGE_CURVE('',#10669,#10670,#6931,.T.);
#13498=EDGE_CURVE('',#10669,#10667,#545,.T.);
#13499=EDGE_CURVE('',#10670,#10668,#546,.T.);
#13500=EDGE_CURVE('',#10641,#10671,#547,.T.);
#13501=EDGE_CURVE('',#10672,#10671,#5598,.T.);
#13502=EDGE_CURVE('',#10673,#10672,#5599,.T.);
#13503=EDGE_CURVE('',#10673,#10642,#548,.T.);
#13504=EDGE_CURVE('',#10638,#10673,#549,.T.);
#13505=EDGE_CURVE('',#10674,#10612,#550,.T.);
#13506=EDGE_CURVE('',#10674,#10670,#551,.T.);
#13507=EDGE_CURVE('',#10609,#10675,#552,.T.);
#13508=EDGE_CURVE('',#10675,#10674,#5600,.T.);
#13509=EDGE_CURVE('',#10675,#10669,#553,.T.);
#13510=EDGE_CURVE('',#10671,#10637,#554,.T.);
#13511=EDGE_CURVE('',#10676,#10677,#5601,.T.);
#13512=EDGE_CURVE('',#10676,#10678,#6932,.T.);
#13513=EDGE_CURVE('',#10678,#10677,#6933,.T.);
#13514=EDGE_CURVE('',#10677,#10679,#6934,.T.);
#13515=EDGE_CURVE('',#10678,#10680,#6935,.T.);
#13516=EDGE_CURVE('',#10679,#10680,#147,.T.);
#13517=EDGE_CURVE('',#10681,#10676,#6936,.T.);
#13518=EDGE_CURVE('',#10680,#10681,#148,.T.);
#13519=EDGE_CURVE('',#10682,#10683,#5602,.T.);
#13520=EDGE_CURVE('',#10682,#10684,#6937,.T.);
#13521=EDGE_CURVE('',#10684,#10683,#6938,.T.);
#13522=EDGE_CURVE('',#10683,#10685,#6939,.T.);
#13523=EDGE_CURVE('',#10684,#10686,#6940,.T.);
#13524=EDGE_CURVE('',#10685,#10686,#149,.T.);
#13525=EDGE_CURVE('',#10687,#10682,#6941,.T.);
#13526=EDGE_CURVE('',#10686,#10687,#150,.T.);
#13527=EDGE_CURVE('',#10688,#10689,#5603,.T.);
#13528=EDGE_CURVE('',#10688,#10690,#6942,.T.);
#13529=EDGE_CURVE('',#10690,#10689,#6943,.T.);
#13530=EDGE_CURVE('',#10689,#10691,#6944,.T.);
#13531=EDGE_CURVE('',#10690,#10692,#6945,.T.);
#13532=EDGE_CURVE('',#10691,#10692,#151,.T.);
#13533=EDGE_CURVE('',#10693,#10688,#6946,.T.);
#13534=EDGE_CURVE('',#10692,#10693,#152,.T.);
#13535=EDGE_CURVE('',#10694,#10695,#5604,.T.);
#13536=EDGE_CURVE('',#10694,#10696,#6947,.T.);
#13537=EDGE_CURVE('',#10696,#10695,#6948,.T.);
#13538=EDGE_CURVE('',#10695,#10697,#6949,.T.);
#13539=EDGE_CURVE('',#10696,#10698,#6950,.T.);
#13540=EDGE_CURVE('',#10697,#10698,#153,.T.);
#13541=EDGE_CURVE('',#10699,#10694,#6951,.T.);
#13542=EDGE_CURVE('',#10698,#10699,#154,.T.);
#13543=EDGE_CURVE('',#10700,#10701,#5605,.T.);
#13544=EDGE_CURVE('',#10700,#10702,#6952,.T.);
#13545=EDGE_CURVE('',#10702,#10701,#6953,.T.);
#13546=EDGE_CURVE('',#10701,#10703,#6954,.T.);
#13547=EDGE_CURVE('',#10702,#10704,#6955,.T.);
#13548=EDGE_CURVE('',#10703,#10704,#155,.T.);
#13549=EDGE_CURVE('',#10705,#10700,#6956,.T.);
#13550=EDGE_CURVE('',#10704,#10705,#156,.T.);
#13551=EDGE_CURVE('',#10706,#10707,#5606,.T.);
#13552=EDGE_CURVE('',#10706,#10708,#6957,.T.);
#13553=EDGE_CURVE('',#10708,#10707,#6958,.T.);
#13554=EDGE_CURVE('',#10707,#10709,#6959,.T.);
#13555=EDGE_CURVE('',#10708,#10710,#6960,.T.);
#13556=EDGE_CURVE('',#10709,#10710,#157,.T.);
#13557=EDGE_CURVE('',#10711,#10706,#6961,.T.);
#13558=EDGE_CURVE('',#10710,#10711,#158,.T.);
#13559=EDGE_CURVE('',#10712,#10713,#5607,.T.);
#13560=EDGE_CURVE('',#10712,#10714,#6962,.T.);
#13561=EDGE_CURVE('',#10714,#10713,#6963,.T.);
#13562=EDGE_CURVE('',#10713,#10715,#6964,.T.);
#13563=EDGE_CURVE('',#10714,#10716,#6965,.T.);
#13564=EDGE_CURVE('',#10715,#10716,#159,.T.);
#13565=EDGE_CURVE('',#10717,#10712,#6966,.T.);
#13566=EDGE_CURVE('',#10716,#10717,#160,.T.);
#13567=EDGE_CURVE('',#10718,#10719,#5608,.T.);
#13568=EDGE_CURVE('',#10718,#10720,#6967,.T.);
#13569=EDGE_CURVE('',#10720,#10719,#6968,.T.);
#13570=EDGE_CURVE('',#10719,#10721,#6969,.T.);
#13571=EDGE_CURVE('',#10720,#10722,#6970,.T.);
#13572=EDGE_CURVE('',#10721,#10722,#161,.T.);
#13573=EDGE_CURVE('',#10723,#10718,#6971,.T.);
#13574=EDGE_CURVE('',#10722,#10723,#162,.T.);
#13575=EDGE_CURVE('',#10724,#10725,#5609,.T.);
#13576=EDGE_CURVE('',#10724,#10726,#6972,.T.);
#13577=EDGE_CURVE('',#10726,#10725,#6973,.T.);
#13578=EDGE_CURVE('',#10725,#10727,#6974,.T.);
#13579=EDGE_CURVE('',#10726,#10728,#6975,.T.);
#13580=EDGE_CURVE('',#10727,#10728,#163,.T.);
#13581=EDGE_CURVE('',#10729,#10724,#6976,.T.);
#13582=EDGE_CURVE('',#10728,#10729,#164,.T.);
#13583=EDGE_CURVE('',#10730,#10731,#5610,.T.);
#13584=EDGE_CURVE('',#10730,#10732,#6977,.T.);
#13585=EDGE_CURVE('',#10732,#10731,#6978,.T.);
#13586=EDGE_CURVE('',#10731,#10733,#6979,.T.);
#13587=EDGE_CURVE('',#10732,#10734,#6980,.T.);
#13588=EDGE_CURVE('',#10733,#10734,#165,.T.);
#13589=EDGE_CURVE('',#10735,#10730,#6981,.T.);
#13590=EDGE_CURVE('',#10734,#10735,#166,.T.);
#13591=EDGE_CURVE('',#10736,#10737,#5611,.T.);
#13592=EDGE_CURVE('',#10736,#10738,#6982,.T.);
#13593=EDGE_CURVE('',#10738,#10737,#6983,.T.);
#13594=EDGE_CURVE('',#10737,#10739,#6984,.T.);
#13595=EDGE_CURVE('',#10738,#10740,#6985,.T.);
#13596=EDGE_CURVE('',#10739,#10740,#167,.T.);
#13597=EDGE_CURVE('',#10741,#10736,#6986,.T.);
#13598=EDGE_CURVE('',#10740,#10741,#168,.T.);
#13599=EDGE_CURVE('',#10742,#10743,#5612,.T.);
#13600=EDGE_CURVE('',#10742,#10744,#6987,.T.);
#13601=EDGE_CURVE('',#10744,#10743,#6988,.T.);
#13602=EDGE_CURVE('',#10743,#10745,#6989,.T.);
#13603=EDGE_CURVE('',#10744,#10746,#6990,.T.);
#13604=EDGE_CURVE('',#10745,#10746,#169,.T.);
#13605=EDGE_CURVE('',#10747,#10742,#6991,.T.);
#13606=EDGE_CURVE('',#10746,#10747,#170,.T.);
#13607=EDGE_CURVE('',#10748,#10749,#5613,.T.);
#13608=EDGE_CURVE('',#10748,#10750,#6992,.T.);
#13609=EDGE_CURVE('',#10750,#10749,#6993,.T.);
#13610=EDGE_CURVE('',#10749,#10751,#6994,.T.);
#13611=EDGE_CURVE('',#10750,#10752,#6995,.T.);
#13612=EDGE_CURVE('',#10751,#10752,#171,.T.);
#13613=EDGE_CURVE('',#10753,#10748,#6996,.T.);
#13614=EDGE_CURVE('',#10752,#10753,#172,.T.);
#13615=EDGE_CURVE('',#10754,#10755,#5614,.T.);
#13616=EDGE_CURVE('',#10754,#10756,#6997,.T.);
#13617=EDGE_CURVE('',#10756,#10755,#6998,.T.);
#13618=EDGE_CURVE('',#10755,#10757,#6999,.T.);
#13619=EDGE_CURVE('',#10756,#10758,#7000,.T.);
#13620=EDGE_CURVE('',#10757,#10758,#173,.T.);
#13621=EDGE_CURVE('',#10759,#10754,#7001,.T.);
#13622=EDGE_CURVE('',#10758,#10759,#174,.T.);
#13623=EDGE_CURVE('',#10760,#10761,#5615,.T.);
#13624=EDGE_CURVE('',#10760,#10762,#7002,.T.);
#13625=EDGE_CURVE('',#10762,#10761,#7003,.T.);
#13626=EDGE_CURVE('',#10761,#10763,#7004,.T.);
#13627=EDGE_CURVE('',#10762,#10764,#7005,.T.);
#13628=EDGE_CURVE('',#10763,#10764,#175,.T.);
#13629=EDGE_CURVE('',#10765,#10760,#7006,.T.);
#13630=EDGE_CURVE('',#10764,#10765,#176,.T.);
#13631=EDGE_CURVE('',#10766,#10767,#5616,.T.);
#13632=EDGE_CURVE('',#10766,#10768,#7007,.T.);
#13633=EDGE_CURVE('',#10768,#10767,#7008,.T.);
#13634=EDGE_CURVE('',#10767,#10769,#7009,.T.);
#13635=EDGE_CURVE('',#10768,#10770,#7010,.T.);
#13636=EDGE_CURVE('',#10769,#10770,#177,.T.);
#13637=EDGE_CURVE('',#10771,#10766,#7011,.T.);
#13638=EDGE_CURVE('',#10770,#10771,#178,.T.);
#13639=EDGE_CURVE('',#10772,#10773,#5617,.T.);
#13640=EDGE_CURVE('',#10772,#10774,#7012,.T.);
#13641=EDGE_CURVE('',#10774,#10773,#7013,.T.);
#13642=EDGE_CURVE('',#10773,#10775,#7014,.T.);
#13643=EDGE_CURVE('',#10774,#10776,#7015,.T.);
#13644=EDGE_CURVE('',#10775,#10776,#179,.T.);
#13645=EDGE_CURVE('',#10777,#10772,#7016,.T.);
#13646=EDGE_CURVE('',#10776,#10777,#180,.T.);
#13647=EDGE_CURVE('',#10778,#10779,#5618,.T.);
#13648=EDGE_CURVE('',#10778,#10780,#7017,.T.);
#13649=EDGE_CURVE('',#10780,#10781,#7018,.T.);
#13650=EDGE_CURVE('',#10779,#10781,#5619,.T.);
#13651=EDGE_CURVE('',#10781,#10782,#7019,.T.);
#13652=EDGE_CURVE('',#10780,#10783,#7020,.T.);
#13653=EDGE_CURVE('',#10782,#10783,#181,.T.);
#13654=EDGE_CURVE('',#10784,#10778,#7021,.T.);
#13655=EDGE_CURVE('',#10783,#10784,#182,.T.);
#13656=EDGE_CURVE('',#10785,#10786,#5620,.T.);
#13657=EDGE_CURVE('',#10785,#10787,#7022,.T.);
#13658=EDGE_CURVE('',#10787,#10786,#7023,.T.);
#13659=EDGE_CURVE('',#10786,#10788,#7024,.T.);
#13660=EDGE_CURVE('',#10787,#10789,#7025,.T.);
#13661=EDGE_CURVE('',#10788,#10789,#183,.T.);
#13662=EDGE_CURVE('',#10790,#10785,#7026,.T.);
#13663=EDGE_CURVE('',#10789,#10790,#184,.T.);
#13664=EDGE_CURVE('',#10791,#10792,#5621,.T.);
#13665=EDGE_CURVE('',#10791,#10793,#7027,.T.);
#13666=EDGE_CURVE('',#10793,#10792,#7028,.T.);
#13667=EDGE_CURVE('',#10792,#10794,#7029,.T.);
#13668=EDGE_CURVE('',#10793,#10795,#7030,.T.);
#13669=EDGE_CURVE('',#10794,#10795,#185,.T.);
#13670=EDGE_CURVE('',#10796,#10791,#7031,.T.);
#13671=EDGE_CURVE('',#10795,#10796,#186,.T.);
#13672=EDGE_CURVE('',#10797,#10798,#5622,.T.);
#13673=EDGE_CURVE('',#10797,#10799,#7032,.T.);
#13674=EDGE_CURVE('',#10799,#10798,#7033,.T.);
#13675=EDGE_CURVE('',#10798,#10800,#7034,.T.);
#13676=EDGE_CURVE('',#10799,#10801,#7035,.T.);
#13677=EDGE_CURVE('',#10800,#10801,#187,.T.);
#13678=EDGE_CURVE('',#10802,#10797,#7036,.T.);
#13679=EDGE_CURVE('',#10801,#10802,#188,.T.);
#13680=EDGE_CURVE('',#10803,#10804,#5623,.T.);
#13681=EDGE_CURVE('',#10803,#10805,#7037,.T.);
#13682=EDGE_CURVE('',#10805,#10804,#7038,.T.);
#13683=EDGE_CURVE('',#10804,#10806,#7039,.T.);
#13684=EDGE_CURVE('',#10805,#10807,#7040,.T.);
#13685=EDGE_CURVE('',#10806,#10807,#189,.T.);
#13686=EDGE_CURVE('',#10808,#10803,#7041,.T.);
#13687=EDGE_CURVE('',#10807,#10808,#190,.T.);
#13688=EDGE_CURVE('',#10809,#10810,#5624,.T.);
#13689=EDGE_CURVE('',#10809,#10811,#7042,.T.);
#13690=EDGE_CURVE('',#10811,#10810,#7043,.T.);
#13691=EDGE_CURVE('',#10810,#10812,#7044,.T.);
#13692=EDGE_CURVE('',#10811,#10813,#7045,.T.);
#13693=EDGE_CURVE('',#10812,#10813,#191,.T.);
#13694=EDGE_CURVE('',#10814,#10809,#7046,.T.);
#13695=EDGE_CURVE('',#10813,#10814,#192,.T.);
#13696=EDGE_CURVE('',#10815,#10816,#5625,.T.);
#13697=EDGE_CURVE('',#10815,#10817,#7047,.T.);
#13698=EDGE_CURVE('',#10817,#10816,#7048,.T.);
#13699=EDGE_CURVE('',#10816,#10818,#7049,.T.);
#13700=EDGE_CURVE('',#10817,#10819,#7050,.T.);
#13701=EDGE_CURVE('',#10818,#10819,#193,.T.);
#13702=EDGE_CURVE('',#10820,#10815,#7051,.T.);
#13703=EDGE_CURVE('',#10819,#10820,#194,.T.);
#13704=EDGE_CURVE('',#10821,#10822,#5626,.T.);
#13705=EDGE_CURVE('',#10821,#10823,#7052,.T.);
#13706=EDGE_CURVE('',#10823,#10822,#7053,.T.);
#13707=EDGE_CURVE('',#10822,#10824,#7054,.T.);
#13708=EDGE_CURVE('',#10823,#10825,#7055,.T.);
#13709=EDGE_CURVE('',#10824,#10825,#195,.T.);
#13710=EDGE_CURVE('',#10826,#10821,#7056,.T.);
#13711=EDGE_CURVE('',#10825,#10826,#196,.T.);
#13712=EDGE_CURVE('',#10827,#10828,#5627,.T.);
#13713=EDGE_CURVE('',#10827,#10829,#7057,.T.);
#13714=EDGE_CURVE('',#10829,#10828,#7058,.T.);
#13715=EDGE_CURVE('',#10828,#10830,#7059,.T.);
#13716=EDGE_CURVE('',#10829,#10831,#7060,.T.);
#13717=EDGE_CURVE('',#10830,#10831,#197,.T.);
#13718=EDGE_CURVE('',#10832,#10827,#7061,.T.);
#13719=EDGE_CURVE('',#10831,#10832,#198,.T.);
#13720=EDGE_CURVE('',#10833,#10834,#5628,.T.);
#13721=EDGE_CURVE('',#10833,#10835,#7062,.T.);
#13722=EDGE_CURVE('',#10835,#10834,#7063,.T.);
#13723=EDGE_CURVE('',#10834,#10836,#7064,.T.);
#13724=EDGE_CURVE('',#10835,#10837,#7065,.T.);
#13725=EDGE_CURVE('',#10836,#10837,#199,.T.);
#13726=EDGE_CURVE('',#10838,#10833,#7066,.T.);
#13727=EDGE_CURVE('',#10837,#10838,#200,.T.);
#13728=EDGE_CURVE('',#10839,#10840,#5629,.T.);
#13729=EDGE_CURVE('',#10839,#10841,#7067,.T.);
#13730=EDGE_CURVE('',#10841,#10840,#7068,.T.);
#13731=EDGE_CURVE('',#10840,#10842,#7069,.T.);
#13732=EDGE_CURVE('',#10841,#10843,#7070,.T.);
#13733=EDGE_CURVE('',#10842,#10843,#201,.T.);
#13734=EDGE_CURVE('',#10844,#10839,#7071,.T.);
#13735=EDGE_CURVE('',#10843,#10844,#202,.T.);
#13736=EDGE_CURVE('',#10845,#10846,#5630,.T.);
#13737=EDGE_CURVE('',#10845,#10847,#7072,.T.);
#13738=EDGE_CURVE('',#10847,#10846,#7073,.T.);
#13739=EDGE_CURVE('',#10846,#10848,#7074,.T.);
#13740=EDGE_CURVE('',#10847,#10849,#7075,.T.);
#13741=EDGE_CURVE('',#10848,#10849,#203,.T.);
#13742=EDGE_CURVE('',#10850,#10845,#7076,.T.);
#13743=EDGE_CURVE('',#10849,#10850,#204,.T.);
#13744=EDGE_CURVE('',#10851,#10852,#5631,.T.);
#13745=EDGE_CURVE('',#10851,#10853,#7077,.T.);
#13746=EDGE_CURVE('',#10853,#10852,#7078,.T.);
#13747=EDGE_CURVE('',#10852,#10854,#7079,.T.);
#13748=EDGE_CURVE('',#10853,#10855,#7080,.T.);
#13749=EDGE_CURVE('',#10854,#10855,#205,.T.);
#13750=EDGE_CURVE('',#10856,#10851,#7081,.T.);
#13751=EDGE_CURVE('',#10855,#10856,#206,.T.);
#13752=EDGE_CURVE('',#10857,#10858,#5632,.T.);
#13753=EDGE_CURVE('',#10857,#10859,#7082,.T.);
#13754=EDGE_CURVE('',#10859,#10858,#7083,.T.);
#13755=EDGE_CURVE('',#10858,#10860,#7084,.T.);
#13756=EDGE_CURVE('',#10859,#10861,#7085,.T.);
#13757=EDGE_CURVE('',#10860,#10861,#207,.T.);
#13758=EDGE_CURVE('',#10862,#10857,#7086,.T.);
#13759=EDGE_CURVE('',#10861,#10862,#208,.T.);
#13760=EDGE_CURVE('',#10863,#10864,#5633,.T.);
#13761=EDGE_CURVE('',#10863,#10865,#7087,.T.);
#13762=EDGE_CURVE('',#10865,#10864,#7088,.T.);
#13763=EDGE_CURVE('',#10864,#10866,#7089,.T.);
#13764=EDGE_CURVE('',#10865,#10867,#7090,.T.);
#13765=EDGE_CURVE('',#10866,#10867,#209,.T.);
#13766=EDGE_CURVE('',#10868,#10863,#7091,.T.);
#13767=EDGE_CURVE('',#10867,#10868,#210,.T.);
#13768=EDGE_CURVE('',#10869,#10870,#5634,.T.);
#13769=EDGE_CURVE('',#10869,#10871,#7092,.T.);
#13770=EDGE_CURVE('',#10871,#10870,#7093,.T.);
#13771=EDGE_CURVE('',#10870,#10872,#7094,.T.);
#13772=EDGE_CURVE('',#10871,#10873,#7095,.T.);
#13773=EDGE_CURVE('',#10872,#10873,#211,.T.);
#13774=EDGE_CURVE('',#10874,#10869,#7096,.T.);
#13775=EDGE_CURVE('',#10873,#10874,#212,.T.);
#13776=EDGE_CURVE('',#10875,#10876,#5635,.T.);
#13777=EDGE_CURVE('',#10875,#10877,#7097,.T.);
#13778=EDGE_CURVE('',#10877,#10876,#7098,.T.);
#13779=EDGE_CURVE('',#10876,#10878,#7099,.T.);
#13780=EDGE_CURVE('',#10877,#10879,#7100,.T.);
#13781=EDGE_CURVE('',#10878,#10879,#213,.T.);
#13782=EDGE_CURVE('',#10880,#10875,#7101,.T.);
#13783=EDGE_CURVE('',#10879,#10880,#214,.T.);
#13784=EDGE_CURVE('',#10881,#10882,#5636,.T.);
#13785=EDGE_CURVE('',#10881,#10883,#7102,.T.);
#13786=EDGE_CURVE('',#10883,#10882,#7103,.T.);
#13787=EDGE_CURVE('',#10882,#10884,#7104,.T.);
#13788=EDGE_CURVE('',#10883,#10885,#7105,.T.);
#13789=EDGE_CURVE('',#10884,#10885,#215,.T.);
#13790=EDGE_CURVE('',#10886,#10881,#7106,.T.);
#13791=EDGE_CURVE('',#10885,#10886,#216,.T.);
#13792=EDGE_CURVE('',#10687,#10679,#5637,.T.);
#13793=EDGE_CURVE('',#10693,#10685,#5638,.T.);
#13794=EDGE_CURVE('',#10699,#10691,#5639,.T.);
#13795=EDGE_CURVE('',#10705,#10697,#5640,.T.);
#13796=EDGE_CURVE('',#10711,#10703,#5641,.T.);
#13797=EDGE_CURVE('',#10717,#10709,#5642,.T.);
#13798=EDGE_CURVE('',#10723,#10715,#5643,.T.);
#13799=EDGE_CURVE('',#10729,#10721,#5644,.T.);
#13800=EDGE_CURVE('',#10735,#10727,#5645,.T.);
#13801=EDGE_CURVE('',#10741,#10733,#5646,.T.);
#13802=EDGE_CURVE('',#10747,#10739,#5647,.T.);
#13803=EDGE_CURVE('',#10753,#10745,#5648,.T.);
#13804=EDGE_CURVE('',#10759,#10751,#5649,.T.);
#13805=EDGE_CURVE('',#10765,#10757,#5650,.T.);
#13806=EDGE_CURVE('',#10771,#10763,#5651,.T.);
#13807=EDGE_CURVE('',#10777,#10769,#5652,.T.);
#13808=EDGE_CURVE('',#10784,#10775,#5653,.T.);
#13809=EDGE_CURVE('',#10779,#10887,#7107,.T.);
#13810=EDGE_CURVE('',#10887,#10887,#5654,.T.);
#13811=EDGE_CURVE('',#10790,#10782,#5655,.T.);
#13812=EDGE_CURVE('',#10796,#10788,#5656,.T.);
#13813=EDGE_CURVE('',#10802,#10794,#5657,.T.);
#13814=EDGE_CURVE('',#10808,#10800,#5658,.T.);
#13815=EDGE_CURVE('',#10814,#10806,#5659,.T.);
#13816=EDGE_CURVE('',#10820,#10812,#5660,.T.);
#13817=EDGE_CURVE('',#10826,#10818,#5661,.T.);
#13818=EDGE_CURVE('',#10832,#10824,#5662,.T.);
#13819=EDGE_CURVE('',#10838,#10830,#5663,.T.);
#13820=EDGE_CURVE('',#10844,#10836,#5664,.T.);
#13821=EDGE_CURVE('',#10850,#10842,#5665,.T.);
#13822=EDGE_CURVE('',#10856,#10848,#5666,.T.);
#13823=EDGE_CURVE('',#10862,#10854,#5667,.T.);
#13824=EDGE_CURVE('',#10868,#10860,#5668,.T.);
#13825=EDGE_CURVE('',#10874,#10866,#5669,.T.);
#13826=EDGE_CURVE('',#10880,#10872,#5670,.T.);
#13827=EDGE_CURVE('',#10886,#10878,#5671,.T.);
#13828=EDGE_CURVE('',#10888,#10884,#5672,.T.);
#13829=EDGE_CURVE('',#10888,#10889,#7108,.T.);
#13830=EDGE_CURVE('',#10889,#10890,#5673,.T.);
#13831=EDGE_CURVE('',#10890,#10891,#7109,.T.);
#13832=EDGE_CURVE('',#10681,#10891,#5674,.T.);
#13833=EDGE_CURVE('',#10892,#10890,#7110,.T.);
#13834=EDGE_CURVE('',#10892,#10893,#7111,.T.);
#13835=EDGE_CURVE('',#10891,#10893,#217,.T.);
#13836=EDGE_CURVE('',#10893,#10888,#218,.T.);
#13837=EDGE_CURVE('',#10889,#10892,#7112,.T.);
#13838=EDGE_CURVE('',#10894,#10894,#5675,.T.);
#13839=EDGE_CURVE('',#10894,#10783,#7113,.T.);
#13840=EDGE_CURVE('',#10895,#10896,#7114,.T.);
#13841=EDGE_CURVE('',#10896,#10896,#5676,.T.);
#13842=EDGE_CURVE('',#10897,#10898,#7115,.T.);
#13843=EDGE_CURVE('',#10897,#10899,#7116,.T.);
#13844=EDGE_CURVE('',#10899,#10900,#7117,.T.);
#13845=EDGE_CURVE('',#10898,#10900,#7118,.T.);
#13846=EDGE_CURVE('',#10901,#10897,#7119,.T.);
#13847=EDGE_CURVE('',#10901,#10902,#7120,.T.);
#13848=EDGE_CURVE('',#10902,#10899,#7121,.T.);
#13849=EDGE_CURVE('',#10903,#10901,#7122,.T.);
#13850=EDGE_CURVE('',#10903,#10904,#7123,.T.);
#13851=EDGE_CURVE('',#10904,#10902,#7124,.T.);
#13852=EDGE_CURVE('',#10905,#10903,#7125,.T.);
#13853=EDGE_CURVE('',#10905,#10906,#7126,.T.);
#13854=EDGE_CURVE('',#10906,#10904,#7127,.T.);
#13855=EDGE_CURVE('',#10907,#10905,#7128,.T.);
#13856=EDGE_CURVE('',#10907,#10908,#7129,.T.);
#13857=EDGE_CURVE('',#10908,#10906,#7130,.T.);
#13858=EDGE_CURVE('',#10898,#10907,#7131,.T.);
#13859=EDGE_CURVE('',#10900,#10908,#7132,.T.);
#13860=EDGE_CURVE('',#10909,#10909,#5677,.T.);
#13861=EDGE_CURVE('',#10611,#10909,#7133,.T.);
#13862=EDGE_CURVE('',#10671,#10673,#5678,.T.);
#13863=EDGE_CURVE('',#10910,#10910,#5679,.T.);
#13864=EDGE_CURVE('',#10910,#10672,#7134,.T.);
#18461=ORIENTED_EDGE('',*,*,#13408,.F.);
#18462=ORIENTED_EDGE('',*,*,#13409,.T.);
#18463=ORIENTED_EDGE('',*,*,#13410,.T.);
#18464=ORIENTED_EDGE('',*,*,#13411,.T.);
#18465=ORIENTED_EDGE('',*,*,#13412,.T.);
#18466=ORIENTED_EDGE('',*,*,#13411,.F.);
#18467=ORIENTED_EDGE('',*,*,#13413,.T.);
#18468=ORIENTED_EDGE('',*,*,#13414,.T.);
#18469=ORIENTED_EDGE('',*,*,#13415,.F.);
#18470=ORIENTED_EDGE('',*,*,#13416,.T.);
#18471=ORIENTED_EDGE('',*,*,#13408,.T.);
#18472=ORIENTED_EDGE('',*,*,#13417,.T.);
#18473=ORIENTED_EDGE('',*,*,#13418,.F.);
#18474=ORIENTED_EDGE('',*,*,#13419,.T.);
#18475=ORIENTED_EDGE('',*,*,#13415,.T.);
#18476=ORIENTED_EDGE('',*,*,#13420,.T.);
#18477=ORIENTED_EDGE('',*,*,#13421,.F.);
#18478=ORIENTED_EDGE('',*,*,#13422,.T.);
#18479=ORIENTED_EDGE('',*,*,#13418,.T.);
#18480=ORIENTED_EDGE('',*,*,#13423,.T.);
#18481=ORIENTED_EDGE('',*,*,#13424,.F.);
#18482=ORIENTED_EDGE('',*,*,#13425,.T.);
#18483=ORIENTED_EDGE('',*,*,#13421,.T.);
#18484=ORIENTED_EDGE('',*,*,#13426,.T.);
#18485=ORIENTED_EDGE('',*,*,#13427,.F.);
#18486=ORIENTED_EDGE('',*,*,#13428,.T.);
#18487=ORIENTED_EDGE('',*,*,#13424,.T.);
#18488=ORIENTED_EDGE('',*,*,#13429,.T.);
#18489=ORIENTED_EDGE('',*,*,#13430,.F.);
#18490=ORIENTED_EDGE('',*,*,#13431,.T.);
#18491=ORIENTED_EDGE('',*,*,#13427,.T.);
#18492=ORIENTED_EDGE('',*,*,#13432,.T.);
#18493=ORIENTED_EDGE('',*,*,#13433,.F.);
#18494=ORIENTED_EDGE('',*,*,#13434,.T.);
#18495=ORIENTED_EDGE('',*,*,#13430,.T.);
#18496=ORIENTED_EDGE('',*,*,#13435,.T.);
#18497=ORIENTED_EDGE('',*,*,#13436,.F.);
#18498=ORIENTED_EDGE('',*,*,#13437,.T.);
#18499=ORIENTED_EDGE('',*,*,#13433,.T.);
#18500=ORIENTED_EDGE('',*,*,#13438,.T.);
#18501=ORIENTED_EDGE('',*,*,#13439,.F.);
#18502=ORIENTED_EDGE('',*,*,#13440,.T.);
#18503=ORIENTED_EDGE('',*,*,#13436,.T.);
#18504=ORIENTED_EDGE('',*,*,#13441,.T.);
#18505=ORIENTED_EDGE('',*,*,#13442,.F.);
#18506=ORIENTED_EDGE('',*,*,#13443,.T.);
#18507=ORIENTED_EDGE('',*,*,#13439,.T.);
#18508=ORIENTED_EDGE('',*,*,#13444,.T.);
#18509=ORIENTED_EDGE('',*,*,#13445,.F.);
#18510=ORIENTED_EDGE('',*,*,#13446,.T.);
#18511=ORIENTED_EDGE('',*,*,#13442,.T.);
#18512=ORIENTED_EDGE('',*,*,#13447,.T.);
#18513=ORIENTED_EDGE('',*,*,#13448,.F.);
#18514=ORIENTED_EDGE('',*,*,#13449,.T.);
#18515=ORIENTED_EDGE('',*,*,#13445,.T.);
#18516=ORIENTED_EDGE('',*,*,#13450,.T.);
#18517=ORIENTED_EDGE('',*,*,#13451,.F.);
#18518=ORIENTED_EDGE('',*,*,#13452,.T.);
#18519=ORIENTED_EDGE('',*,*,#13448,.T.);
#18520=ORIENTED_EDGE('',*,*,#13453,.T.);
#18521=ORIENTED_EDGE('',*,*,#13454,.F.);
#18522=ORIENTED_EDGE('',*,*,#13455,.T.);
#18523=ORIENTED_EDGE('',*,*,#13456,.F.);
#18524=ORIENTED_EDGE('',*,*,#13457,.F.);
#18525=ORIENTED_EDGE('',*,*,#13458,.F.);
#18526=ORIENTED_EDGE('',*,*,#13459,.T.);
#18527=ORIENTED_EDGE('',*,*,#13454,.T.);
#18528=ORIENTED_EDGE('',*,*,#13460,.F.);
#18529=ORIENTED_EDGE('',*,*,#13461,.F.);
#18530=ORIENTED_EDGE('',*,*,#13462,.T.);
#18531=ORIENTED_EDGE('',*,*,#13458,.T.);
#18532=ORIENTED_EDGE('',*,*,#13463,.F.);
#18533=ORIENTED_EDGE('',*,*,#13464,.F.);
#18534=ORIENTED_EDGE('',*,*,#13465,.T.);
#18535=ORIENTED_EDGE('',*,*,#13461,.T.);
#18536=ORIENTED_EDGE('',*,*,#13466,.F.);
#18537=ORIENTED_EDGE('',*,*,#13467,.F.);
#18538=ORIENTED_EDGE('',*,*,#13468,.T.);
#18539=ORIENTED_EDGE('',*,*,#13464,.T.);
#18540=ORIENTED_EDGE('',*,*,#13469,.F.);
#18541=ORIENTED_EDGE('',*,*,#13470,.F.);
#18542=ORIENTED_EDGE('',*,*,#13471,.T.);
#18543=ORIENTED_EDGE('',*,*,#13467,.T.);
#18544=ORIENTED_EDGE('',*,*,#13472,.F.);
#18545=ORIENTED_EDGE('',*,*,#13473,.F.);
#18546=ORIENTED_EDGE('',*,*,#13474,.T.);
#18547=ORIENTED_EDGE('',*,*,#13470,.T.);
#18548=ORIENTED_EDGE('',*,*,#13475,.F.);
#18549=ORIENTED_EDGE('',*,*,#13476,.F.);
#18550=ORIENTED_EDGE('',*,*,#13477,.T.);
#18551=ORIENTED_EDGE('',*,*,#13473,.T.);
#18552=ORIENTED_EDGE('',*,*,#13478,.F.);
#18553=ORIENTED_EDGE('',*,*,#13479,.F.);
#18554=ORIENTED_EDGE('',*,*,#13480,.T.);
#18555=ORIENTED_EDGE('',*,*,#13476,.T.);
#18556=ORIENTED_EDGE('',*,*,#13481,.F.);
#18557=ORIENTED_EDGE('',*,*,#13482,.F.);
#18558=ORIENTED_EDGE('',*,*,#13483,.T.);
#18559=ORIENTED_EDGE('',*,*,#13479,.T.);
#18560=ORIENTED_EDGE('',*,*,#13484,.F.);
#18561=ORIENTED_EDGE('',*,*,#13485,.F.);
#18562=ORIENTED_EDGE('',*,*,#13486,.T.);
#18563=ORIENTED_EDGE('',*,*,#13482,.T.);
#18564=ORIENTED_EDGE('',*,*,#13487,.F.);
#18565=ORIENTED_EDGE('',*,*,#13488,.F.);
#18566=ORIENTED_EDGE('',*,*,#13489,.T.);
#18567=ORIENTED_EDGE('',*,*,#13485,.T.);
#18568=ORIENTED_EDGE('',*,*,#13490,.F.);
#18569=ORIENTED_EDGE('',*,*,#13491,.F.);
#18570=ORIENTED_EDGE('',*,*,#13492,.T.);
#18571=ORIENTED_EDGE('',*,*,#13488,.T.);
#18572=ORIENTED_EDGE('',*,*,#13493,.F.);
#18573=ORIENTED_EDGE('',*,*,#13494,.F.);
#18574=ORIENTED_EDGE('',*,*,#13495,.T.);
#18575=ORIENTED_EDGE('',*,*,#13491,.T.);
#18576=ORIENTED_EDGE('',*,*,#13496,.F.);
#18577=ORIENTED_EDGE('',*,*,#13497,.F.);
#18578=ORIENTED_EDGE('',*,*,#13498,.T.);
#18579=ORIENTED_EDGE('',*,*,#13494,.T.);
#18580=ORIENTED_EDGE('',*,*,#13499,.F.);
#18581=ORIENTED_EDGE('',*,*,#13456,.T.);
#18582=ORIENTED_EDGE('',*,*,#13500,.T.);
#18583=ORIENTED_EDGE('',*,*,#13501,.F.);
#18584=ORIENTED_EDGE('',*,*,#13502,.F.);
#18585=ORIENTED_EDGE('',*,*,#13503,.T.);
#18586=ORIENTED_EDGE('',*,*,#13503,.F.);
#18587=ORIENTED_EDGE('',*,*,#13504,.F.);
#18588=ORIENTED_EDGE('',*,*,#13453,.F.);
#18589=ORIENTED_EDGE('',*,*,#13450,.F.);
#18590=ORIENTED_EDGE('',*,*,#13447,.F.);
#18591=ORIENTED_EDGE('',*,*,#13444,.F.);
#18592=ORIENTED_EDGE('',*,*,#13441,.F.);
#18593=ORIENTED_EDGE('',*,*,#13438,.F.);
#18594=ORIENTED_EDGE('',*,*,#13435,.F.);
#18595=ORIENTED_EDGE('',*,*,#13432,.F.);
#18596=ORIENTED_EDGE('',*,*,#13429,.F.);
#18597=ORIENTED_EDGE('',*,*,#13426,.F.);
#18598=ORIENTED_EDGE('',*,*,#13423,.F.);
#18599=ORIENTED_EDGE('',*,*,#13420,.F.);
#18600=ORIENTED_EDGE('',*,*,#13417,.F.);
#18601=ORIENTED_EDGE('',*,*,#13414,.F.);
#18602=ORIENTED_EDGE('',*,*,#13505,.F.);
#18603=ORIENTED_EDGE('',*,*,#13506,.T.);
#18604=ORIENTED_EDGE('',*,*,#13499,.T.);
#18605=ORIENTED_EDGE('',*,*,#13496,.T.);
#18606=ORIENTED_EDGE('',*,*,#13493,.T.);
#18607=ORIENTED_EDGE('',*,*,#13490,.T.);
#18608=ORIENTED_EDGE('',*,*,#13487,.T.);
#18609=ORIENTED_EDGE('',*,*,#13484,.T.);
#18610=ORIENTED_EDGE('',*,*,#13481,.T.);
#18611=ORIENTED_EDGE('',*,*,#13478,.T.);
#18612=ORIENTED_EDGE('',*,*,#13475,.T.);
#18613=ORIENTED_EDGE('',*,*,#13472,.T.);
#18614=ORIENTED_EDGE('',*,*,#13469,.T.);
#18615=ORIENTED_EDGE('',*,*,#13466,.T.);
#18616=ORIENTED_EDGE('',*,*,#13463,.T.);
#18617=ORIENTED_EDGE('',*,*,#13460,.T.);
#18618=ORIENTED_EDGE('',*,*,#13457,.T.);
#18619=ORIENTED_EDGE('',*,*,#13410,.F.);
#18620=ORIENTED_EDGE('',*,*,#13507,.T.);
#18621=ORIENTED_EDGE('',*,*,#13508,.T.);
#18622=ORIENTED_EDGE('',*,*,#13505,.T.);
#18623=ORIENTED_EDGE('',*,*,#13413,.F.);
#18624=ORIENTED_EDGE('',*,*,#13497,.T.);
#18625=ORIENTED_EDGE('',*,*,#13506,.F.);
#18626=ORIENTED_EDGE('',*,*,#13508,.F.);
#18627=ORIENTED_EDGE('',*,*,#13509,.T.);
#18628=ORIENTED_EDGE('',*,*,#13500,.F.);
#18629=ORIENTED_EDGE('',*,*,#13455,.F.);
#18630=ORIENTED_EDGE('',*,*,#13459,.F.);
#18631=ORIENTED_EDGE('',*,*,#13462,.F.);
#18632=ORIENTED_EDGE('',*,*,#13465,.F.);
#18633=ORIENTED_EDGE('',*,*,#13468,.F.);
#18634=ORIENTED_EDGE('',*,*,#13471,.F.);
#18635=ORIENTED_EDGE('',*,*,#13474,.F.);
#18636=ORIENTED_EDGE('',*,*,#13477,.F.);
#18637=ORIENTED_EDGE('',*,*,#13480,.F.);
#18638=ORIENTED_EDGE('',*,*,#13483,.F.);
#18639=ORIENTED_EDGE('',*,*,#13486,.F.);
#18640=ORIENTED_EDGE('',*,*,#13489,.F.);
#18641=ORIENTED_EDGE('',*,*,#13492,.F.);
#18642=ORIENTED_EDGE('',*,*,#13495,.F.);
#18643=ORIENTED_EDGE('',*,*,#13498,.F.);
#18644=ORIENTED_EDGE('',*,*,#13509,.F.);
#18645=ORIENTED_EDGE('',*,*,#13507,.F.);
#18646=ORIENTED_EDGE('',*,*,#13409,.F.);
#18647=ORIENTED_EDGE('',*,*,#13416,.F.);
#18648=ORIENTED_EDGE('',*,*,#13419,.F.);
#18649=ORIENTED_EDGE('',*,*,#13422,.F.);
#18650=ORIENTED_EDGE('',*,*,#13425,.F.);
#18651=ORIENTED_EDGE('',*,*,#13428,.F.);
#18652=ORIENTED_EDGE('',*,*,#13431,.F.);
#18653=ORIENTED_EDGE('',*,*,#13434,.F.);
#18654=ORIENTED_EDGE('',*,*,#13437,.F.);
#18655=ORIENTED_EDGE('',*,*,#13440,.F.);
#18656=ORIENTED_EDGE('',*,*,#13443,.F.);
#18657=ORIENTED_EDGE('',*,*,#13446,.F.);
#18658=ORIENTED_EDGE('',*,*,#13449,.F.);
#18659=ORIENTED_EDGE('',*,*,#13452,.F.);
#18660=ORIENTED_EDGE('',*,*,#13510,.F.);
#18661=ORIENTED_EDGE('',*,*,#13511,.F.);
#18662=ORIENTED_EDGE('',*,*,#13512,.T.);
#18663=ORIENTED_EDGE('',*,*,#13513,.T.);
#18664=ORIENTED_EDGE('',*,*,#13514,.F.);
#18665=ORIENTED_EDGE('',*,*,#13513,.F.);
#18666=ORIENTED_EDGE('',*,*,#13515,.T.);
#18667=ORIENTED_EDGE('',*,*,#13516,.F.);
#18668=ORIENTED_EDGE('',*,*,#13517,.F.);
#18669=ORIENTED_EDGE('',*,*,#13518,.F.);
#18670=ORIENTED_EDGE('',*,*,#13515,.F.);
#18671=ORIENTED_EDGE('',*,*,#13512,.F.);
#18672=ORIENTED_EDGE('',*,*,#13519,.F.);
#18673=ORIENTED_EDGE('',*,*,#13520,.T.);
#18674=ORIENTED_EDGE('',*,*,#13521,.T.);
#18675=ORIENTED_EDGE('',*,*,#13522,.F.);
#18676=ORIENTED_EDGE('',*,*,#13521,.F.);
#18677=ORIENTED_EDGE('',*,*,#13523,.T.);
#18678=ORIENTED_EDGE('',*,*,#13524,.F.);
#18679=ORIENTED_EDGE('',*,*,#13525,.F.);
#18680=ORIENTED_EDGE('',*,*,#13526,.F.);
#18681=ORIENTED_EDGE('',*,*,#13523,.F.);
#18682=ORIENTED_EDGE('',*,*,#13520,.F.);
#18683=ORIENTED_EDGE('',*,*,#13527,.F.);
#18684=ORIENTED_EDGE('',*,*,#13528,.T.);
#18685=ORIENTED_EDGE('',*,*,#13529,.T.);
#18686=ORIENTED_EDGE('',*,*,#13530,.F.);
#18687=ORIENTED_EDGE('',*,*,#13529,.F.);
#18688=ORIENTED_EDGE('',*,*,#13531,.T.);
#18689=ORIENTED_EDGE('',*,*,#13532,.F.);
#18690=ORIENTED_EDGE('',*,*,#13533,.F.);
#18691=ORIENTED_EDGE('',*,*,#13534,.F.);
#18692=ORIENTED_EDGE('',*,*,#13531,.F.);
#18693=ORIENTED_EDGE('',*,*,#13528,.F.);
#18694=ORIENTED_EDGE('',*,*,#13535,.F.);
#18695=ORIENTED_EDGE('',*,*,#13536,.T.);
#18696=ORIENTED_EDGE('',*,*,#13537,.T.);
#18697=ORIENTED_EDGE('',*,*,#13538,.F.);
#18698=ORIENTED_EDGE('',*,*,#13537,.F.);
#18699=ORIENTED_EDGE('',*,*,#13539,.T.);
#18700=ORIENTED_EDGE('',*,*,#13540,.F.);
#18701=ORIENTED_EDGE('',*,*,#13541,.F.);
#18702=ORIENTED_EDGE('',*,*,#13542,.F.);
#18703=ORIENTED_EDGE('',*,*,#13539,.F.);
#18704=ORIENTED_EDGE('',*,*,#13536,.F.);
#18705=ORIENTED_EDGE('',*,*,#13543,.F.);
#18706=ORIENTED_EDGE('',*,*,#13544,.T.);
#18707=ORIENTED_EDGE('',*,*,#13545,.T.);
#18708=ORIENTED_EDGE('',*,*,#13546,.F.);
#18709=ORIENTED_EDGE('',*,*,#13545,.F.);
#18710=ORIENTED_EDGE('',*,*,#13547,.T.);
#18711=ORIENTED_EDGE('',*,*,#13548,.F.);
#18712=ORIENTED_EDGE('',*,*,#13549,.F.);
#18713=ORIENTED_EDGE('',*,*,#13550,.F.);
#18714=ORIENTED_EDGE('',*,*,#13547,.F.);
#18715=ORIENTED_EDGE('',*,*,#13544,.F.);
#18716=ORIENTED_EDGE('',*,*,#13551,.F.);
#18717=ORIENTED_EDGE('',*,*,#13552,.T.);
#18718=ORIENTED_EDGE('',*,*,#13553,.T.);
#18719=ORIENTED_EDGE('',*,*,#13554,.F.);
#18720=ORIENTED_EDGE('',*,*,#13553,.F.);
#18721=ORIENTED_EDGE('',*,*,#13555,.T.);
#18722=ORIENTED_EDGE('',*,*,#13556,.F.);
#18723=ORIENTED_EDGE('',*,*,#13557,.F.);
#18724=ORIENTED_EDGE('',*,*,#13558,.F.);
#18725=ORIENTED_EDGE('',*,*,#13555,.F.);
#18726=ORIENTED_EDGE('',*,*,#13552,.F.);
#18727=ORIENTED_EDGE('',*,*,#13559,.F.);
#18728=ORIENTED_EDGE('',*,*,#13560,.T.);
#18729=ORIENTED_EDGE('',*,*,#13561,.T.);
#18730=ORIENTED_EDGE('',*,*,#13562,.F.);
#18731=ORIENTED_EDGE('',*,*,#13561,.F.);
#18732=ORIENTED_EDGE('',*,*,#13563,.T.);
#18733=ORIENTED_EDGE('',*,*,#13564,.F.);
#18734=ORIENTED_EDGE('',*,*,#13565,.F.);
#18735=ORIENTED_EDGE('',*,*,#13566,.F.);
#18736=ORIENTED_EDGE('',*,*,#13563,.F.);
#18737=ORIENTED_EDGE('',*,*,#13560,.F.);
#18738=ORIENTED_EDGE('',*,*,#13567,.F.);
#18739=ORIENTED_EDGE('',*,*,#13568,.T.);
#18740=ORIENTED_EDGE('',*,*,#13569,.T.);
#18741=ORIENTED_EDGE('',*,*,#13570,.F.);
#18742=ORIENTED_EDGE('',*,*,#13569,.F.);
#18743=ORIENTED_EDGE('',*,*,#13571,.T.);
#18744=ORIENTED_EDGE('',*,*,#13572,.F.);
#18745=ORIENTED_EDGE('',*,*,#13573,.F.);
#18746=ORIENTED_EDGE('',*,*,#13574,.F.);
#18747=ORIENTED_EDGE('',*,*,#13571,.F.);
#18748=ORIENTED_EDGE('',*,*,#13568,.F.);
#18749=ORIENTED_EDGE('',*,*,#13575,.F.);
#18750=ORIENTED_EDGE('',*,*,#13576,.T.);
#18751=ORIENTED_EDGE('',*,*,#13577,.T.);
#18752=ORIENTED_EDGE('',*,*,#13578,.F.);
#18753=ORIENTED_EDGE('',*,*,#13577,.F.);
#18754=ORIENTED_EDGE('',*,*,#13579,.T.);
#18755=ORIENTED_EDGE('',*,*,#13580,.F.);
#18756=ORIENTED_EDGE('',*,*,#13581,.F.);
#18757=ORIENTED_EDGE('',*,*,#13582,.F.);
#18758=ORIENTED_EDGE('',*,*,#13579,.F.);
#18759=ORIENTED_EDGE('',*,*,#13576,.F.);
#18760=ORIENTED_EDGE('',*,*,#13583,.F.);
#18761=ORIENTED_EDGE('',*,*,#13584,.T.);
#18762=ORIENTED_EDGE('',*,*,#13585,.T.);
#18763=ORIENTED_EDGE('',*,*,#13586,.F.);
#18764=ORIENTED_EDGE('',*,*,#13585,.F.);
#18765=ORIENTED_EDGE('',*,*,#13587,.T.);
#18766=ORIENTED_EDGE('',*,*,#13588,.F.);
#18767=ORIENTED_EDGE('',*,*,#13589,.F.);
#18768=ORIENTED_EDGE('',*,*,#13590,.F.);
#18769=ORIENTED_EDGE('',*,*,#13587,.F.);
#18770=ORIENTED_EDGE('',*,*,#13584,.F.);
#18771=ORIENTED_EDGE('',*,*,#13591,.F.);
#18772=ORIENTED_EDGE('',*,*,#13592,.T.);
#18773=ORIENTED_EDGE('',*,*,#13593,.T.);
#18774=ORIENTED_EDGE('',*,*,#13594,.F.);
#18775=ORIENTED_EDGE('',*,*,#13593,.F.);
#18776=ORIENTED_EDGE('',*,*,#13595,.T.);
#18777=ORIENTED_EDGE('',*,*,#13596,.F.);
#18778=ORIENTED_EDGE('',*,*,#13597,.F.);
#18779=ORIENTED_EDGE('',*,*,#13598,.F.);
#18780=ORIENTED_EDGE('',*,*,#13595,.F.);
#18781=ORIENTED_EDGE('',*,*,#13592,.F.);
#18782=ORIENTED_EDGE('',*,*,#13599,.F.);
#18783=ORIENTED_EDGE('',*,*,#13600,.T.);
#18784=ORIENTED_EDGE('',*,*,#13601,.T.);
#18785=ORIENTED_EDGE('',*,*,#13602,.F.);
#18786=ORIENTED_EDGE('',*,*,#13601,.F.);
#18787=ORIENTED_EDGE('',*,*,#13603,.T.);
#18788=ORIENTED_EDGE('',*,*,#13604,.F.);
#18789=ORIENTED_EDGE('',*,*,#13605,.F.);
#18790=ORIENTED_EDGE('',*,*,#13606,.F.);
#18791=ORIENTED_EDGE('',*,*,#13603,.F.);
#18792=ORIENTED_EDGE('',*,*,#13600,.F.);
#18793=ORIENTED_EDGE('',*,*,#13607,.F.);
#18794=ORIENTED_EDGE('',*,*,#13608,.T.);
#18795=ORIENTED_EDGE('',*,*,#13609,.T.);
#18796=ORIENTED_EDGE('',*,*,#13610,.F.);
#18797=ORIENTED_EDGE('',*,*,#13609,.F.);
#18798=ORIENTED_EDGE('',*,*,#13611,.T.);
#18799=ORIENTED_EDGE('',*,*,#13612,.F.);
#18800=ORIENTED_EDGE('',*,*,#13613,.F.);
#18801=ORIENTED_EDGE('',*,*,#13614,.F.);
#18802=ORIENTED_EDGE('',*,*,#13611,.F.);
#18803=ORIENTED_EDGE('',*,*,#13608,.F.);
#18804=ORIENTED_EDGE('',*,*,#13615,.F.);
#18805=ORIENTED_EDGE('',*,*,#13616,.T.);
#18806=ORIENTED_EDGE('',*,*,#13617,.T.);
#18807=ORIENTED_EDGE('',*,*,#13618,.F.);
#18808=ORIENTED_EDGE('',*,*,#13617,.F.);
#18809=ORIENTED_EDGE('',*,*,#13619,.T.);
#18810=ORIENTED_EDGE('',*,*,#13620,.F.);
#18811=ORIENTED_EDGE('',*,*,#13621,.F.);
#18812=ORIENTED_EDGE('',*,*,#13622,.F.);
#18813=ORIENTED_EDGE('',*,*,#13619,.F.);
#18814=ORIENTED_EDGE('',*,*,#13616,.F.);
#18815=ORIENTED_EDGE('',*,*,#13623,.F.);
#18816=ORIENTED_EDGE('',*,*,#13624,.T.);
#18817=ORIENTED_EDGE('',*,*,#13625,.T.);
#18818=ORIENTED_EDGE('',*,*,#13626,.F.);
#18819=ORIENTED_EDGE('',*,*,#13625,.F.);
#18820=ORIENTED_EDGE('',*,*,#13627,.T.);
#18821=ORIENTED_EDGE('',*,*,#13628,.F.);
#18822=ORIENTED_EDGE('',*,*,#13629,.F.);
#18823=ORIENTED_EDGE('',*,*,#13630,.F.);
#18824=ORIENTED_EDGE('',*,*,#13627,.F.);
#18825=ORIENTED_EDGE('',*,*,#13624,.F.);
#18826=ORIENTED_EDGE('',*,*,#13631,.F.);
#18827=ORIENTED_EDGE('',*,*,#13632,.T.);
#18828=ORIENTED_EDGE('',*,*,#13633,.T.);
#18829=ORIENTED_EDGE('',*,*,#13634,.F.);
#18830=ORIENTED_EDGE('',*,*,#13633,.F.);
#18831=ORIENTED_EDGE('',*,*,#13635,.T.);
#18832=ORIENTED_EDGE('',*,*,#13636,.F.);
#18833=ORIENTED_EDGE('',*,*,#13637,.F.);
#18834=ORIENTED_EDGE('',*,*,#13638,.F.);
#18835=ORIENTED_EDGE('',*,*,#13635,.F.);
#18836=ORIENTED_EDGE('',*,*,#13632,.F.);
#18837=ORIENTED_EDGE('',*,*,#13639,.F.);
#18838=ORIENTED_EDGE('',*,*,#13640,.T.);
#18839=ORIENTED_EDGE('',*,*,#13641,.T.);
#18840=ORIENTED_EDGE('',*,*,#13642,.F.);
#18841=ORIENTED_EDGE('',*,*,#13641,.F.);
#18842=ORIENTED_EDGE('',*,*,#13643,.T.);
#18843=ORIENTED_EDGE('',*,*,#13644,.F.);
#18844=ORIENTED_EDGE('',*,*,#13645,.F.);
#18845=ORIENTED_EDGE('',*,*,#13646,.F.);
#18846=ORIENTED_EDGE('',*,*,#13643,.F.);
#18847=ORIENTED_EDGE('',*,*,#13640,.F.);
#18848=ORIENTED_EDGE('',*,*,#13647,.F.);
#18849=ORIENTED_EDGE('',*,*,#13648,.T.);
#18850=ORIENTED_EDGE('',*,*,#13649,.T.);
#18851=ORIENTED_EDGE('',*,*,#13650,.F.);
#18852=ORIENTED_EDGE('',*,*,#13651,.F.);
#18853=ORIENTED_EDGE('',*,*,#13649,.F.);
#18854=ORIENTED_EDGE('',*,*,#13652,.T.);
#18855=ORIENTED_EDGE('',*,*,#13653,.F.);
#18856=ORIENTED_EDGE('',*,*,#13654,.F.);
#18857=ORIENTED_EDGE('',*,*,#13655,.F.);
#18858=ORIENTED_EDGE('',*,*,#13652,.F.);
#18859=ORIENTED_EDGE('',*,*,#13648,.F.);
#18860=ORIENTED_EDGE('',*,*,#13656,.F.);
#18861=ORIENTED_EDGE('',*,*,#13657,.T.);
#18862=ORIENTED_EDGE('',*,*,#13658,.T.);
#18863=ORIENTED_EDGE('',*,*,#13659,.F.);
#18864=ORIENTED_EDGE('',*,*,#13658,.F.);
#18865=ORIENTED_EDGE('',*,*,#13660,.T.);
#18866=ORIENTED_EDGE('',*,*,#13661,.F.);
#18867=ORIENTED_EDGE('',*,*,#13662,.F.);
#18868=ORIENTED_EDGE('',*,*,#13663,.F.);
#18869=ORIENTED_EDGE('',*,*,#13660,.F.);
#18870=ORIENTED_EDGE('',*,*,#13657,.F.);
#18871=ORIENTED_EDGE('',*,*,#13664,.F.);
#18872=ORIENTED_EDGE('',*,*,#13665,.T.);
#18873=ORIENTED_EDGE('',*,*,#13666,.T.);
#18874=ORIENTED_EDGE('',*,*,#13667,.F.);
#18875=ORIENTED_EDGE('',*,*,#13666,.F.);
#18876=ORIENTED_EDGE('',*,*,#13668,.T.);
#18877=ORIENTED_EDGE('',*,*,#13669,.F.);
#18878=ORIENTED_EDGE('',*,*,#13670,.F.);
#18879=ORIENTED_EDGE('',*,*,#13671,.F.);
#18880=ORIENTED_EDGE('',*,*,#13668,.F.);
#18881=ORIENTED_EDGE('',*,*,#13665,.F.);
#18882=ORIENTED_EDGE('',*,*,#13672,.F.);
#18883=ORIENTED_EDGE('',*,*,#13673,.T.);
#18884=ORIENTED_EDGE('',*,*,#13674,.T.);
#18885=ORIENTED_EDGE('',*,*,#13675,.F.);
#18886=ORIENTED_EDGE('',*,*,#13674,.F.);
#18887=ORIENTED_EDGE('',*,*,#13676,.T.);
#18888=ORIENTED_EDGE('',*,*,#13677,.F.);
#18889=ORIENTED_EDGE('',*,*,#13678,.F.);
#18890=ORIENTED_EDGE('',*,*,#13679,.F.);
#18891=ORIENTED_EDGE('',*,*,#13676,.F.);
#18892=ORIENTED_EDGE('',*,*,#13673,.F.);
#18893=ORIENTED_EDGE('',*,*,#13680,.F.);
#18894=ORIENTED_EDGE('',*,*,#13681,.T.);
#18895=ORIENTED_EDGE('',*,*,#13682,.T.);
#18896=ORIENTED_EDGE('',*,*,#13683,.F.);
#18897=ORIENTED_EDGE('',*,*,#13682,.F.);
#18898=ORIENTED_EDGE('',*,*,#13684,.T.);
#18899=ORIENTED_EDGE('',*,*,#13685,.F.);
#18900=ORIENTED_EDGE('',*,*,#13686,.F.);
#18901=ORIENTED_EDGE('',*,*,#13687,.F.);
#18902=ORIENTED_EDGE('',*,*,#13684,.F.);
#18903=ORIENTED_EDGE('',*,*,#13681,.F.);
#18904=ORIENTED_EDGE('',*,*,#13688,.F.);
#18905=ORIENTED_EDGE('',*,*,#13689,.T.);
#18906=ORIENTED_EDGE('',*,*,#13690,.T.);
#18907=ORIENTED_EDGE('',*,*,#13691,.F.);
#18908=ORIENTED_EDGE('',*,*,#13690,.F.);
#18909=ORIENTED_EDGE('',*,*,#13692,.T.);
#18910=ORIENTED_EDGE('',*,*,#13693,.F.);
#18911=ORIENTED_EDGE('',*,*,#13694,.F.);
#18912=ORIENTED_EDGE('',*,*,#13695,.F.);
#18913=ORIENTED_EDGE('',*,*,#13692,.F.);
#18914=ORIENTED_EDGE('',*,*,#13689,.F.);
#18915=ORIENTED_EDGE('',*,*,#13696,.F.);
#18916=ORIENTED_EDGE('',*,*,#13697,.T.);
#18917=ORIENTED_EDGE('',*,*,#13698,.T.);
#18918=ORIENTED_EDGE('',*,*,#13699,.F.);
#18919=ORIENTED_EDGE('',*,*,#13698,.F.);
#18920=ORIENTED_EDGE('',*,*,#13700,.T.);
#18921=ORIENTED_EDGE('',*,*,#13701,.F.);
#18922=ORIENTED_EDGE('',*,*,#13702,.F.);
#18923=ORIENTED_EDGE('',*,*,#13703,.F.);
#18924=ORIENTED_EDGE('',*,*,#13700,.F.);
#18925=ORIENTED_EDGE('',*,*,#13697,.F.);
#18926=ORIENTED_EDGE('',*,*,#13704,.F.);
#18927=ORIENTED_EDGE('',*,*,#13705,.T.);
#18928=ORIENTED_EDGE('',*,*,#13706,.T.);
#18929=ORIENTED_EDGE('',*,*,#13707,.F.);
#18930=ORIENTED_EDGE('',*,*,#13706,.F.);
#18931=ORIENTED_EDGE('',*,*,#13708,.T.);
#18932=ORIENTED_EDGE('',*,*,#13709,.F.);
#18933=ORIENTED_EDGE('',*,*,#13710,.F.);
#18934=ORIENTED_EDGE('',*,*,#13711,.F.);
#18935=ORIENTED_EDGE('',*,*,#13708,.F.);
#18936=ORIENTED_EDGE('',*,*,#13705,.F.);
#18937=ORIENTED_EDGE('',*,*,#13712,.F.);
#18938=ORIENTED_EDGE('',*,*,#13713,.T.);
#18939=ORIENTED_EDGE('',*,*,#13714,.T.);
#18940=ORIENTED_EDGE('',*,*,#13715,.F.);
#18941=ORIENTED_EDGE('',*,*,#13714,.F.);
#18942=ORIENTED_EDGE('',*,*,#13716,.T.);
#18943=ORIENTED_EDGE('',*,*,#13717,.F.);
#18944=ORIENTED_EDGE('',*,*,#13718,.F.);
#18945=ORIENTED_EDGE('',*,*,#13719,.F.);
#18946=ORIENTED_EDGE('',*,*,#13716,.F.);
#18947=ORIENTED_EDGE('',*,*,#13713,.F.);
#18948=ORIENTED_EDGE('',*,*,#13720,.F.);
#18949=ORIENTED_EDGE('',*,*,#13721,.T.);
#18950=ORIENTED_EDGE('',*,*,#13722,.T.);
#18951=ORIENTED_EDGE('',*,*,#13723,.F.);
#18952=ORIENTED_EDGE('',*,*,#13722,.F.);
#18953=ORIENTED_EDGE('',*,*,#13724,.T.);
#18954=ORIENTED_EDGE('',*,*,#13725,.F.);
#18955=ORIENTED_EDGE('',*,*,#13726,.F.);
#18956=ORIENTED_EDGE('',*,*,#13727,.F.);
#18957=ORIENTED_EDGE('',*,*,#13724,.F.);
#18958=ORIENTED_EDGE('',*,*,#13721,.F.);
#18959=ORIENTED_EDGE('',*,*,#13728,.F.);
#18960=ORIENTED_EDGE('',*,*,#13729,.T.);
#18961=ORIENTED_EDGE('',*,*,#13730,.T.);
#18962=ORIENTED_EDGE('',*,*,#13731,.F.);
#18963=ORIENTED_EDGE('',*,*,#13730,.F.);
#18964=ORIENTED_EDGE('',*,*,#13732,.T.);
#18965=ORIENTED_EDGE('',*,*,#13733,.F.);
#18966=ORIENTED_EDGE('',*,*,#13734,.F.);
#18967=ORIENTED_EDGE('',*,*,#13735,.F.);
#18968=ORIENTED_EDGE('',*,*,#13732,.F.);
#18969=ORIENTED_EDGE('',*,*,#13729,.F.);
#18970=ORIENTED_EDGE('',*,*,#13736,.F.);
#18971=ORIENTED_EDGE('',*,*,#13737,.T.);
#18972=ORIENTED_EDGE('',*,*,#13738,.T.);
#18973=ORIENTED_EDGE('',*,*,#13739,.F.);
#18974=ORIENTED_EDGE('',*,*,#13738,.F.);
#18975=ORIENTED_EDGE('',*,*,#13740,.T.);
#18976=ORIENTED_EDGE('',*,*,#13741,.F.);
#18977=ORIENTED_EDGE('',*,*,#13742,.F.);
#18978=ORIENTED_EDGE('',*,*,#13743,.F.);
#18979=ORIENTED_EDGE('',*,*,#13740,.F.);
#18980=ORIENTED_EDGE('',*,*,#13737,.F.);
#18981=ORIENTED_EDGE('',*,*,#13744,.F.);
#18982=ORIENTED_EDGE('',*,*,#13745,.T.);
#18983=ORIENTED_EDGE('',*,*,#13746,.T.);
#18984=ORIENTED_EDGE('',*,*,#13747,.F.);
#18985=ORIENTED_EDGE('',*,*,#13746,.F.);
#18986=ORIENTED_EDGE('',*,*,#13748,.T.);
#18987=ORIENTED_EDGE('',*,*,#13749,.F.);
#18988=ORIENTED_EDGE('',*,*,#13750,.F.);
#18989=ORIENTED_EDGE('',*,*,#13751,.F.);
#18990=ORIENTED_EDGE('',*,*,#13748,.F.);
#18991=ORIENTED_EDGE('',*,*,#13745,.F.);
#18992=ORIENTED_EDGE('',*,*,#13752,.F.);
#18993=ORIENTED_EDGE('',*,*,#13753,.T.);
#18994=ORIENTED_EDGE('',*,*,#13754,.T.);
#18995=ORIENTED_EDGE('',*,*,#13755,.F.);
#18996=ORIENTED_EDGE('',*,*,#13754,.F.);
#18997=ORIENTED_EDGE('',*,*,#13756,.T.);
#18998=ORIENTED_EDGE('',*,*,#13757,.F.);
#18999=ORIENTED_EDGE('',*,*,#13758,.F.);
#19000=ORIENTED_EDGE('',*,*,#13759,.F.);
#19001=ORIENTED_EDGE('',*,*,#13756,.F.);
#19002=ORIENTED_EDGE('',*,*,#13753,.F.);
#19003=ORIENTED_EDGE('',*,*,#13760,.F.);
#19004=ORIENTED_EDGE('',*,*,#13761,.T.);
#19005=ORIENTED_EDGE('',*,*,#13762,.T.);
#19006=ORIENTED_EDGE('',*,*,#13763,.F.);
#19007=ORIENTED_EDGE('',*,*,#13762,.F.);
#19008=ORIENTED_EDGE('',*,*,#13764,.T.);
#19009=ORIENTED_EDGE('',*,*,#13765,.F.);
#19010=ORIENTED_EDGE('',*,*,#13766,.F.);
#19011=ORIENTED_EDGE('',*,*,#13767,.F.);
#19012=ORIENTED_EDGE('',*,*,#13764,.F.);
#19013=ORIENTED_EDGE('',*,*,#13761,.F.);
#19014=ORIENTED_EDGE('',*,*,#13768,.F.);
#19015=ORIENTED_EDGE('',*,*,#13769,.T.);
#19016=ORIENTED_EDGE('',*,*,#13770,.T.);
#19017=ORIENTED_EDGE('',*,*,#13771,.F.);
#19018=ORIENTED_EDGE('',*,*,#13770,.F.);
#19019=ORIENTED_EDGE('',*,*,#13772,.T.);
#19020=ORIENTED_EDGE('',*,*,#13773,.F.);
#19021=ORIENTED_EDGE('',*,*,#13774,.F.);
#19022=ORIENTED_EDGE('',*,*,#13775,.F.);
#19023=ORIENTED_EDGE('',*,*,#13772,.F.);
#19024=ORIENTED_EDGE('',*,*,#13769,.F.);
#19025=ORIENTED_EDGE('',*,*,#13776,.F.);
#19026=ORIENTED_EDGE('',*,*,#13777,.T.);
#19027=ORIENTED_EDGE('',*,*,#13778,.T.);
#19028=ORIENTED_EDGE('',*,*,#13779,.F.);
#19029=ORIENTED_EDGE('',*,*,#13778,.F.);
#19030=ORIENTED_EDGE('',*,*,#13780,.T.);
#19031=ORIENTED_EDGE('',*,*,#13781,.F.);
#19032=ORIENTED_EDGE('',*,*,#13782,.F.);
#19033=ORIENTED_EDGE('',*,*,#13783,.F.);
#19034=ORIENTED_EDGE('',*,*,#13780,.F.);
#19035=ORIENTED_EDGE('',*,*,#13777,.F.);
#19036=ORIENTED_EDGE('',*,*,#13784,.F.);
#19037=ORIENTED_EDGE('',*,*,#13785,.T.);
#19038=ORIENTED_EDGE('',*,*,#13786,.T.);
#19039=ORIENTED_EDGE('',*,*,#13787,.F.);
#19040=ORIENTED_EDGE('',*,*,#13786,.F.);
#19041=ORIENTED_EDGE('',*,*,#13788,.T.);
#19042=ORIENTED_EDGE('',*,*,#13789,.F.);
#19043=ORIENTED_EDGE('',*,*,#13790,.F.);
#19044=ORIENTED_EDGE('',*,*,#13791,.F.);
#19045=ORIENTED_EDGE('',*,*,#13788,.F.);
#19046=ORIENTED_EDGE('',*,*,#13785,.F.);
#19047=ORIENTED_EDGE('',*,*,#13517,.T.);
#19048=ORIENTED_EDGE('',*,*,#13511,.T.);
#19049=ORIENTED_EDGE('',*,*,#13514,.T.);
#19050=ORIENTED_EDGE('',*,*,#13792,.F.);
#19051=ORIENTED_EDGE('',*,*,#13525,.T.);
#19052=ORIENTED_EDGE('',*,*,#13519,.T.);
#19053=ORIENTED_EDGE('',*,*,#13522,.T.);
#19054=ORIENTED_EDGE('',*,*,#13793,.F.);
#19055=ORIENTED_EDGE('',*,*,#13533,.T.);
#19056=ORIENTED_EDGE('',*,*,#13527,.T.);
#19057=ORIENTED_EDGE('',*,*,#13530,.T.);
#19058=ORIENTED_EDGE('',*,*,#13794,.F.);
#19059=ORIENTED_EDGE('',*,*,#13541,.T.);
#19060=ORIENTED_EDGE('',*,*,#13535,.T.);
#19061=ORIENTED_EDGE('',*,*,#13538,.T.);
#19062=ORIENTED_EDGE('',*,*,#13795,.F.);
#19063=ORIENTED_EDGE('',*,*,#13549,.T.);
#19064=ORIENTED_EDGE('',*,*,#13543,.T.);
#19065=ORIENTED_EDGE('',*,*,#13546,.T.);
#19066=ORIENTED_EDGE('',*,*,#13796,.F.);
#19067=ORIENTED_EDGE('',*,*,#13557,.T.);
#19068=ORIENTED_EDGE('',*,*,#13551,.T.);
#19069=ORIENTED_EDGE('',*,*,#13554,.T.);
#19070=ORIENTED_EDGE('',*,*,#13797,.F.);
#19071=ORIENTED_EDGE('',*,*,#13565,.T.);
#19072=ORIENTED_EDGE('',*,*,#13559,.T.);
#19073=ORIENTED_EDGE('',*,*,#13562,.T.);
#19074=ORIENTED_EDGE('',*,*,#13798,.F.);
#19075=ORIENTED_EDGE('',*,*,#13573,.T.);
#19076=ORIENTED_EDGE('',*,*,#13567,.T.);
#19077=ORIENTED_EDGE('',*,*,#13570,.T.);
#19078=ORIENTED_EDGE('',*,*,#13799,.F.);
#19079=ORIENTED_EDGE('',*,*,#13581,.T.);
#19080=ORIENTED_EDGE('',*,*,#13575,.T.);
#19081=ORIENTED_EDGE('',*,*,#13578,.T.);
#19082=ORIENTED_EDGE('',*,*,#13800,.F.);
#19083=ORIENTED_EDGE('',*,*,#13589,.T.);
#19084=ORIENTED_EDGE('',*,*,#13583,.T.);
#19085=ORIENTED_EDGE('',*,*,#13586,.T.);
#19086=ORIENTED_EDGE('',*,*,#13801,.F.);
#19087=ORIENTED_EDGE('',*,*,#13597,.T.);
#19088=ORIENTED_EDGE('',*,*,#13591,.T.);
#19089=ORIENTED_EDGE('',*,*,#13594,.T.);
#19090=ORIENTED_EDGE('',*,*,#13802,.F.);
#19091=ORIENTED_EDGE('',*,*,#13605,.T.);
#19092=ORIENTED_EDGE('',*,*,#13599,.T.);
#19093=ORIENTED_EDGE('',*,*,#13602,.T.);
#19094=ORIENTED_EDGE('',*,*,#13803,.F.);
#19095=ORIENTED_EDGE('',*,*,#13613,.T.);
#19096=ORIENTED_EDGE('',*,*,#13607,.T.);
#19097=ORIENTED_EDGE('',*,*,#13610,.T.);
#19098=ORIENTED_EDGE('',*,*,#13804,.F.);
#19099=ORIENTED_EDGE('',*,*,#13621,.T.);
#19100=ORIENTED_EDGE('',*,*,#13615,.T.);
#19101=ORIENTED_EDGE('',*,*,#13618,.T.);
#19102=ORIENTED_EDGE('',*,*,#13805,.F.);
#19103=ORIENTED_EDGE('',*,*,#13629,.T.);
#19104=ORIENTED_EDGE('',*,*,#13623,.T.);
#19105=ORIENTED_EDGE('',*,*,#13626,.T.);
#19106=ORIENTED_EDGE('',*,*,#13806,.F.);
#19107=ORIENTED_EDGE('',*,*,#13637,.T.);
#19108=ORIENTED_EDGE('',*,*,#13631,.T.);
#19109=ORIENTED_EDGE('',*,*,#13634,.T.);
#19110=ORIENTED_EDGE('',*,*,#13807,.F.);
#19111=ORIENTED_EDGE('',*,*,#13645,.T.);
#19112=ORIENTED_EDGE('',*,*,#13639,.T.);
#19113=ORIENTED_EDGE('',*,*,#13642,.T.);
#19114=ORIENTED_EDGE('',*,*,#13808,.F.);
#19115=ORIENTED_EDGE('',*,*,#13654,.T.);
#19116=ORIENTED_EDGE('',*,*,#13647,.T.);
#19117=ORIENTED_EDGE('',*,*,#13809,.T.);
#19118=ORIENTED_EDGE('',*,*,#13810,.T.);
#19119=ORIENTED_EDGE('',*,*,#13809,.F.);
#19120=ORIENTED_EDGE('',*,*,#13650,.T.);
#19121=ORIENTED_EDGE('',*,*,#13651,.T.);
#19122=ORIENTED_EDGE('',*,*,#13811,.F.);
#19123=ORIENTED_EDGE('',*,*,#13662,.T.);
#19124=ORIENTED_EDGE('',*,*,#13656,.T.);
#19125=ORIENTED_EDGE('',*,*,#13659,.T.);
#19126=ORIENTED_EDGE('',*,*,#13812,.F.);
#19127=ORIENTED_EDGE('',*,*,#13670,.T.);
#19128=ORIENTED_EDGE('',*,*,#13664,.T.);
#19129=ORIENTED_EDGE('',*,*,#13667,.T.);
#19130=ORIENTED_EDGE('',*,*,#13813,.F.);
#19131=ORIENTED_EDGE('',*,*,#13678,.T.);
#19132=ORIENTED_EDGE('',*,*,#13672,.T.);
#19133=ORIENTED_EDGE('',*,*,#13675,.T.);
#19134=ORIENTED_EDGE('',*,*,#13814,.F.);
#19135=ORIENTED_EDGE('',*,*,#13686,.T.);
#19136=ORIENTED_EDGE('',*,*,#13680,.T.);
#19137=ORIENTED_EDGE('',*,*,#13683,.T.);
#19138=ORIENTED_EDGE('',*,*,#13815,.F.);
#19139=ORIENTED_EDGE('',*,*,#13694,.T.);
#19140=ORIENTED_EDGE('',*,*,#13688,.T.);
#19141=ORIENTED_EDGE('',*,*,#13691,.T.);
#19142=ORIENTED_EDGE('',*,*,#13816,.F.);
#19143=ORIENTED_EDGE('',*,*,#13702,.T.);
#19144=ORIENTED_EDGE('',*,*,#13696,.T.);
#19145=ORIENTED_EDGE('',*,*,#13699,.T.);
#19146=ORIENTED_EDGE('',*,*,#13817,.F.);
#19147=ORIENTED_EDGE('',*,*,#13710,.T.);
#19148=ORIENTED_EDGE('',*,*,#13704,.T.);
#19149=ORIENTED_EDGE('',*,*,#13707,.T.);
#19150=ORIENTED_EDGE('',*,*,#13818,.F.);
#19151=ORIENTED_EDGE('',*,*,#13718,.T.);
#19152=ORIENTED_EDGE('',*,*,#13712,.T.);
#19153=ORIENTED_EDGE('',*,*,#13715,.T.);
#19154=ORIENTED_EDGE('',*,*,#13819,.F.);
#19155=ORIENTED_EDGE('',*,*,#13726,.T.);
#19156=ORIENTED_EDGE('',*,*,#13720,.T.);
#19157=ORIENTED_EDGE('',*,*,#13723,.T.);
#19158=ORIENTED_EDGE('',*,*,#13820,.F.);
#19159=ORIENTED_EDGE('',*,*,#13734,.T.);
#19160=ORIENTED_EDGE('',*,*,#13728,.T.);
#19161=ORIENTED_EDGE('',*,*,#13731,.T.);
#19162=ORIENTED_EDGE('',*,*,#13821,.F.);
#19163=ORIENTED_EDGE('',*,*,#13742,.T.);
#19164=ORIENTED_EDGE('',*,*,#13736,.T.);
#19165=ORIENTED_EDGE('',*,*,#13739,.T.);
#19166=ORIENTED_EDGE('',*,*,#13822,.F.);
#19167=ORIENTED_EDGE('',*,*,#13750,.T.);
#19168=ORIENTED_EDGE('',*,*,#13744,.T.);
#19169=ORIENTED_EDGE('',*,*,#13747,.T.);
#19170=ORIENTED_EDGE('',*,*,#13823,.F.);
#19171=ORIENTED_EDGE('',*,*,#13758,.T.);
#19172=ORIENTED_EDGE('',*,*,#13752,.T.);
#19173=ORIENTED_EDGE('',*,*,#13755,.T.);
#19174=ORIENTED_EDGE('',*,*,#13824,.F.);
#19175=ORIENTED_EDGE('',*,*,#13766,.T.);
#19176=ORIENTED_EDGE('',*,*,#13760,.T.);
#19177=ORIENTED_EDGE('',*,*,#13763,.T.);
#19178=ORIENTED_EDGE('',*,*,#13825,.F.);
#19179=ORIENTED_EDGE('',*,*,#13774,.T.);
#19180=ORIENTED_EDGE('',*,*,#13768,.T.);
#19181=ORIENTED_EDGE('',*,*,#13771,.T.);
#19182=ORIENTED_EDGE('',*,*,#13826,.F.);
#19183=ORIENTED_EDGE('',*,*,#13782,.T.);
#19184=ORIENTED_EDGE('',*,*,#13776,.T.);
#19185=ORIENTED_EDGE('',*,*,#13779,.T.);
#19186=ORIENTED_EDGE('',*,*,#13827,.F.);
#19187=ORIENTED_EDGE('',*,*,#13790,.T.);
#19188=ORIENTED_EDGE('',*,*,#13784,.T.);
#19189=ORIENTED_EDGE('',*,*,#13787,.T.);
#19190=ORIENTED_EDGE('',*,*,#13828,.F.);
#19191=ORIENTED_EDGE('',*,*,#13829,.T.);
#19192=ORIENTED_EDGE('',*,*,#13830,.T.);
#19193=ORIENTED_EDGE('',*,*,#13831,.T.);
#19194=ORIENTED_EDGE('',*,*,#13832,.F.);
#19195=ORIENTED_EDGE('',*,*,#13831,.F.);
#19196=ORIENTED_EDGE('',*,*,#13833,.F.);
#19197=ORIENTED_EDGE('',*,*,#13834,.T.);
#19198=ORIENTED_EDGE('',*,*,#13835,.F.);
#19199=ORIENTED_EDGE('',*,*,#13836,.F.);
#19200=ORIENTED_EDGE('',*,*,#13834,.F.);
#19201=ORIENTED_EDGE('',*,*,#13837,.F.);
#19202=ORIENTED_EDGE('',*,*,#13829,.F.);
#19203=ORIENTED_EDGE('',*,*,#13830,.F.);
#19204=ORIENTED_EDGE('',*,*,#13837,.T.);
#19205=ORIENTED_EDGE('',*,*,#13833,.T.);
#19206=ORIENTED_EDGE('',*,*,#13838,.F.);
#19207=ORIENTED_EDGE('',*,*,#13839,.T.);
#19208=ORIENTED_EDGE('',*,*,#13655,.T.);
#19209=ORIENTED_EDGE('',*,*,#13808,.T.);
#19210=ORIENTED_EDGE('',*,*,#13644,.T.);
#19211=ORIENTED_EDGE('',*,*,#13646,.T.);
#19212=ORIENTED_EDGE('',*,*,#13807,.T.);
#19213=ORIENTED_EDGE('',*,*,#13636,.T.);
#19214=ORIENTED_EDGE('',*,*,#13638,.T.);
#19215=ORIENTED_EDGE('',*,*,#13806,.T.);
#19216=ORIENTED_EDGE('',*,*,#13628,.T.);
#19217=ORIENTED_EDGE('',*,*,#13630,.T.);
#19218=ORIENTED_EDGE('',*,*,#13805,.T.);
#19219=ORIENTED_EDGE('',*,*,#13620,.T.);
#19220=ORIENTED_EDGE('',*,*,#13622,.T.);
#19221=ORIENTED_EDGE('',*,*,#13804,.T.);
#19222=ORIENTED_EDGE('',*,*,#13612,.T.);
#19223=ORIENTED_EDGE('',*,*,#13614,.T.);
#19224=ORIENTED_EDGE('',*,*,#13803,.T.);
#19225=ORIENTED_EDGE('',*,*,#13604,.T.);
#19226=ORIENTED_EDGE('',*,*,#13606,.T.);
#19227=ORIENTED_EDGE('',*,*,#13802,.T.);
#19228=ORIENTED_EDGE('',*,*,#13596,.T.);
#19229=ORIENTED_EDGE('',*,*,#13598,.T.);
#19230=ORIENTED_EDGE('',*,*,#13801,.T.);
#19231=ORIENTED_EDGE('',*,*,#13588,.T.);
#19232=ORIENTED_EDGE('',*,*,#13590,.T.);
#19233=ORIENTED_EDGE('',*,*,#13800,.T.);
#19234=ORIENTED_EDGE('',*,*,#13580,.T.);
#19235=ORIENTED_EDGE('',*,*,#13582,.T.);
#19236=ORIENTED_EDGE('',*,*,#13799,.T.);
#19237=ORIENTED_EDGE('',*,*,#13572,.T.);
#19238=ORIENTED_EDGE('',*,*,#13574,.T.);
#19239=ORIENTED_EDGE('',*,*,#13798,.T.);
#19240=ORIENTED_EDGE('',*,*,#13564,.T.);
#19241=ORIENTED_EDGE('',*,*,#13566,.T.);
#19242=ORIENTED_EDGE('',*,*,#13797,.T.);
#19243=ORIENTED_EDGE('',*,*,#13556,.T.);
#19244=ORIENTED_EDGE('',*,*,#13558,.T.);
#19245=ORIENTED_EDGE('',*,*,#13796,.T.);
#19246=ORIENTED_EDGE('',*,*,#13548,.T.);
#19247=ORIENTED_EDGE('',*,*,#13550,.T.);
#19248=ORIENTED_EDGE('',*,*,#13795,.T.);
#19249=ORIENTED_EDGE('',*,*,#13540,.T.);
#19250=ORIENTED_EDGE('',*,*,#13542,.T.);
#19251=ORIENTED_EDGE('',*,*,#13794,.T.);
#19252=ORIENTED_EDGE('',*,*,#13532,.T.);
#19253=ORIENTED_EDGE('',*,*,#13534,.T.);
#19254=ORIENTED_EDGE('',*,*,#13793,.T.);
#19255=ORIENTED_EDGE('',*,*,#13524,.T.);
#19256=ORIENTED_EDGE('',*,*,#13526,.T.);
#19257=ORIENTED_EDGE('',*,*,#13792,.T.);
#19258=ORIENTED_EDGE('',*,*,#13516,.T.);
#19259=ORIENTED_EDGE('',*,*,#13518,.T.);
#19260=ORIENTED_EDGE('',*,*,#13832,.T.);
#19261=ORIENTED_EDGE('',*,*,#13835,.T.);
#19262=ORIENTED_EDGE('',*,*,#13836,.T.);
#19263=ORIENTED_EDGE('',*,*,#13828,.T.);
#19264=ORIENTED_EDGE('',*,*,#13789,.T.);
#19265=ORIENTED_EDGE('',*,*,#13791,.T.);
#19266=ORIENTED_EDGE('',*,*,#13827,.T.);
#19267=ORIENTED_EDGE('',*,*,#13781,.T.);
#19268=ORIENTED_EDGE('',*,*,#13783,.T.);
#19269=ORIENTED_EDGE('',*,*,#13826,.T.);
#19270=ORIENTED_EDGE('',*,*,#13773,.T.);
#19271=ORIENTED_EDGE('',*,*,#13775,.T.);
#19272=ORIENTED_EDGE('',*,*,#13825,.T.);
#19273=ORIENTED_EDGE('',*,*,#13765,.T.);
#19274=ORIENTED_EDGE('',*,*,#13767,.T.);
#19275=ORIENTED_EDGE('',*,*,#13824,.T.);
#19276=ORIENTED_EDGE('',*,*,#13757,.T.);
#19277=ORIENTED_EDGE('',*,*,#13759,.T.);
#19278=ORIENTED_EDGE('',*,*,#13823,.T.);
#19279=ORIENTED_EDGE('',*,*,#13749,.T.);
#19280=ORIENTED_EDGE('',*,*,#13751,.T.);
#19281=ORIENTED_EDGE('',*,*,#13822,.T.);
#19282=ORIENTED_EDGE('',*,*,#13741,.T.);
#19283=ORIENTED_EDGE('',*,*,#13743,.T.);
#19284=ORIENTED_EDGE('',*,*,#13821,.T.);
#19285=ORIENTED_EDGE('',*,*,#13733,.T.);
#19286=ORIENTED_EDGE('',*,*,#13735,.T.);
#19287=ORIENTED_EDGE('',*,*,#13820,.T.);
#19288=ORIENTED_EDGE('',*,*,#13725,.T.);
#19289=ORIENTED_EDGE('',*,*,#13727,.T.);
#19290=ORIENTED_EDGE('',*,*,#13819,.T.);
#19291=ORIENTED_EDGE('',*,*,#13717,.T.);
#19292=ORIENTED_EDGE('',*,*,#13719,.T.);
#19293=ORIENTED_EDGE('',*,*,#13818,.T.);
#19294=ORIENTED_EDGE('',*,*,#13709,.T.);
#19295=ORIENTED_EDGE('',*,*,#13711,.T.);
#19296=ORIENTED_EDGE('',*,*,#13817,.T.);
#19297=ORIENTED_EDGE('',*,*,#13701,.T.);
#19298=ORIENTED_EDGE('',*,*,#13703,.T.);
#19299=ORIENTED_EDGE('',*,*,#13816,.T.);
#19300=ORIENTED_EDGE('',*,*,#13693,.T.);
#19301=ORIENTED_EDGE('',*,*,#13695,.T.);
#19302=ORIENTED_EDGE('',*,*,#13815,.T.);
#19303=ORIENTED_EDGE('',*,*,#13685,.T.);
#19304=ORIENTED_EDGE('',*,*,#13687,.T.);
#19305=ORIENTED_EDGE('',*,*,#13814,.T.);
#19306=ORIENTED_EDGE('',*,*,#13677,.T.);
#19307=ORIENTED_EDGE('',*,*,#13679,.T.);
#19308=ORIENTED_EDGE('',*,*,#13813,.T.);
#19309=ORIENTED_EDGE('',*,*,#13669,.T.);
#19310=ORIENTED_EDGE('',*,*,#13671,.T.);
#19311=ORIENTED_EDGE('',*,*,#13812,.T.);
#19312=ORIENTED_EDGE('',*,*,#13661,.T.);
#19313=ORIENTED_EDGE('',*,*,#13663,.T.);
#19314=ORIENTED_EDGE('',*,*,#13811,.T.);
#19315=ORIENTED_EDGE('',*,*,#13653,.T.);
#19316=ORIENTED_EDGE('',*,*,#13839,.F.);
#19317=ORIENTED_EDGE('',*,*,#13840,.T.);
#19318=ORIENTED_EDGE('',*,*,#13841,.F.);
#19319=ORIENTED_EDGE('',*,*,#13840,.F.);
#19320=ORIENTED_EDGE('',*,*,#13842,.F.);
#19321=ORIENTED_EDGE('',*,*,#13843,.T.);
#19322=ORIENTED_EDGE('',*,*,#13844,.T.);
#19323=ORIENTED_EDGE('',*,*,#13845,.F.);
#19324=ORIENTED_EDGE('',*,*,#13846,.F.);
#19325=ORIENTED_EDGE('',*,*,#13847,.T.);
#19326=ORIENTED_EDGE('',*,*,#13848,.T.);
#19327=ORIENTED_EDGE('',*,*,#13843,.F.);
#19328=ORIENTED_EDGE('',*,*,#13849,.F.);
#19329=ORIENTED_EDGE('',*,*,#13850,.T.);
#19330=ORIENTED_EDGE('',*,*,#13851,.T.);
#19331=ORIENTED_EDGE('',*,*,#13847,.F.);
#19332=ORIENTED_EDGE('',*,*,#13852,.F.);
#19333=ORIENTED_EDGE('',*,*,#13853,.T.);
#19334=ORIENTED_EDGE('',*,*,#13854,.T.);
#19335=ORIENTED_EDGE('',*,*,#13850,.F.);
#19336=ORIENTED_EDGE('',*,*,#13855,.F.);
#19337=ORIENTED_EDGE('',*,*,#13856,.T.);
#19338=ORIENTED_EDGE('',*,*,#13857,.T.);
#19339=ORIENTED_EDGE('',*,*,#13853,.F.);
#19340=ORIENTED_EDGE('',*,*,#13858,.F.);
#19341=ORIENTED_EDGE('',*,*,#13845,.T.);
#19342=ORIENTED_EDGE('',*,*,#13859,.T.);
#19343=ORIENTED_EDGE('',*,*,#13856,.F.);
#19344=ORIENTED_EDGE('',*,*,#13859,.F.);
#19345=ORIENTED_EDGE('',*,*,#13844,.F.);
#19346=ORIENTED_EDGE('',*,*,#13848,.F.);
#19347=ORIENTED_EDGE('',*,*,#13851,.F.);
#19348=ORIENTED_EDGE('',*,*,#13854,.F.);
#19349=ORIENTED_EDGE('',*,*,#13857,.F.);
#19350=ORIENTED_EDGE('',*,*,#13841,.T.);
#19351=ORIENTED_EDGE('',*,*,#13860,.F.);
#19352=ORIENTED_EDGE('',*,*,#13412,.F.);
#19353=ORIENTED_EDGE('',*,*,#13861,.T.);
#19354=ORIENTED_EDGE('',*,*,#13860,.T.);
#19355=ORIENTED_EDGE('',*,*,#13861,.F.);
#19356=ORIENTED_EDGE('',*,*,#13451,.T.);
#19357=ORIENTED_EDGE('',*,*,#13504,.T.);
#19358=ORIENTED_EDGE('',*,*,#13862,.F.);
#19359=ORIENTED_EDGE('',*,*,#13510,.T.);
#19360=ORIENTED_EDGE('',*,*,#13863,.F.);
#19361=ORIENTED_EDGE('',*,*,#13864,.T.);
#19362=ORIENTED_EDGE('',*,*,#13501,.T.);
#19363=ORIENTED_EDGE('',*,*,#13862,.T.);
#19364=ORIENTED_EDGE('',*,*,#13502,.T.);
#19365=ORIENTED_EDGE('',*,*,#13864,.F.);
#19366=ORIENTED_EDGE('',*,*,#13810,.F.);
#19367=ORIENTED_EDGE('',*,*,#13863,.T.);
#19368=ORIENTED_EDGE('',*,*,#13838,.T.);
#19369=ORIENTED_EDGE('',*,*,#13842,.T.);
#19370=ORIENTED_EDGE('',*,*,#13858,.T.);
#19371=ORIENTED_EDGE('',*,*,#13855,.T.);
#19372=ORIENTED_EDGE('',*,*,#13852,.T.);
#19373=ORIENTED_EDGE('',*,*,#13849,.T.);
#19374=ORIENTED_EDGE('',*,*,#13846,.T.);
#21963=CONICAL_SURFACE('',#25018,0.2675,0.78539816339745);
#21964=CONICAL_SURFACE('',#25020,0.0577350269189626,1.00599363799961);
#21965=CONICAL_SURFACE('',#25031,0.132,0.785398163397448);
#21966=CONICAL_SURFACE('',#25034,0.155,0.785398163397449);
#22733=ADVANCED_FACE('',(#2994),#1085,.T.);
#22734=ADVANCED_FACE('',(#2995),#1086,.T.);
#22735=ADVANCED_FACE('',(#2996),#1087,.T.);
#22736=ADVANCED_FACE('',(#2997),#1088,.T.);
#22737=ADVANCED_FACE('',(#2998),#1089,.T.);
#22738=ADVANCED_FACE('',(#2999),#1090,.T.);
#22739=ADVANCED_FACE('',(#3000),#1091,.T.);
#22740=ADVANCED_FACE('',(#3001),#1092,.T.);
#22741=ADVANCED_FACE('',(#3002),#1093,.T.);
#22742=ADVANCED_FACE('',(#3003),#1094,.T.);
#22743=ADVANCED_FACE('',(#3004),#1095,.T.);
#22744=ADVANCED_FACE('',(#3005),#1096,.T.);
#22745=ADVANCED_FACE('',(#3006),#1097,.T.);
#22746=ADVANCED_FACE('',(#3007),#1098,.T.);
#22747=ADVANCED_FACE('',(#3008),#1099,.T.);
#22748=ADVANCED_FACE('',(#3009),#1100,.T.);
#22749=ADVANCED_FACE('',(#3010),#1101,.T.);
#22750=ADVANCED_FACE('',(#3011),#1102,.T.);
#22751=ADVANCED_FACE('',(#3012),#1103,.T.);
#22752=ADVANCED_FACE('',(#3013),#1104,.T.);
#22753=ADVANCED_FACE('',(#3014),#1105,.T.);
#22754=ADVANCED_FACE('',(#3015),#1106,.T.);
#22755=ADVANCED_FACE('',(#3016),#1107,.T.);
#22756=ADVANCED_FACE('',(#3017),#1108,.T.);
#22757=ADVANCED_FACE('',(#3018),#1109,.T.);
#22758=ADVANCED_FACE('',(#3019),#1110,.T.);
#22759=ADVANCED_FACE('',(#3020),#1111,.T.);
#22760=ADVANCED_FACE('',(#3021),#1112,.T.);
#22761=ADVANCED_FACE('',(#3022),#1113,.T.);
#22762=ADVANCED_FACE('',(#3023),#1876,.F.);
#22763=ADVANCED_FACE('',(#3024),#367,.F.);
#22764=ADVANCED_FACE('',(#3025),#1877,.T.);
#22765=ADVANCED_FACE('',(#3026),#1114,.T.);
#22766=ADVANCED_FACE('',(#3027),#368,.F.);
#22767=ADVANCED_FACE('',(#3028),#1878,.T.);
#22768=ADVANCED_FACE('',(#3029),#1879,.F.);
#22769=ADVANCED_FACE('',(#3030),#1880,.F.);
#22770=ADVANCED_FACE('',(#3031),#1881,.T.);
#22771=ADVANCED_FACE('',(#3032),#1882,.F.);
#22772=ADVANCED_FACE('',(#3033),#1883,.F.);
#22773=ADVANCED_FACE('',(#3034),#1884,.T.);
#22774=ADVANCED_FACE('',(#3035),#1885,.F.);
#22775=ADVANCED_FACE('',(#3036),#1886,.F.);
#22776=ADVANCED_FACE('',(#3037),#1887,.T.);
#22777=ADVANCED_FACE('',(#3038),#1888,.F.);
#22778=ADVANCED_FACE('',(#3039),#1889,.F.);
#22779=ADVANCED_FACE('',(#3040),#1890,.T.);
#22780=ADVANCED_FACE('',(#3041),#1891,.F.);
#22781=ADVANCED_FACE('',(#3042),#1892,.F.);
#22782=ADVANCED_FACE('',(#3043),#1893,.T.);
#22783=ADVANCED_FACE('',(#3044),#1894,.F.);
#22784=ADVANCED_FACE('',(#3045),#1895,.F.);
#22785=ADVANCED_FACE('',(#3046),#1896,.T.);
#22786=ADVANCED_FACE('',(#3047),#1897,.F.);
#22787=ADVANCED_FACE('',(#3048),#1898,.F.);
#22788=ADVANCED_FACE('',(#3049),#1899,.T.);
#22789=ADVANCED_FACE('',(#3050),#1900,.F.);
#22790=ADVANCED_FACE('',(#3051),#1901,.F.);
#22791=ADVANCED_FACE('',(#3052),#1902,.T.);
#22792=ADVANCED_FACE('',(#3053),#1903,.F.);
#22793=ADVANCED_FACE('',(#3054),#1904,.F.);
#22794=ADVANCED_FACE('',(#3055),#1905,.T.);
#22795=ADVANCED_FACE('',(#3056),#1906,.F.);
#22796=ADVANCED_FACE('',(#3057),#1907,.F.);
#22797=ADVANCED_FACE('',(#3058),#1908,.T.);
#22798=ADVANCED_FACE('',(#3059),#1909,.F.);
#22799=ADVANCED_FACE('',(#3060),#1910,.F.);
#22800=ADVANCED_FACE('',(#3061),#1911,.T.);
#22801=ADVANCED_FACE('',(#3062),#1912,.F.);
#22802=ADVANCED_FACE('',(#3063),#1913,.F.);
#22803=ADVANCED_FACE('',(#3064),#1914,.T.);
#22804=ADVANCED_FACE('',(#3065),#1915,.F.);
#22805=ADVANCED_FACE('',(#3066),#1916,.F.);
#22806=ADVANCED_FACE('',(#3067),#1917,.T.);
#22807=ADVANCED_FACE('',(#3068),#1918,.F.);
#22808=ADVANCED_FACE('',(#3069),#1919,.F.);
#22809=ADVANCED_FACE('',(#3070),#1920,.T.);
#22810=ADVANCED_FACE('',(#3071),#1921,.F.);
#22811=ADVANCED_FACE('',(#3072),#1922,.F.);
#22812=ADVANCED_FACE('',(#3073),#1923,.T.);
#22813=ADVANCED_FACE('',(#3074),#1924,.F.);
#22814=ADVANCED_FACE('',(#3075),#1925,.F.);
#22815=ADVANCED_FACE('',(#3076),#1926,.T.);
#22816=ADVANCED_FACE('',(#3077),#1927,.F.);
#22817=ADVANCED_FACE('',(#3078),#1928,.F.);
#22818=ADVANCED_FACE('',(#3079),#1929,.T.);
#22819=ADVANCED_FACE('',(#3080),#1930,.F.);
#22820=ADVANCED_FACE('',(#3081),#1931,.F.);
#22821=ADVANCED_FACE('',(#3082),#1932,.T.);
#22822=ADVANCED_FACE('',(#3083),#1933,.F.);
#22823=ADVANCED_FACE('',(#3084),#1934,.F.);
#22824=ADVANCED_FACE('',(#3085),#1935,.T.);
#22825=ADVANCED_FACE('',(#3086),#1936,.F.);
#22826=ADVANCED_FACE('',(#3087),#1937,.F.);
#22827=ADVANCED_FACE('',(#3088),#1938,.T.);
#22828=ADVANCED_FACE('',(#3089),#1939,.F.);
#22829=ADVANCED_FACE('',(#3090),#1940,.F.);
#22830=ADVANCED_FACE('',(#3091),#1941,.T.);
#22831=ADVANCED_FACE('',(#3092),#1942,.F.);
#22832=ADVANCED_FACE('',(#3093),#1943,.F.);
#22833=ADVANCED_FACE('',(#3094),#1944,.T.);
#22834=ADVANCED_FACE('',(#3095),#1945,.F.);
#22835=ADVANCED_FACE('',(#3096),#1946,.F.);
#22836=ADVANCED_FACE('',(#3097),#1947,.T.);
#22837=ADVANCED_FACE('',(#3098),#1948,.F.);
#22838=ADVANCED_FACE('',(#3099),#1949,.F.);
#22839=ADVANCED_FACE('',(#3100),#1950,.T.);
#22840=ADVANCED_FACE('',(#3101),#1951,.F.);
#22841=ADVANCED_FACE('',(#3102),#1952,.F.);
#22842=ADVANCED_FACE('',(#3103),#1953,.T.);
#22843=ADVANCED_FACE('',(#3104),#1954,.F.);
#22844=ADVANCED_FACE('',(#3105),#1955,.F.);
#22845=ADVANCED_FACE('',(#3106),#1956,.T.);
#22846=ADVANCED_FACE('',(#3107),#1957,.F.);
#22847=ADVANCED_FACE('',(#3108),#1958,.F.);
#22848=ADVANCED_FACE('',(#3109),#1959,.T.);
#22849=ADVANCED_FACE('',(#3110),#1960,.F.);
#22850=ADVANCED_FACE('',(#3111),#1961,.F.);
#22851=ADVANCED_FACE('',(#3112),#1962,.T.);
#22852=ADVANCED_FACE('',(#3113),#1963,.F.);
#22853=ADVANCED_FACE('',(#3114),#1964,.F.);
#22854=ADVANCED_FACE('',(#3115),#1965,.T.);
#22855=ADVANCED_FACE('',(#3116),#1966,.F.);
#22856=ADVANCED_FACE('',(#3117),#1967,.F.);
#22857=ADVANCED_FACE('',(#3118),#1968,.T.);
#22858=ADVANCED_FACE('',(#3119),#1969,.F.);
#22859=ADVANCED_FACE('',(#3120),#1970,.F.);
#22860=ADVANCED_FACE('',(#3121),#1971,.T.);
#22861=ADVANCED_FACE('',(#3122),#1972,.F.);
#22862=ADVANCED_FACE('',(#3123),#1973,.F.);
#22863=ADVANCED_FACE('',(#3124),#1974,.T.);
#22864=ADVANCED_FACE('',(#3125),#1975,.F.);
#22865=ADVANCED_FACE('',(#3126),#1976,.F.);
#22866=ADVANCED_FACE('',(#3127),#1977,.T.);
#22867=ADVANCED_FACE('',(#3128),#1978,.F.);
#22868=ADVANCED_FACE('',(#3129),#1979,.F.);
#22869=ADVANCED_FACE('',(#3130),#1980,.T.);
#22870=ADVANCED_FACE('',(#3131),#1981,.F.);
#22871=ADVANCED_FACE('',(#3132),#1982,.F.);
#22872=ADVANCED_FACE('',(#3133),#1115,.T.);
#22873=ADVANCED_FACE('',(#3134),#1983,.F.);
#22874=ADVANCED_FACE('',(#3135),#1984,.F.);
#22875=ADVANCED_FACE('',(#3136),#1985,.T.);
#22876=ADVANCED_FACE('',(#3137),#21963,.T.);
#22877=ADVANCED_FACE('',(#3138),#21964,.F.);
#22878=ADVANCED_FACE('',(#3139),#1986,.F.);
#22879=ADVANCED_FACE('',(#3140),#1987,.F.);
#22880=ADVANCED_FACE('',(#3141),#1988,.F.);
#22881=ADVANCED_FACE('',(#3142),#1989,.F.);
#22882=ADVANCED_FACE('',(#3143),#1990,.F.);
#22883=ADVANCED_FACE('',(#3144),#1991,.F.);
#22884=ADVANCED_FACE('',(#3145,#1439),#1992,.F.);
#22885=ADVANCED_FACE('',(#3146),#1993,.T.);
#22886=ADVANCED_FACE('',(#3147),#21965,.T.);
#22887=ADVANCED_FACE('',(#3148),#1116,.T.);
#22888=ADVANCED_FACE('',(#3149),#21966,.T.);
#22889=ADVANCED_FACE('',(#3150,#1440),#1994,.T.);
#22890=ADVANCED_FACE('',(#3151,#1441),#1995,.T.);
#23316=CLOSED_SHELL('',(#22733,#22734,#22735,#22736,#22737,#22738,#22739,
#22740,#22741,#22742,#22743,#22744,#22745,#22746,#22747,#22748,#22749,#22750,
#22751,#22752,#22753,#22754,#22755,#22756,#22757,#22758,#22759,#22760,#22761,
#22762,#22763,#22764,#22765,#22766,#22767,#22768,#22769,#22770,#22771,#22772,
#22773,#22774,#22775,#22776,#22777,#22778,#22779,#22780,#22781,#22782,#22783,
#22784,#22785,#22786,#22787,#22788,#22789,#22790,#22791,#22792,#22793,#22794,
#22795,#22796,#22797,#22798,#22799,#22800,#22801,#22802,#22803,#22804,#22805,
#22806,#22807,#22808,#22809,#22810,#22811,#22812,#22813,#22814,#22815,#22816,
#22817,#22818,#22819,#22820,#22821,#22822,#22823,#22824,#22825,#22826,#22827,
#22828,#22829,#22830,#22831,#22832,#22833,#22834,#22835,#22836,#22837,#22838,
#22839,#22840,#22841,#22842,#22843,#22844,#22845,#22846,#22847,#22848,#22849,
#22850,#22851,#22852,#22853,#22854,#22855,#22856,#22857,#22858,#22859,#22860,
#22861,#22862,#22863,#22864,#22865,#22866,#22867,#22868,#22869,#22870,#22871,
#22872,#22873,#22874,#22875,#22876,#22877,#22878,#22879,#22880,#22881,#22882,
#22883,#22884,#22885,#22886,#22887,#22888,#22889,#22890));
#24795=AXIS2_PLACEMENT_3D('',#38705,#29302,#29303);
#24796=AXIS2_PLACEMENT_3D('',#38706,#29304,#29305);
#24797=AXIS2_PLACEMENT_3D('',#38728,#29307,#29308);
#24798=AXIS2_PLACEMENT_3D('',#38731,#29310,#29311);
#24799=AXIS2_PLACEMENT_3D('',#38733,#29312,#29313);
#24800=AXIS2_PLACEMENT_3D('',#38747,#29314,#29315);
#24801=AXIS2_PLACEMENT_3D('',#38801,#29317,#29318);
#24802=AXIS2_PLACEMENT_3D('',#38849,#29320,#29321);
#24803=AXIS2_PLACEMENT_3D('',#38897,#29323,#29324);
#24804=AXIS2_PLACEMENT_3D('',#38951,#29326,#29327);
#24805=AXIS2_PLACEMENT_3D('',#38999,#29329,#29330);
#24806=AXIS2_PLACEMENT_3D('',#39047,#29332,#29333);
#24807=AXIS2_PLACEMENT_3D('',#39101,#29335,#29336);
#24808=AXIS2_PLACEMENT_3D('',#39149,#29338,#29339);
#24809=AXIS2_PLACEMENT_3D('',#39197,#29341,#29342);
#24810=AXIS2_PLACEMENT_3D('',#39251,#29344,#29345);
#24811=AXIS2_PLACEMENT_3D('',#39299,#29347,#29348);
#24812=AXIS2_PLACEMENT_3D('',#39347,#29350,#29351);
#24813=AXIS2_PLACEMENT_3D('',#39401,#29353,#29354);
#24814=AXIS2_PLACEMENT_3D('',#39413,#29356,#29357);
#24815=AXIS2_PLACEMENT_3D('',#39419,#29358,#29359);
#24816=AXIS2_PLACEMENT_3D('',#39444,#29361,#29362);
#24817=AXIS2_PLACEMENT_3D('',#39469,#29364,#29365);
#24818=AXIS2_PLACEMENT_3D('',#39493,#29367,#29368);
#24819=AXIS2_PLACEMENT_3D('',#39518,#29370,#29371);
#24820=AXIS2_PLACEMENT_3D('',#39543,#29373,#29374);
#24821=AXIS2_PLACEMENT_3D('',#39567,#29376,#29377);
#24822=AXIS2_PLACEMENT_3D('',#39592,#29379,#29380);
#24823=AXIS2_PLACEMENT_3D('',#39617,#29382,#29383);
#24824=AXIS2_PLACEMENT_3D('',#39641,#29385,#29386);
#24825=AXIS2_PLACEMENT_3D('',#39666,#29388,#29389);
#24826=AXIS2_PLACEMENT_3D('',#39691,#29391,#29392);
#24827=AXIS2_PLACEMENT_3D('',#39715,#29394,#29395);
#24828=AXIS2_PLACEMENT_3D('',#39740,#29397,#29398);
#24829=AXIS2_PLACEMENT_3D('',#39765,#29400,#29401);
#24830=AXIS2_PLACEMENT_3D('',#39820,#29402,#29403);
#24831=AXIS2_PLACEMENT_3D('',#39822,#29404,#29405);
#24832=AXIS2_PLACEMENT_3D('',#40340,#29406,#29407);
#24833=AXIS2_PLACEMENT_3D('',#40394,#29408,#29409);
#24834=AXIS2_PLACEMENT_3D('',#40395,#29410,#29411);
#24835=AXIS2_PLACEMENT_3D('',#40804,#29412,#29413);
#24836=AXIS2_PLACEMENT_3D('',#40807,#29414,#29415);
#24837=AXIS2_PLACEMENT_3D('',#40811,#29418,#29419);
#24838=AXIS2_PLACEMENT_3D('',#40819,#29422,#29423);
#24839=AXIS2_PLACEMENT_3D('',#40825,#29425,#29426);
#24840=AXIS2_PLACEMENT_3D('',#40828,#29427,#29428);
#24841=AXIS2_PLACEMENT_3D('',#40832,#29431,#29432);
#24842=AXIS2_PLACEMENT_3D('',#40840,#29435,#29436);
#24843=AXIS2_PLACEMENT_3D('',#40846,#29438,#29439);
#24844=AXIS2_PLACEMENT_3D('',#40849,#29440,#29441);
#24845=AXIS2_PLACEMENT_3D('',#40853,#29444,#29445);
#24846=AXIS2_PLACEMENT_3D('',#40861,#29448,#29449);
#24847=AXIS2_PLACEMENT_3D('',#40867,#29451,#29452);
#24848=AXIS2_PLACEMENT_3D('',#40870,#29453,#29454);
#24849=AXIS2_PLACEMENT_3D('',#40874,#29457,#29458);
#24850=AXIS2_PLACEMENT_3D('',#40882,#29461,#29462);
#24851=AXIS2_PLACEMENT_3D('',#40888,#29464,#29465);
#24852=AXIS2_PLACEMENT_3D('',#40891,#29466,#29467);
#24853=AXIS2_PLACEMENT_3D('',#40895,#29470,#29471);
#24854=AXIS2_PLACEMENT_3D('',#40903,#29474,#29475);
#24855=AXIS2_PLACEMENT_3D('',#40909,#29477,#29478);
#24856=AXIS2_PLACEMENT_3D('',#40912,#29479,#29480);
#24857=AXIS2_PLACEMENT_3D('',#40916,#29483,#29484);
#24858=AXIS2_PLACEMENT_3D('',#40924,#29487,#29488);
#24859=AXIS2_PLACEMENT_3D('',#40930,#29490,#29491);
#24860=AXIS2_PLACEMENT_3D('',#40933,#29492,#29493);
#24861=AXIS2_PLACEMENT_3D('',#40937,#29496,#29497);
#24862=AXIS2_PLACEMENT_3D('',#40945,#29500,#29501);
#24863=AXIS2_PLACEMENT_3D('',#40951,#29503,#29504);
#24864=AXIS2_PLACEMENT_3D('',#40954,#29505,#29506);
#24865=AXIS2_PLACEMENT_3D('',#40958,#29509,#29510);
#24866=AXIS2_PLACEMENT_3D('',#40966,#29513,#29514);
#24867=AXIS2_PLACEMENT_3D('',#40972,#29516,#29517);
#24868=AXIS2_PLACEMENT_3D('',#40975,#29518,#29519);
#24869=AXIS2_PLACEMENT_3D('',#40979,#29522,#29523);
#24870=AXIS2_PLACEMENT_3D('',#40987,#29526,#29527);
#24871=AXIS2_PLACEMENT_3D('',#40993,#29529,#29530);
#24872=AXIS2_PLACEMENT_3D('',#40996,#29531,#29532);
#24873=AXIS2_PLACEMENT_3D('',#41000,#29535,#29536);
#24874=AXIS2_PLACEMENT_3D('',#41008,#29539,#29540);
#24875=AXIS2_PLACEMENT_3D('',#41014,#29542,#29543);
#24876=AXIS2_PLACEMENT_3D('',#41017,#29544,#29545);
#24877=AXIS2_PLACEMENT_3D('',#41021,#29548,#29549);
#24878=AXIS2_PLACEMENT_3D('',#41029,#29552,#29553);
#24879=AXIS2_PLACEMENT_3D('',#41035,#29555,#29556);
#24880=AXIS2_PLACEMENT_3D('',#41038,#29557,#29558);
#24881=AXIS2_PLACEMENT_3D('',#41042,#29561,#29562);
#24882=AXIS2_PLACEMENT_3D('',#41050,#29565,#29566);
#24883=AXIS2_PLACEMENT_3D('',#41056,#29568,#29569);
#24884=AXIS2_PLACEMENT_3D('',#41059,#29570,#29571);
#24885=AXIS2_PLACEMENT_3D('',#41063,#29574,#29575);
#24886=AXIS2_PLACEMENT_3D('',#41071,#29578,#29579);
#24887=AXIS2_PLACEMENT_3D('',#41077,#29581,#29582);
#24888=AXIS2_PLACEMENT_3D('',#41080,#29583,#29584);
#24889=AXIS2_PLACEMENT_3D('',#41084,#29587,#29588);
#24890=AXIS2_PLACEMENT_3D('',#41092,#29591,#29592);
#24891=AXIS2_PLACEMENT_3D('',#41098,#29594,#29595);
#24892=AXIS2_PLACEMENT_3D('',#41101,#29596,#29597);
#24893=AXIS2_PLACEMENT_3D('',#41105,#29600,#29601);
#24894=AXIS2_PLACEMENT_3D('',#41113,#29604,#29605);
#24895=AXIS2_PLACEMENT_3D('',#41119,#29607,#29608);
#24896=AXIS2_PLACEMENT_3D('',#41122,#29609,#29610);
#24897=AXIS2_PLACEMENT_3D('',#41126,#29613,#29614);
#24898=AXIS2_PLACEMENT_3D('',#41134,#29617,#29618);
#24899=AXIS2_PLACEMENT_3D('',#41140,#29620,#29621);
#24900=AXIS2_PLACEMENT_3D('',#41143,#29622,#29623);
#24901=AXIS2_PLACEMENT_3D('',#41147,#29626,#29627);
#24902=AXIS2_PLACEMENT_3D('',#41155,#29630,#29631);
#24903=AXIS2_PLACEMENT_3D('',#41161,#29633,#29634);
#24904=AXIS2_PLACEMENT_3D('',#41164,#29635,#29636);
#24905=AXIS2_PLACEMENT_3D('',#41169,#29639,#29640);
#24906=AXIS2_PLACEMENT_3D('',#41170,#29641,#29642);
#24907=AXIS2_PLACEMENT_3D('',#41178,#29645,#29646);
#24908=AXIS2_PLACEMENT_3D('',#41184,#29648,#29649);
#24909=AXIS2_PLACEMENT_3D('',#41187,#29650,#29651);
#24910=AXIS2_PLACEMENT_3D('',#41191,#29654,#29655);
#24911=AXIS2_PLACEMENT_3D('',#41199,#29658,#29659);
#24912=AXIS2_PLACEMENT_3D('',#41205,#29661,#29662);
#24913=AXIS2_PLACEMENT_3D('',#41208,#29663,#29664);
#24914=AXIS2_PLACEMENT_3D('',#41212,#29667,#29668);
#24915=AXIS2_PLACEMENT_3D('',#41220,#29671,#29672);
#24916=AXIS2_PLACEMENT_3D('',#41226,#29674,#29675);
#24917=AXIS2_PLACEMENT_3D('',#41229,#29676,#29677);
#24918=AXIS2_PLACEMENT_3D('',#41233,#29680,#29681);
#24919=AXIS2_PLACEMENT_3D('',#41241,#29684,#29685);
#24920=AXIS2_PLACEMENT_3D('',#41247,#29687,#29688);
#24921=AXIS2_PLACEMENT_3D('',#41250,#29689,#29690);
#24922=AXIS2_PLACEMENT_3D('',#41254,#29693,#29694);
#24923=AXIS2_PLACEMENT_3D('',#41262,#29697,#29698);
#24924=AXIS2_PLACEMENT_3D('',#41268,#29700,#29701);
#24925=AXIS2_PLACEMENT_3D('',#41271,#29702,#29703);
#24926=AXIS2_PLACEMENT_3D('',#41275,#29706,#29707);
#24927=AXIS2_PLACEMENT_3D('',#41283,#29710,#29711);
#24928=AXIS2_PLACEMENT_3D('',#41289,#29713,#29714);
#24929=AXIS2_PLACEMENT_3D('',#41292,#29715,#29716);
#24930=AXIS2_PLACEMENT_3D('',#41296,#29719,#29720);
#24931=AXIS2_PLACEMENT_3D('',#41304,#29723,#29724);
#24932=AXIS2_PLACEMENT_3D('',#41310,#29726,#29727);
#24933=AXIS2_PLACEMENT_3D('',#41313,#29728,#29729);
#24934=AXIS2_PLACEMENT_3D('',#41317,#29732,#29733);
#24935=AXIS2_PLACEMENT_3D('',#41325,#29736,#29737);
#24936=AXIS2_PLACEMENT_3D('',#41331,#29739,#29740);
#24937=AXIS2_PLACEMENT_3D('',#41334,#29741,#29742);
#24938=AXIS2_PLACEMENT_3D('',#41338,#29745,#29746);
#24939=AXIS2_PLACEMENT_3D('',#41346,#29749,#29750);
#24940=AXIS2_PLACEMENT_3D('',#41352,#29752,#29753);
#24941=AXIS2_PLACEMENT_3D('',#41355,#29754,#29755);
#24942=AXIS2_PLACEMENT_3D('',#41359,#29758,#29759);
#24943=AXIS2_PLACEMENT_3D('',#41367,#29762,#29763);
#24944=AXIS2_PLACEMENT_3D('',#41373,#29765,#29766);
#24945=AXIS2_PLACEMENT_3D('',#41376,#29767,#29768);
#24946=AXIS2_PLACEMENT_3D('',#41380,#29771,#29772);
#24947=AXIS2_PLACEMENT_3D('',#41388,#29775,#29776);
#24948=AXIS2_PLACEMENT_3D('',#41394,#29778,#29779);
#24949=AXIS2_PLACEMENT_3D('',#41397,#29780,#29781);
#24950=AXIS2_PLACEMENT_3D('',#41401,#29784,#29785);
#24951=AXIS2_PLACEMENT_3D('',#41409,#29788,#29789);
#24952=AXIS2_PLACEMENT_3D('',#41415,#29791,#29792);
#24953=AXIS2_PLACEMENT_3D('',#41418,#29793,#29794);
#24954=AXIS2_PLACEMENT_3D('',#41422,#29797,#29798);
#24955=AXIS2_PLACEMENT_3D('',#41430,#29801,#29802);
#24956=AXIS2_PLACEMENT_3D('',#41436,#29804,#29805);
#24957=AXIS2_PLACEMENT_3D('',#41439,#29806,#29807);
#24958=AXIS2_PLACEMENT_3D('',#41443,#29810,#29811);
#24959=AXIS2_PLACEMENT_3D('',#41451,#29814,#29815);
#24960=AXIS2_PLACEMENT_3D('',#41457,#29817,#29818);
#24961=AXIS2_PLACEMENT_3D('',#41460,#29819,#29820);
#24962=AXIS2_PLACEMENT_3D('',#41464,#29823,#29824);
#24963=AXIS2_PLACEMENT_3D('',#41472,#29827,#29828);
#24964=AXIS2_PLACEMENT_3D('',#41478,#29830,#29831);
#24965=AXIS2_PLACEMENT_3D('',#41481,#29832,#29833);
#24966=AXIS2_PLACEMENT_3D('',#41485,#29836,#29837);
#24967=AXIS2_PLACEMENT_3D('',#41493,#29840,#29841);
#24968=AXIS2_PLACEMENT_3D('',#41499,#29843,#29844);
#24969=AXIS2_PLACEMENT_3D('',#41502,#29845,#29846);
#24970=AXIS2_PLACEMENT_3D('',#41506,#29849,#29850);
#24971=AXIS2_PLACEMENT_3D('',#41514,#29853,#29854);
#24972=AXIS2_PLACEMENT_3D('',#41520,#29856,#29857);
#24973=AXIS2_PLACEMENT_3D('',#41523,#29858,#29859);
#24974=AXIS2_PLACEMENT_3D('',#41527,#29862,#29863);
#24975=AXIS2_PLACEMENT_3D('',#41535,#29866,#29867);
#24976=AXIS2_PLACEMENT_3D('',#41541,#29869,#29870);
#24977=AXIS2_PLACEMENT_3D('',#41542,#29871,#29872);
#24978=AXIS2_PLACEMENT_3D('',#41543,#29873,#29874);
#24979=AXIS2_PLACEMENT_3D('',#41544,#29875,#29876);
#24980=AXIS2_PLACEMENT_3D('',#41545,#29877,#29878);
#24981=AXIS2_PLACEMENT_3D('',#41546,#29879,#29880);
#24982=AXIS2_PLACEMENT_3D('',#41547,#29881,#29882);
#24983=AXIS2_PLACEMENT_3D('',#41548,#29883,#29884);
#24984=AXIS2_PLACEMENT_3D('',#41549,#29885,#29886);
#24985=AXIS2_PLACEMENT_3D('',#41550,#29887,#29888);
#24986=AXIS2_PLACEMENT_3D('',#41551,#29889,#29890);
#24987=AXIS2_PLACEMENT_3D('',#41552,#29891,#29892);
#24988=AXIS2_PLACEMENT_3D('',#41553,#29893,#29894);
#24989=AXIS2_PLACEMENT_3D('',#41554,#29895,#29896);
#24990=AXIS2_PLACEMENT_3D('',#41555,#29897,#29898);
#24991=AXIS2_PLACEMENT_3D('',#41556,#29899,#29900);
#24992=AXIS2_PLACEMENT_3D('',#41557,#29901,#29902);
#24993=AXIS2_PLACEMENT_3D('',#41558,#29903,#29904);
#24994=AXIS2_PLACEMENT_3D('',#41561,#29906,#29907);
#24995=AXIS2_PLACEMENT_3D('',#41562,#29908,#29909);
#24996=AXIS2_PLACEMENT_3D('',#41563,#29910,#29911);
#24997=AXIS2_PLACEMENT_3D('',#41564,#29912,#29913);
#24998=AXIS2_PLACEMENT_3D('',#41565,#29914,#29915);
#24999=AXIS2_PLACEMENT_3D('',#41566,#29916,#29917);
#25000=AXIS2_PLACEMENT_3D('',#41567,#29918,#29919);
#25001=AXIS2_PLACEMENT_3D('',#41568,#29920,#29921);
#25002=AXIS2_PLACEMENT_3D('',#41569,#29922,#29923);
#25003=AXIS2_PLACEMENT_3D('',#41570,#29924,#29925);
#25004=AXIS2_PLACEMENT_3D('',#41571,#29926,#29927);
#25005=AXIS2_PLACEMENT_3D('',#41572,#29928,#29929);
#25006=AXIS2_PLACEMENT_3D('',#41573,#29930,#29931);
#25007=AXIS2_PLACEMENT_3D('',#41574,#29932,#29933);
#25008=AXIS2_PLACEMENT_3D('',#41575,#29934,#29935);
#25009=AXIS2_PLACEMENT_3D('',#41576,#29936,#29937);
#25010=AXIS2_PLACEMENT_3D('',#41577,#29938,#29939);
#25011=AXIS2_PLACEMENT_3D('',#41578,#29940,#29941);
#25012=AXIS2_PLACEMENT_3D('',#41580,#29942,#29943);
#25013=AXIS2_PLACEMENT_3D('',#41584,#29945,#29946);
#25014=AXIS2_PLACEMENT_3D('',#41587,#29948,#29949);
#25015=AXIS2_PLACEMENT_3D('',#41588,#29950,#29951);
#25016=AXIS2_PLACEMENT_3D('',#41596,#29954,#29955);
#25017=AXIS2_PLACEMENT_3D('',#41601,#29957,#29958);
#25018=AXIS2_PLACEMENT_3D('',#41602,#29959,#29960);
#25019=AXIS2_PLACEMENT_3D('',#41604,#29961,#29962);
#25020=AXIS2_PLACEMENT_3D('',#41606,#29964,#29965);
#25021=AXIS2_PLACEMENT_3D('',#41610,#29967,#29968);
#25022=AXIS2_PLACEMENT_3D('',#41611,#29969,#29970);
#25023=AXIS2_PLACEMENT_3D('',#41620,#29975,#29976);
#25024=AXIS2_PLACEMENT_3D('',#41626,#29980,#29981);
#25025=AXIS2_PLACEMENT_3D('',#41632,#29985,#29986);
#25026=AXIS2_PLACEMENT_3D('',#41638,#29990,#29991);
#25027=AXIS2_PLACEMENT_3D('',#41644,#29995,#29996);
#25028=AXIS2_PLACEMENT_3D('',#41647,#29999,#30000);
#25029=AXIS2_PLACEMENT_3D('',#41648,#30001,#30002);
#25030=AXIS2_PLACEMENT_3D('',#41650,#30003,#30004);
#25031=AXIS2_PLACEMENT_3D('',#41651,#30005,#30006);
#25032=AXIS2_PLACEMENT_3D('',#41653,#30008,#30009);
#25033=AXIS2_PLACEMENT_3D('',#41654,#30010,#30011);
#25034=AXIS2_PLACEMENT_3D('',#41655,#30012,#30013);
#25035=AXIS2_PLACEMENT_3D('',#41657,#30014,#30015);
#25036=AXIS2_PLACEMENT_3D('',#41659,#30017,#30018);
#25037=AXIS2_PLACEMENT_3D('',#41660,#30019,#30020);
#29302=DIRECTION('axis',(0.,0.,1.));
#29303=DIRECTION('refdir',(1.,0.,0.));
#29304=DIRECTION('center_axis',(0.,0.,1.));
#29305=DIRECTION('ref_axis',(1.,0.,0.));
#29306=DIRECTION('',(0.,0.,-1.));
#29307=DIRECTION('center_axis',(0.,0.,-1.));
#29308=DIRECTION('ref_axis',(1.,0.,0.));
#29309=DIRECTION('',(0.,0.,-1.));
#29310=DIRECTION('center_axis',(0.,0.,1.));
#29311=DIRECTION('ref_axis',(1.,0.,0.));
#29312=DIRECTION('center_axis',(0.,0.,-1.));
#29313=DIRECTION('ref_axis',(1.,0.,0.));
#29314=DIRECTION('center_axis',(0.,0.,1.));
#29315=DIRECTION('ref_axis',(1.,0.,0.));
#29316=DIRECTION('',(0.,0.,-1.));
#29317=DIRECTION('center_axis',(0.,0.,1.));
#29318=DIRECTION('ref_axis',(1.,0.,0.));
#29319=DIRECTION('',(0.,0.,-1.));
#29320=DIRECTION('center_axis',(0.,0.,1.));
#29321=DIRECTION('ref_axis',(1.,0.,0.));
#29322=DIRECTION('',(0.,0.,-1.));
#29323=DIRECTION('center_axis',(0.,0.,1.));
#29324=DIRECTION('ref_axis',(1.,0.,0.));
#29325=DIRECTION('',(0.,0.,-1.));
#29326=DIRECTION('center_axis',(0.,0.,1.));
#29327=DIRECTION('ref_axis',(1.,0.,0.));
#29328=DIRECTION('',(0.,0.,-1.));
#29329=DIRECTION('center_axis',(0.,0.,1.));
#29330=DIRECTION('ref_axis',(1.,0.,0.));
#29331=DIRECTION('',(0.,0.,-1.));
#29332=DIRECTION('center_axis',(0.,0.,1.));
#29333=DIRECTION('ref_axis',(1.,0.,0.));
#29334=DIRECTION('',(0.,0.,-1.));
#29335=DIRECTION('center_axis',(0.,0.,1.));
#29336=DIRECTION('ref_axis',(1.,0.,0.));
#29337=DIRECTION('',(0.,0.,-1.));
#29338=DIRECTION('center_axis',(0.,0.,1.));
#29339=DIRECTION('ref_axis',(1.,0.,0.));
#29340=DIRECTION('',(0.,0.,-1.));
#29341=DIRECTION('center_axis',(0.,0.,1.));
#29342=DIRECTION('ref_axis',(1.,0.,0.));
#29343=DIRECTION('',(0.,0.,-1.));
#29344=DIRECTION('center_axis',(0.,0.,1.));
#29345=DIRECTION('ref_axis',(1.,0.,0.));
#29346=DIRECTION('',(0.,0.,-1.));
#29347=DIRECTION('center_axis',(0.,0.,1.));
#29348=DIRECTION('ref_axis',(1.,0.,0.));
#29349=DIRECTION('',(0.,0.,-1.));
#29350=DIRECTION('center_axis',(0.,0.,1.));
#29351=DIRECTION('ref_axis',(1.,0.,0.));
#29352=DIRECTION('',(0.,0.,-1.));
#29353=DIRECTION('center_axis',(0.,0.,1.));
#29354=DIRECTION('ref_axis',(-0.222205845997876,-0.97499977538683,0.));
#29355=DIRECTION('',(0.,0.,1.));
#29356=DIRECTION('center_axis',(0.,0.,1.));
#29357=DIRECTION('ref_axis',(1.,9.74274476199959E-14,0.));
#29358=DIRECTION('center_axis',(0.,0.,1.));
#29359=DIRECTION('ref_axis',(1.,9.74274476199959E-14,0.));
#29360=DIRECTION('',(0.,0.,1.));
#29361=DIRECTION('center_axis',(0.,0.,1.));
#29362=DIRECTION('ref_axis',(1.,9.74274476199959E-14,0.));
#29363=DIRECTION('',(0.,0.,1.));
#29364=DIRECTION('center_axis',(0.,0.,1.));
#29365=DIRECTION('ref_axis',(1.,9.74274476199959E-14,0.));
#29366=DIRECTION('',(0.,0.,1.));
#29367=DIRECTION('center_axis',(0.,0.,1.));
#29368=DIRECTION('ref_axis',(1.,9.74274476199959E-14,0.));
#29369=DIRECTION('',(0.,0.,1.));
#29370=DIRECTION('center_axis',(0.,0.,1.));
#29371=DIRECTION('ref_axis',(1.,9.74274476199959E-14,0.));
#29372=DIRECTION('',(0.,0.,1.));
#29373=DIRECTION('center_axis',(0.,0.,1.));
#29374=DIRECTION('ref_axis',(1.,9.74274476199959E-14,0.));
#29375=DIRECTION('',(0.,0.,1.));
#29376=DIRECTION('center_axis',(0.,0.,1.));
#29377=DIRECTION('ref_axis',(1.,9.74274476199959E-14,0.));
#29378=DIRECTION('',(0.,0.,1.));
#29379=DIRECTION('center_axis',(0.,0.,1.));
#29380=DIRECTION('ref_axis',(1.,9.74274476199959E-14,0.));
#29381=DIRECTION('',(0.,0.,1.));
#29382=DIRECTION('center_axis',(0.,0.,1.));
#29383=DIRECTION('ref_axis',(1.,9.74274476199959E-14,0.));
#29384=DIRECTION('',(0.,0.,1.));
#29385=DIRECTION('center_axis',(0.,0.,1.));
#29386=DIRECTION('ref_axis',(1.,9.74274476199959E-14,0.));
#29387=DIRECTION('',(0.,0.,1.));
#29388=DIRECTION('center_axis',(0.,0.,1.));
#29389=DIRECTION('ref_axis',(1.,9.74274476199959E-14,0.));
#29390=DIRECTION('',(0.,0.,1.));
#29391=DIRECTION('center_axis',(0.,0.,1.));
#29392=DIRECTION('ref_axis',(1.,9.74274476199959E-14,0.));
#29393=DIRECTION('',(0.,0.,1.));
#29394=DIRECTION('center_axis',(0.,0.,1.));
#29395=DIRECTION('ref_axis',(1.,9.74274476199959E-14,0.));
#29396=DIRECTION('',(0.,0.,1.));
#29397=DIRECTION('center_axis',(0.,0.,1.));
#29398=DIRECTION('ref_axis',(1.,9.74274476199959E-14,0.));
#29399=DIRECTION('',(0.,0.,1.));
#29400=DIRECTION('center_axis',(0.,0.,1.));
#29401=DIRECTION('ref_axis',(1.,0.,0.));
#29402=DIRECTION('center_axis',(0.,0.,1.));
#29403=DIRECTION('ref_axis',(1.,0.,0.));
#29404=DIRECTION('center_axis',(0.,0.,1.));
#29405=DIRECTION('ref_axis',(1.,0.,0.));
#29406=DIRECTION('center_axis',(0.,0.,1.));
#29407=DIRECTION('ref_axis',(1.,0.,0.));
#29408=DIRECTION('center_axis',(0.,0.,-1.));
#29409=DIRECTION('ref_axis',(1.,9.74274476199959E-14,0.));
#29410=DIRECTION('center_axis',(0.,0.,1.));
#29411=DIRECTION('ref_axis',(-0.710030672795894,0.704170748958667,0.));
#29412=DIRECTION('center_axis',(0.,0.,1.));
#29413=DIRECTION('ref_axis',(0.984807753012208,-0.17364817766693,0.));
#29414=DIRECTION('center_axis',(0.,0.,-1.));
#29415=DIRECTION('ref_axis',(1.,0.,0.));
#29416=DIRECTION('',(-0.996089805327885,-0.0883464754353932,0.));
#29417=DIRECTION('',(0.905801965515954,-0.423701309022563,0.));
#29418=DIRECTION('center_axis',(-0.423701309022563,-0.905801965515954,0.));
#29419=DIRECTION('ref_axis',(0.905801965515954,-0.423701309022563,0.));
#29420=DIRECTION('',(0.,0.,1.));
#29421=DIRECTION('',(0.,0.,1.));
#29422=DIRECTION('center_axis',(-0.0883464754353932,0.996089805327885,0.));
#29423=DIRECTION('ref_axis',(-0.996089805327885,-0.0883464754353932,0.));
#29424=DIRECTION('',(0.,0.,-1.));
#29425=DIRECTION('center_axis',(0.,0.,1.));
#29426=DIRECTION('ref_axis',(0.939692620785908,-0.342020143325669,0.));
#29427=DIRECTION('center_axis',(0.,0.,-1.));
#29428=DIRECTION('ref_axis',(1.,0.,0.));
#29429=DIRECTION('',(-0.996298167445974,0.0859648855277176,0.));
#29430=DIRECTION('',(0.818465838146947,-0.574555194725812,0.));
#29431=DIRECTION('center_axis',(-0.574555194725812,-0.818465838146947,0.));
#29432=DIRECTION('ref_axis',(0.818465838146947,-0.574555194725812,0.));
#29433=DIRECTION('',(0.,0.,1.));
#29434=DIRECTION('',(0.,0.,1.));
#29435=DIRECTION('center_axis',(0.0859648855277176,0.996298167445974,0.));
#29436=DIRECTION('ref_axis',(-0.996298167445974,0.0859648855277176,0.));
#29437=DIRECTION('',(0.,0.,-1.));
#29438=DIRECTION('center_axis',(0.,0.,1.));
#29439=DIRECTION('ref_axis',(0.866025403784438,-0.5,0.));
#29440=DIRECTION('center_axis',(0.,0.,-1.));
#29441=DIRECTION('ref_axis',(1.,0.,0.));
#29442=DIRECTION('',(-0.966234513897416,0.257664246944399,0.));
#29443=DIRECTION('',(0.706261040449543,-0.707951511576272,0.));
#29444=DIRECTION('center_axis',(-0.707951511576272,-0.706261040449543,0.));
#29445=DIRECTION('ref_axis',(0.706261040449543,-0.707951511576272,0.));
#29446=DIRECTION('',(0.,0.,1.));
#29447=DIRECTION('',(0.,0.,1.));
#29448=DIRECTION('center_axis',(0.257664246944399,0.966234513897416,0.));
#29449=DIRECTION('ref_axis',(-0.966234513897416,0.257664246944399,0.));
#29450=DIRECTION('',(0.,0.,-1.));
#29451=DIRECTION('center_axis',(0.,0.,1.));
#29452=DIRECTION('ref_axis',(0.766044443118978,-0.64278760968654,0.));
#29453=DIRECTION('center_axis',(0.,0.,-1.));
#29454=DIRECTION('ref_axis',(1.,0.,0.));
#29455=DIRECTION('',(-0.906812313582341,0.421534610602074,0.));
#29456=DIRECTION('',(0.572596858423411,-0.819837079988238,0.));
#29457=DIRECTION('center_axis',(-0.819837079988238,-0.572596858423411,0.));
#29458=DIRECTION('ref_axis',(0.572596858423411,-0.819837079988238,0.));
#29459=DIRECTION('',(0.,0.,1.));
#29460=DIRECTION('',(0.,0.,1.));
#29461=DIRECTION('center_axis',(0.421534610602074,0.906812313582341,0.));
#29462=DIRECTION('ref_axis',(-0.906812313582341,0.421534610602074,0.));
#29463=DIRECTION('',(0.,0.,-1.));
#29464=DIRECTION('center_axis',(0.,0.,1.));
#29465=DIRECTION('ref_axis',(0.642787609686539,-0.766044443118978,0.));
#29466=DIRECTION('center_axis',(0.,0.,-1.));
#29467=DIRECTION('ref_axis',(1.,0.,0.));
#29468=DIRECTION('',(-0.819837079988238,0.572596858423411,0.));
#29469=DIRECTION('',(0.421534610602074,-0.906812313582341,0.));
#29470=DIRECTION('center_axis',(-0.906812313582341,-0.421534610602074,0.));
#29471=DIRECTION('ref_axis',(0.421534610602074,-0.906812313582341,0.));
#29472=DIRECTION('',(0.,0.,1.));
#29473=DIRECTION('',(0.,0.,1.));
#29474=DIRECTION('center_axis',(0.572596858423411,0.819837079988238,0.));
#29475=DIRECTION('ref_axis',(-0.819837079988238,0.572596858423411,0.));
#29476=DIRECTION('',(0.,0.,-1.));
#29477=DIRECTION('center_axis',(0.,0.,1.));
#29478=DIRECTION('ref_axis',(0.5,-0.866025403784438,0.));
#29479=DIRECTION('center_axis',(0.,0.,-1.));
#29480=DIRECTION('ref_axis',(1.,0.,0.));
#29481=DIRECTION('',(-0.707951511576272,0.706261040449544,0.));
#29482=DIRECTION('',(0.257664246944398,-0.966234513897416,0.));
#29483=DIRECTION('center_axis',(-0.966234513897416,-0.257664246944398,0.));
#29484=DIRECTION('ref_axis',(0.257664246944398,-0.966234513897416,0.));
#29485=DIRECTION('',(0.,0.,1.));
#29486=DIRECTION('',(0.,0.,1.));
#29487=DIRECTION('center_axis',(0.706261040449544,0.707951511576272,0.));
#29488=DIRECTION('ref_axis',(-0.707951511576272,0.706261040449544,0.));
#29489=DIRECTION('',(0.,0.,-1.));
#29490=DIRECTION('center_axis',(0.,0.,1.));
#29491=DIRECTION('ref_axis',(0.342020143325668,-0.939692620785909,0.));
#29492=DIRECTION('center_axis',(0.,0.,-1.));
#29493=DIRECTION('ref_axis',(1.,0.,0.));
#29494=DIRECTION('',(-0.57455519472581,0.818465838146948,0.));
#29495=DIRECTION('',(0.0859648855277162,-0.996298167445974,0.));
#29496=DIRECTION('center_axis',(-0.996298167445974,-0.0859648855277162,
0.));
#29497=DIRECTION('ref_axis',(0.0859648855277162,-0.996298167445974,0.));
#29498=DIRECTION('',(0.,0.,1.));
#29499=DIRECTION('',(0.,0.,1.));
#29500=DIRECTION('center_axis',(0.818465838146948,0.57455519472581,0.));
#29501=DIRECTION('ref_axis',(-0.57455519472581,0.818465838146948,0.));
#29502=DIRECTION('',(0.,0.,-1.));
#29503=DIRECTION('center_axis',(0.,0.,1.));
#29504=DIRECTION('ref_axis',(0.17364817766693,-0.984807753012208,0.));
#29505=DIRECTION('center_axis',(0.,0.,-1.));
#29506=DIRECTION('ref_axis',(1.,0.,0.));
#29507=DIRECTION('',(-0.423701309022563,0.905801965515955,0.));
#29508=DIRECTION('',(-0.0883464754353936,-0.996089805327885,0.));
#29509=DIRECTION('center_axis',(-0.996089805327885,0.0883464754353937,0.));
#29510=DIRECTION('ref_axis',(-0.0883464754353937,-0.996089805327885,0.));
#29511=DIRECTION('',(0.,0.,1.));
#29512=DIRECTION('',(0.,0.,1.));
#29513=DIRECTION('center_axis',(0.905801965515955,0.423701309022563,0.));
#29514=DIRECTION('ref_axis',(-0.423701309022563,0.905801965515955,0.));
#29515=DIRECTION('',(0.,0.,-1.));
#29516=DIRECTION('center_axis',(0.,0.,1.));
#29517=DIRECTION('ref_axis',(-1.94289029309402E-16,-1.,0.));
#29518=DIRECTION('center_axis',(0.,0.,-1.));
#29519=DIRECTION('ref_axis',(1.,0.,0.));
#29520=DIRECTION('',(-0.259973473447872,0.96561575852067,0.));
#29521=DIRECTION('',(-0.259973473447873,-0.96561575852067,0.));
#29522=DIRECTION('center_axis',(-0.96561575852067,0.259973473447873,0.));
#29523=DIRECTION('ref_axis',(-0.259973473447873,-0.96561575852067,0.));
#29524=DIRECTION('',(0.,0.,1.));
#29525=DIRECTION('',(0.,0.,1.));
#29526=DIRECTION('center_axis',(0.96561575852067,0.259973473447872,0.));
#29527=DIRECTION('ref_axis',(-0.259973473447872,0.96561575852067,0.));
#29528=DIRECTION('',(0.,0.,-1.));
#29529=DIRECTION('center_axis',(0.,0.,1.));
#29530=DIRECTION('ref_axis',(-0.17364817766693,-0.984807753012208,0.));
#29531=DIRECTION('center_axis',(0.,0.,-1.));
#29532=DIRECTION('ref_axis',(1.,0.,0.));
#29533=DIRECTION('',(-0.0883464754353933,0.996089805327885,0.));
#29534=DIRECTION('',(-0.423701309022563,-0.905801965515955,0.));
#29535=DIRECTION('center_axis',(-0.905801965515955,0.423701309022563,0.));
#29536=DIRECTION('ref_axis',(-0.423701309022563,-0.905801965515955,0.));
#29537=DIRECTION('',(0.,0.,1.));
#29538=DIRECTION('',(0.,0.,1.));
#29539=DIRECTION('center_axis',(0.996089805327885,0.0883464754353932,0.));
#29540=DIRECTION('ref_axis',(-0.0883464754353932,0.996089805327885,0.));
#29541=DIRECTION('',(0.,0.,-1.));
#29542=DIRECTION('center_axis',(0.,0.,1.));
#29543=DIRECTION('ref_axis',(-0.342020143325669,-0.939692620785908,0.));
#29544=DIRECTION('center_axis',(0.,0.,-1.));
#29545=DIRECTION('ref_axis',(1.,0.,0.));
#29546=DIRECTION('',(0.0859648855277175,0.996298167445974,0.));
#29547=DIRECTION('',(-0.574555194725811,-0.818465838146947,0.));
#29548=DIRECTION('center_axis',(-0.818465838146947,0.574555194725811,0.));
#29549=DIRECTION('ref_axis',(-0.574555194725811,-0.818465838146947,0.));
#29550=DIRECTION('',(0.,0.,1.));
#29551=DIRECTION('',(0.,0.,1.));
#29552=DIRECTION('center_axis',(0.996298167445974,-0.0859648855277175,0.));
#29553=DIRECTION('ref_axis',(0.0859648855277175,0.996298167445974,0.));
#29554=DIRECTION('',(0.,0.,-1.));
#29555=DIRECTION('center_axis',(0.,0.,1.));
#29556=DIRECTION('ref_axis',(-0.5,-0.866025403784438,0.));
#29557=DIRECTION('center_axis',(0.,0.,-1.));
#29558=DIRECTION('ref_axis',(1.,0.,0.));
#29559=DIRECTION('',(0.257664246944399,0.966234513897416,0.));
#29560=DIRECTION('',(-0.707951511576272,-0.706261040449543,0.));
#29561=DIRECTION('center_axis',(-0.706261040449543,0.707951511576272,0.));
#29562=DIRECTION('ref_axis',(-0.707951511576272,-0.706261040449543,0.));
#29563=DIRECTION('',(0.,0.,1.));
#29564=DIRECTION('',(0.,0.,1.));
#29565=DIRECTION('center_axis',(0.966234513897416,-0.257664246944399,0.));
#29566=DIRECTION('ref_axis',(0.257664246944399,0.966234513897416,0.));
#29567=DIRECTION('',(0.,0.,-1.));
#29568=DIRECTION('center_axis',(0.,0.,1.));
#29569=DIRECTION('ref_axis',(-0.642787609686539,-0.766044443118978,0.));
#29570=DIRECTION('center_axis',(0.,0.,-1.));
#29571=DIRECTION('ref_axis',(1.,0.,0.));
#29572=DIRECTION('',(0.421534610602074,0.906812313582341,0.));
#29573=DIRECTION('',(-0.819837079988238,-0.572596858423411,0.));
#29574=DIRECTION('center_axis',(-0.572596858423411,0.819837079988238,0.));
#29575=DIRECTION('ref_axis',(-0.819837079988238,-0.572596858423411,0.));
#29576=DIRECTION('',(0.,0.,1.));
#29577=DIRECTION('',(0.,0.,1.));
#29578=DIRECTION('center_axis',(0.906812313582341,-0.421534610602074,0.));
#29579=DIRECTION('ref_axis',(0.421534610602074,0.906812313582341,0.));
#29580=DIRECTION('',(0.,0.,-1.));
#29581=DIRECTION('center_axis',(0.,0.,1.));
#29582=DIRECTION('ref_axis',(-0.766044443118978,-0.642787609686539,0.));
#29583=DIRECTION('center_axis',(0.,0.,-1.));
#29584=DIRECTION('ref_axis',(1.,0.,0.));
#29585=DIRECTION('',(0.572596858423411,0.819837079988238,0.));
#29586=DIRECTION('',(-0.906812313582341,-0.421534610602074,0.));
#29587=DIRECTION('center_axis',(-0.421534610602074,0.906812313582341,0.));
#29588=DIRECTION('ref_axis',(-0.906812313582341,-0.421534610602074,0.));
#29589=DIRECTION('',(0.,0.,1.));
#29590=DIRECTION('',(0.,0.,1.));
#29591=DIRECTION('center_axis',(0.819837079988238,-0.572596858423411,0.));
#29592=DIRECTION('ref_axis',(0.572596858423411,0.819837079988238,0.));
#29593=DIRECTION('',(0.,0.,-1.));
#29594=DIRECTION('center_axis',(0.,0.,1.));
#29595=DIRECTION('ref_axis',(-0.866025403784439,-0.5,0.));
#29596=DIRECTION('center_axis',(0.,0.,-1.));
#29597=DIRECTION('ref_axis',(1.,0.,0.));
#29598=DIRECTION('',(0.706261040449544,0.707951511576271,0.));
#29599=DIRECTION('',(-0.966234513897416,-0.257664246944398,0.));
#29600=DIRECTION('center_axis',(-0.257664246944398,0.966234513897416,0.));
#29601=DIRECTION('ref_axis',(-0.966234513897416,-0.257664246944398,0.));
#29602=DIRECTION('',(0.,0.,1.));
#29603=DIRECTION('',(0.,0.,1.));
#29604=DIRECTION('center_axis',(0.707951511576271,-0.706261040449544,0.));
#29605=DIRECTION('ref_axis',(0.706261040449544,0.707951511576271,0.));
#29606=DIRECTION('',(0.,0.,-1.));
#29607=DIRECTION('center_axis',(0.,0.,1.));
#29608=DIRECTION('ref_axis',(-0.939692620785909,-0.342020143325669,0.));
#29609=DIRECTION('center_axis',(0.,0.,-1.));
#29610=DIRECTION('ref_axis',(1.,0.,0.));
#29611=DIRECTION('',(0.818465838146948,0.574555194725811,0.));
#29612=DIRECTION('',(-0.996298167445974,-0.0859648855277167,0.));
#29613=DIRECTION('center_axis',(-0.0859648855277167,0.996298167445974,0.));
#29614=DIRECTION('ref_axis',(-0.996298167445974,-0.0859648855277167,0.));
#29615=DIRECTION('',(0.,0.,1.));
#29616=DIRECTION('',(0.,0.,1.));
#29617=DIRECTION('center_axis',(0.574555194725811,-0.818465838146948,0.));
#29618=DIRECTION('ref_axis',(0.818465838146948,0.574555194725811,0.));
#29619=DIRECTION('',(0.,0.,-1.));
#29620=DIRECTION('center_axis',(0.,0.,1.));
#29621=DIRECTION('ref_axis',(-0.984807753012208,-0.17364817766693,0.));
#29622=DIRECTION('center_axis',(0.,0.,-1.));
#29623=DIRECTION('ref_axis',(1.,0.,0.));
#29624=DIRECTION('',(0.905801965515955,0.423701309022563,0.));
#29625=DIRECTION('',(-0.996089805327885,0.0883464754353936,0.));
#29626=DIRECTION('center_axis',(0.0883464754353936,0.996089805327885,0.));
#29627=DIRECTION('ref_axis',(-0.996089805327885,0.0883464754353936,0.));
#29628=DIRECTION('',(0.,0.,1.));
#29629=DIRECTION('',(0.,0.,1.));
#29630=DIRECTION('center_axis',(0.423701309022563,-0.905801965515955,0.));
#29631=DIRECTION('ref_axis',(0.905801965515955,0.423701309022563,0.));
#29632=DIRECTION('',(0.,0.,-1.));
#29633=DIRECTION('center_axis',(0.,0.,1.));
#29634=DIRECTION('ref_axis',(-1.,1.11022302462516E-16,0.));
#29635=DIRECTION('center_axis',(0.,0.,-1.));
#29636=DIRECTION('ref_axis',(1.,0.,0.));
#29637=DIRECTION('',(0.96561575852067,0.259973473447872,0.));
#29638=DIRECTION('',(-0.96561575852067,0.259973473447873,0.));
#29639=DIRECTION('center_axis',(0.,0.,-1.));
#29640=DIRECTION('ref_axis',(1.,0.,0.));
#29641=DIRECTION('center_axis',(0.259973473447873,0.96561575852067,0.));
#29642=DIRECTION('ref_axis',(-0.96561575852067,0.259973473447873,0.));
#29643=DIRECTION('',(0.,0.,1.));
#29644=DIRECTION('',(0.,0.,1.));
#29645=DIRECTION('center_axis',(0.259973473447872,-0.96561575852067,0.));
#29646=DIRECTION('ref_axis',(0.96561575852067,0.259973473447872,0.));
#29647=DIRECTION('',(0.,0.,-1.));
#29648=DIRECTION('center_axis',(0.,0.,1.));
#29649=DIRECTION('ref_axis',(-0.984807753012208,0.173648177666931,0.));
#29650=DIRECTION('center_axis',(0.,0.,-1.));
#29651=DIRECTION('ref_axis',(1.,0.,0.));
#29652=DIRECTION('',(0.996089805327885,0.0883464754353928,0.));
#29653=DIRECTION('',(-0.905801965515954,0.423701309022564,0.));
#29654=DIRECTION('center_axis',(0.423701309022564,0.905801965515954,0.));
#29655=DIRECTION('ref_axis',(-0.905801965515954,0.423701309022564,0.));
#29656=DIRECTION('',(0.,0.,1.));
#29657=DIRECTION('',(0.,0.,1.));
#29658=DIRECTION('center_axis',(0.0883464754353928,-0.996089805327885,0.));
#29659=DIRECTION('ref_axis',(0.996089805327885,0.0883464754353928,0.));
#29660=DIRECTION('',(0.,0.,-1.));
#29661=DIRECTION('center_axis',(0.,0.,1.));
#29662=DIRECTION('ref_axis',(-0.939692620785908,0.342020143325669,0.));
#29663=DIRECTION('center_axis',(0.,0.,-1.));
#29664=DIRECTION('ref_axis',(1.,0.,0.));
#29665=DIRECTION('',(0.996298167445974,-0.085964885527717,0.));
#29666=DIRECTION('',(-0.818465838146948,0.574555194725811,0.));
#29667=DIRECTION('center_axis',(0.574555194725811,0.818465838146948,0.));
#29668=DIRECTION('ref_axis',(-0.818465838146948,0.574555194725811,0.));
#29669=DIRECTION('',(0.,0.,1.));
#29670=DIRECTION('',(0.,0.,1.));
#29671=DIRECTION('center_axis',(-0.085964885527717,-0.996298167445974,0.));
#29672=DIRECTION('ref_axis',(0.996298167445974,-0.085964885527717,0.));
#29673=DIRECTION('',(0.,0.,-1.));
#29674=DIRECTION('center_axis',(0.,0.,1.));
#29675=DIRECTION('ref_axis',(-0.866025403784439,0.5,0.));
#29676=DIRECTION('center_axis',(0.,0.,-1.));
#29677=DIRECTION('ref_axis',(1.,0.,0.));
#29678=DIRECTION('',(0.966234513897416,-0.257664246944398,0.));
#29679=DIRECTION('',(-0.706261040449544,0.707951511576272,0.));
#29680=DIRECTION('center_axis',(0.707951511576272,0.706261040449544,0.));
#29681=DIRECTION('ref_axis',(-0.706261040449544,0.707951511576272,0.));
#29682=DIRECTION('',(0.,0.,1.));
#29683=DIRECTION('',(0.,0.,1.));
#29684=DIRECTION('center_axis',(-0.257664246944398,-0.966234513897416,0.));
#29685=DIRECTION('ref_axis',(0.966234513897416,-0.257664246944398,0.));
#29686=DIRECTION('',(0.,0.,-1.));
#29687=DIRECTION('center_axis',(0.,0.,1.));
#29688=DIRECTION('ref_axis',(-0.766044443118978,0.642787609686539,0.));
#29689=DIRECTION('center_axis',(0.,0.,-1.));
#29690=DIRECTION('ref_axis',(1.,0.,0.));
#29691=DIRECTION('',(0.906812313582341,-0.421534610602074,0.));
#29692=DIRECTION('',(-0.572596858423411,0.819837079988238,0.));
#29693=DIRECTION('center_axis',(0.819837079988238,0.572596858423411,0.));
#29694=DIRECTION('ref_axis',(-0.572596858423411,0.819837079988238,0.));
#29695=DIRECTION('',(0.,0.,1.));
#29696=DIRECTION('',(0.,0.,1.));
#29697=DIRECTION('center_axis',(-0.421534610602074,-0.906812313582341,0.));
#29698=DIRECTION('ref_axis',(0.906812313582341,-0.421534610602074,0.));
#29699=DIRECTION('',(0.,0.,-1.));
#29700=DIRECTION('center_axis',(0.,0.,1.));
#29701=DIRECTION('ref_axis',(-0.642787609686539,0.766044443118978,0.));
#29702=DIRECTION('center_axis',(0.,0.,-1.));
#29703=DIRECTION('ref_axis',(1.,0.,0.));
#29704=DIRECTION('',(0.819837079988238,-0.572596858423411,0.));
#29705=DIRECTION('',(-0.421534610602074,0.906812313582341,0.));
#29706=DIRECTION('center_axis',(0.906812313582341,0.421534610602074,0.));
#29707=DIRECTION('ref_axis',(-0.421534610602074,0.906812313582341,0.));
#29708=DIRECTION('',(0.,0.,1.));
#29709=DIRECTION('',(0.,0.,1.));
#29710=DIRECTION('center_axis',(-0.572596858423411,-0.819837079988238,0.));
#29711=DIRECTION('ref_axis',(0.819837079988238,-0.572596858423411,0.));
#29712=DIRECTION('',(0.,0.,-1.));
#29713=DIRECTION('center_axis',(0.,0.,1.));
#29714=DIRECTION('ref_axis',(-0.5,0.866025403784439,0.));
#29715=DIRECTION('center_axis',(0.,0.,-1.));
#29716=DIRECTION('ref_axis',(1.,0.,0.));
#29717=DIRECTION('',(0.707951511576272,-0.706261040449544,0.));
#29718=DIRECTION('',(-0.257664246944398,0.966234513897416,0.));
#29719=DIRECTION('center_axis',(0.966234513897416,0.257664246944398,0.));
#29720=DIRECTION('ref_axis',(-0.257664246944398,0.966234513897416,0.));
#29721=DIRECTION('',(0.,0.,1.));
#29722=DIRECTION('',(0.,0.,1.));
#29723=DIRECTION('center_axis',(-0.706261040449544,-0.707951511576272,0.));
#29724=DIRECTION('ref_axis',(0.707951511576272,-0.706261040449544,0.));
#29725=DIRECTION('',(0.,0.,-1.));
#29726=DIRECTION('center_axis',(0.,0.,1.));
#29727=DIRECTION('ref_axis',(-0.342020143325669,0.939692620785909,0.));
#29728=DIRECTION('center_axis',(0.,0.,-1.));
#29729=DIRECTION('ref_axis',(1.,0.,0.));
#29730=DIRECTION('',(0.574555194725811,-0.818465838146948,0.));
#29731=DIRECTION('',(-0.0859648855277167,0.996298167445974,0.));
#29732=DIRECTION('center_axis',(0.996298167445974,0.0859648855277167,0.));
#29733=DIRECTION('ref_axis',(-0.0859648855277167,0.996298167445974,0.));
#29734=DIRECTION('',(0.,0.,1.));
#29735=DIRECTION('',(0.,0.,1.));
#29736=DIRECTION('center_axis',(-0.818465838146948,-0.574555194725811,0.));
#29737=DIRECTION('ref_axis',(0.574555194725811,-0.818465838146948,0.));
#29738=DIRECTION('',(0.,0.,-1.));
#29739=DIRECTION('center_axis',(0.,0.,1.));
#29740=DIRECTION('ref_axis',(-0.17364817766693,0.984807753012208,0.));
#29741=DIRECTION('center_axis',(0.,0.,-1.));
#29742=DIRECTION('ref_axis',(1.,0.,0.));
#29743=DIRECTION('',(0.423701309022563,-0.905801965515955,0.));
#29744=DIRECTION('',(0.0883464754353932,0.996089805327885,0.));
#29745=DIRECTION('center_axis',(0.996089805327885,-0.0883464754353932,0.));
#29746=DIRECTION('ref_axis',(0.0883464754353932,0.996089805327885,0.));
#29747=DIRECTION('',(0.,0.,1.));
#29748=DIRECTION('',(0.,0.,1.));
#29749=DIRECTION('center_axis',(-0.905801965515955,-0.423701309022563,0.));
#29750=DIRECTION('ref_axis',(0.423701309022563,-0.905801965515955,0.));
#29751=DIRECTION('',(0.,0.,-1.));
#29752=DIRECTION('center_axis',(0.,0.,1.));
#29753=DIRECTION('ref_axis',(5.55111512312578E-17,1.,0.));
#29754=DIRECTION('center_axis',(0.,0.,-1.));
#29755=DIRECTION('ref_axis',(1.,0.,0.));
#29756=DIRECTION('',(0.259973473447872,-0.96561575852067,0.));
#29757=DIRECTION('',(0.259973473447872,0.96561575852067,0.));
#29758=DIRECTION('center_axis',(0.96561575852067,-0.259973473447873,0.));
#29759=DIRECTION('ref_axis',(0.259973473447873,0.96561575852067,0.));
#29760=DIRECTION('',(0.,0.,1.));
#29761=DIRECTION('',(0.,0.,1.));
#29762=DIRECTION('center_axis',(-0.96561575852067,-0.259973473447872,0.));
#29763=DIRECTION('ref_axis',(0.259973473447872,-0.96561575852067,0.));
#29764=DIRECTION('',(0.,0.,-1.));
#29765=DIRECTION('center_axis',(0.,0.,1.));
#29766=DIRECTION('ref_axis',(0.17364817766693,0.984807753012208,0.));
#29767=DIRECTION('center_axis',(0.,0.,-1.));
#29768=DIRECTION('ref_axis',(1.,0.,0.));
#29769=DIRECTION('',(0.0883464754353931,-0.996089805327885,0.));
#29770=DIRECTION('',(0.423701309022563,0.905801965515954,0.));
#29771=DIRECTION('center_axis',(0.905801965515954,-0.423701309022563,0.));
#29772=DIRECTION('ref_axis',(0.423701309022563,0.905801965515954,0.));
#29773=DIRECTION('',(0.,0.,1.));
#29774=DIRECTION('',(0.,0.,1.));
#29775=DIRECTION('center_axis',(-0.996089805327885,-0.0883464754353932,
0.));
#29776=DIRECTION('ref_axis',(0.0883464754353932,-0.996089805327885,0.));
#29777=DIRECTION('',(0.,0.,-1.));
#29778=DIRECTION('center_axis',(0.,0.,1.));
#29779=DIRECTION('ref_axis',(0.342020143325669,0.939692620785908,0.));
#29780=DIRECTION('center_axis',(0.,0.,-1.));
#29781=DIRECTION('ref_axis',(1.,0.,0.));
#29782=DIRECTION('',(-0.085964885527717,-0.996298167445974,0.));
#29783=DIRECTION('',(0.574555194725811,0.818465838146948,0.));
#29784=DIRECTION('center_axis',(0.818465838146948,-0.574555194725811,0.));
#29785=DIRECTION('ref_axis',(0.574555194725811,0.818465838146948,0.));
#29786=DIRECTION('',(0.,0.,1.));
#29787=DIRECTION('',(0.,0.,1.));
#29788=DIRECTION('center_axis',(-0.996298167445974,0.085964885527717,0.));
#29789=DIRECTION('ref_axis',(-0.085964885527717,-0.996298167445974,0.));
#29790=DIRECTION('',(0.,0.,-1.));
#29791=DIRECTION('center_axis',(0.,0.,1.));
#29792=DIRECTION('ref_axis',(0.5,0.866025403784439,0.));
#29793=DIRECTION('center_axis',(0.,0.,-1.));
#29794=DIRECTION('ref_axis',(1.,0.,0.));
#29795=DIRECTION('',(-0.257664246944398,-0.966234513897416,0.));
#29796=DIRECTION('',(0.707951511576272,0.706261040449544,0.));
#29797=DIRECTION('center_axis',(0.706261040449544,-0.707951511576272,0.));
#29798=DIRECTION('ref_axis',(0.707951511576272,0.706261040449544,0.));
#29799=DIRECTION('',(0.,0.,1.));
#29800=DIRECTION('',(0.,0.,1.));
#29801=DIRECTION('center_axis',(-0.966234513897416,0.257664246944398,0.));
#29802=DIRECTION('ref_axis',(-0.257664246944398,-0.966234513897416,0.));
#29803=DIRECTION('',(0.,0.,-1.));
#29804=DIRECTION('center_axis',(0.,0.,1.));
#29805=DIRECTION('ref_axis',(0.642787609686539,0.766044443118978,0.));
#29806=DIRECTION('center_axis',(0.,0.,-1.));
#29807=DIRECTION('ref_axis',(1.,0.,0.));
#29808=DIRECTION('',(-0.421534610602074,-0.906812313582341,0.));
#29809=DIRECTION('',(0.819837079988238,0.572596858423411,0.));
#29810=DIRECTION('center_axis',(0.572596858423411,-0.819837079988238,0.));
#29811=DIRECTION('ref_axis',(0.819837079988238,0.572596858423411,0.));
#29812=DIRECTION('',(0.,0.,1.));
#29813=DIRECTION('',(0.,0.,1.));
#29814=DIRECTION('center_axis',(-0.906812313582341,0.421534610602074,0.));
#29815=DIRECTION('ref_axis',(-0.421534610602074,-0.906812313582341,0.));
#29816=DIRECTION('',(0.,0.,-1.));
#29817=DIRECTION('center_axis',(0.,0.,1.));
#29818=DIRECTION('ref_axis',(0.766044443118978,0.642787609686539,0.));
#29819=DIRECTION('center_axis',(0.,0.,-1.));
#29820=DIRECTION('ref_axis',(1.,0.,0.));
#29821=DIRECTION('',(-0.572596858423411,-0.819837079988238,0.));
#29822=DIRECTION('',(0.906812313582341,0.421534610602074,0.));
#29823=DIRECTION('center_axis',(0.421534610602074,-0.906812313582341,0.));
#29824=DIRECTION('ref_axis',(0.906812313582341,0.421534610602074,0.));
#29825=DIRECTION('',(0.,0.,1.));
#29826=DIRECTION('',(0.,0.,1.));
#29827=DIRECTION('center_axis',(-0.819837079988238,0.572596858423411,0.));
#29828=DIRECTION('ref_axis',(-0.572596858423411,-0.819837079988238,0.));
#29829=DIRECTION('',(0.,0.,-1.));
#29830=DIRECTION('center_axis',(0.,0.,1.));
#29831=DIRECTION('ref_axis',(0.866025403784439,0.5,0.));
#29832=DIRECTION('center_axis',(0.,0.,-1.));
#29833=DIRECTION('ref_axis',(1.,0.,0.));
#29834=DIRECTION('',(-0.706261040449544,-0.707951511576272,0.));
#29835=DIRECTION('',(0.966234513897416,0.257664246944398,0.));
#29836=DIRECTION('center_axis',(0.257664246944398,-0.966234513897416,0.));
#29837=DIRECTION('ref_axis',(0.966234513897416,0.257664246944398,0.));
#29838=DIRECTION('',(0.,0.,1.));
#29839=DIRECTION('',(0.,0.,1.));
#29840=DIRECTION('center_axis',(-0.707951511576272,0.706261040449544,0.));
#29841=DIRECTION('ref_axis',(-0.706261040449544,-0.707951511576272,0.));
#29842=DIRECTION('',(0.,0.,-1.));
#29843=DIRECTION('center_axis',(0.,0.,1.));
#29844=DIRECTION('ref_axis',(0.939692620785909,0.342020143325669,0.));
#29845=DIRECTION('center_axis',(0.,0.,-1.));
#29846=DIRECTION('ref_axis',(1.,0.,0.));
#29847=DIRECTION('',(-0.818465838146948,-0.574555194725811,0.));
#29848=DIRECTION('',(0.996298167445974,0.0859648855277167,0.));
#29849=DIRECTION('center_axis',(0.0859648855277167,-0.996298167445974,0.));
#29850=DIRECTION('ref_axis',(0.996298167445974,0.0859648855277167,0.));
#29851=DIRECTION('',(0.,0.,1.));
#29852=DIRECTION('',(0.,0.,1.));
#29853=DIRECTION('center_axis',(-0.574555194725811,0.818465838146948,0.));
#29854=DIRECTION('ref_axis',(-0.818465838146948,-0.574555194725811,0.));
#29855=DIRECTION('',(0.,0.,-1.));
#29856=DIRECTION('center_axis',(0.,0.,1.));
#29857=DIRECTION('ref_axis',(0.984807753012208,0.17364817766693,0.));
#29858=DIRECTION('center_axis',(0.,0.,-1.));
#29859=DIRECTION('ref_axis',(1.,0.,0.));
#29860=DIRECTION('',(-0.905801965515955,-0.423701309022563,0.));
#29861=DIRECTION('',(0.996089805327885,-0.0883464754353932,0.));
#29862=DIRECTION('center_axis',(-0.0883464754353933,-0.996089805327885,
0.));
#29863=DIRECTION('ref_axis',(0.996089805327885,-0.0883464754353933,0.));
#29864=DIRECTION('',(0.,0.,1.));
#29865=DIRECTION('',(0.,0.,1.));
#29866=DIRECTION('center_axis',(-0.423701309022563,0.905801965515955,0.));
#29867=DIRECTION('ref_axis',(-0.905801965515954,-0.423701309022563,0.));
#29868=DIRECTION('',(0.,0.,-1.));
#29869=DIRECTION('center_axis',(0.,0.,1.));
#29870=DIRECTION('ref_axis',(1.,0.,0.));
#29871=DIRECTION('center_axis',(0.,0.,1.));
#29872=DIRECTION('ref_axis',(1.,0.,0.));
#29873=DIRECTION('center_axis',(0.,0.,1.));
#29874=DIRECTION('ref_axis',(1.,0.,0.));
#29875=DIRECTION('center_axis',(0.,0.,1.));
#29876=DIRECTION('ref_axis',(1.,0.,0.));
#29877=DIRECTION('center_axis',(0.,0.,1.));
#29878=DIRECTION('ref_axis',(1.,0.,0.));
#29879=DIRECTION('center_axis',(0.,0.,1.));
#29880=DIRECTION('ref_axis',(1.,0.,0.));
#29881=DIRECTION('center_axis',(0.,0.,1.));
#29882=DIRECTION('ref_axis',(1.,0.,0.));
#29883=DIRECTION('center_axis',(0.,0.,1.));
#29884=DIRECTION('ref_axis',(1.,0.,0.));
#29885=DIRECTION('center_axis',(0.,0.,1.));
#29886=DIRECTION('ref_axis',(1.,0.,0.));
#29887=DIRECTION('center_axis',(0.,0.,1.));
#29888=DIRECTION('ref_axis',(1.,0.,0.));
#29889=DIRECTION('center_axis',(0.,0.,1.));
#29890=DIRECTION('ref_axis',(1.,0.,0.));
#29891=DIRECTION('center_axis',(0.,0.,1.));
#29892=DIRECTION('ref_axis',(1.,0.,0.));
#29893=DIRECTION('center_axis',(0.,0.,1.));
#29894=DIRECTION('ref_axis',(1.,0.,0.));
#29895=DIRECTION('center_axis',(0.,0.,1.));
#29896=DIRECTION('ref_axis',(1.,0.,0.));
#29897=DIRECTION('center_axis',(0.,0.,1.));
#29898=DIRECTION('ref_axis',(1.,0.,0.));
#29899=DIRECTION('center_axis',(0.,0.,1.));
#29900=DIRECTION('ref_axis',(1.,0.,0.));
#29901=DIRECTION('center_axis',(0.,0.,1.));
#29902=DIRECTION('ref_axis',(1.,0.,0.));
#29903=DIRECTION('center_axis',(0.,0.,1.));
#29904=DIRECTION('ref_axis',(1.,0.,0.));
#29905=DIRECTION('',(0.,0.,-1.));
#29906=DIRECTION('center_axis',(0.,0.,1.));
#29907=DIRECTION('ref_axis',(1.,0.,0.));
#29908=DIRECTION('center_axis',(0.,0.,1.));
#29909=DIRECTION('ref_axis',(1.,0.,0.));
#29910=DIRECTION('center_axis',(0.,0.,1.));
#29911=DIRECTION('ref_axis',(1.,0.,0.));
#29912=DIRECTION('center_axis',(0.,0.,1.));
#29913=DIRECTION('ref_axis',(1.,0.,0.));
#29914=DIRECTION('center_axis',(0.,0.,1.));
#29915=DIRECTION('ref_axis',(1.,0.,0.));
#29916=DIRECTION('center_axis',(0.,0.,1.));
#29917=DIRECTION('ref_axis',(1.,0.,0.));
#29918=DIRECTION('center_axis',(0.,0.,1.));
#29919=DIRECTION('ref_axis',(1.,0.,0.));
#29920=DIRECTION('center_axis',(0.,0.,1.));
#29921=DIRECTION('ref_axis',(1.,0.,0.));
#29922=DIRECTION('center_axis',(0.,0.,1.));
#29923=DIRECTION('ref_axis',(1.,0.,0.));
#29924=DIRECTION('center_axis',(0.,0.,1.));
#29925=DIRECTION('ref_axis',(1.,0.,0.));
#29926=DIRECTION('center_axis',(0.,0.,1.));
#29927=DIRECTION('ref_axis',(1.,0.,0.));
#29928=DIRECTION('center_axis',(0.,0.,1.));
#29929=DIRECTION('ref_axis',(1.,0.,0.));
#29930=DIRECTION('center_axis',(0.,0.,1.));
#29931=DIRECTION('ref_axis',(1.,0.,0.));
#29932=DIRECTION('center_axis',(0.,0.,1.));
#29933=DIRECTION('ref_axis',(1.,0.,0.));
#29934=DIRECTION('center_axis',(0.,0.,1.));
#29935=DIRECTION('ref_axis',(1.,0.,0.));
#29936=DIRECTION('center_axis',(0.,0.,1.));
#29937=DIRECTION('ref_axis',(1.,0.,0.));
#29938=DIRECTION('center_axis',(0.,0.,1.));
#29939=DIRECTION('ref_axis',(1.,0.,0.));
#29940=DIRECTION('center_axis',(0.,0.,1.));
#29941=DIRECTION('ref_axis',(1.,0.,0.));
#29942=DIRECTION('center_axis',(0.,0.,1.));
#29943=DIRECTION('ref_axis',(1.,0.,0.));
#29944=DIRECTION('',(0.,0.,-1.));
#29945=DIRECTION('center_axis',(0.,0.,-1.));
#29946=DIRECTION('ref_axis',(1.,0.,0.));
#29947=DIRECTION('',(0.,0.,1.));
#29948=DIRECTION('center_axis',(0.,0.,1.));
#29949=DIRECTION('ref_axis',(1.,0.,0.));
#29950=DIRECTION('center_axis',(-0.259973473447872,-0.96561575852067,0.));
#29951=DIRECTION('ref_axis',(0.96561575852067,-0.259973473447872,0.));
#29952=DIRECTION('',(0.96561575852067,-0.259973473447872,0.));
#29953=DIRECTION('',(0.,0.,1.));
#29954=DIRECTION('center_axis',(-0.259973473447872,0.96561575852067,0.));
#29955=DIRECTION('ref_axis',(-0.96561575852067,-0.259973473447872,0.));
#29956=DIRECTION('',(-0.96561575852067,-0.259973473447872,0.));
#29957=DIRECTION('center_axis',(0.,0.,1.));
#29958=DIRECTION('ref_axis',(1.,0.,0.));
#29959=DIRECTION('center_axis',(0.,0.,-1.));
#29960=DIRECTION('ref_axis',(1.,0.,0.));
#29961=DIRECTION('center_axis',(0.,0.,1.));
#29962=DIRECTION('ref_axis',(1.,0.,0.));
#29963=DIRECTION('',(-0.707106781186549,-8.65956056235495E-17,-0.707106781186546));
#29964=DIRECTION('center_axis',(0.,0.,1.));
#29965=DIRECTION('ref_axis',(1.,0.,0.));
#29966=DIRECTION('',(-0.844694227521705,-1.0344520819927E-16,0.535249158795705));
#29967=DIRECTION('center_axis',(0.,0.,-1.));
#29968=DIRECTION('ref_axis',(1.,0.,0.));
#29969=DIRECTION('center_axis',(0.5,0.866025403784439,0.));
#29970=DIRECTION('ref_axis',(0.866025403784439,-0.5,0.));
#29971=DIRECTION('',(0.866025403784439,-0.5,0.));
#29972=DIRECTION('',(0.,0.,-1.));
#29973=DIRECTION('',(0.866025403784439,-0.5,0.));
#29974=DIRECTION('',(0.,0.,-1.));
#29975=DIRECTION('center_axis',(-0.5,0.866025403784439,0.));
#29976=DIRECTION('ref_axis',(0.866025403784439,0.5,0.));
#29977=DIRECTION('',(0.866025403784439,0.5,0.));
#29978=DIRECTION('',(0.,0.,-1.));
#29979=DIRECTION('',(0.866025403784439,0.5,0.));
#29980=DIRECTION('center_axis',(-1.,-1.92296268638356E-16,0.));
#29981=DIRECTION('ref_axis',(-1.92296268638356E-16,1.,0.));
#29982=DIRECTION('',(-1.92296268638356E-16,1.,0.));
#29983=DIRECTION('',(0.,0.,-1.));
#29984=DIRECTION('',(-1.92296268638356E-16,1.,0.));
#29985=DIRECTION('center_axis',(-0.5,-0.866025403784439,0.));
#29986=DIRECTION('ref_axis',(-0.866025403784439,0.5,0.));
#29987=DIRECTION('',(-0.866025403784439,0.5,0.));
#29988=DIRECTION('',(0.,0.,-1.));
#29989=DIRECTION('',(-0.866025403784439,0.5,0.));
#29990=DIRECTION('center_axis',(0.5,-0.866025403784439,0.));
#29991=DIRECTION('ref_axis',(-0.866025403784439,-0.5,0.));
#29992=DIRECTION('',(-0.866025403784439,-0.5,0.));
#29993=DIRECTION('',(0.,0.,-1.));
#29994=DIRECTION('',(-0.866025403784439,-0.5,0.));
#29995=DIRECTION('center_axis',(1.,-3.84592537276713E-16,0.));
#29996=DIRECTION('ref_axis',(-3.84592537276713E-16,-1.,0.));
#29997=DIRECTION('',(-3.84592537276713E-16,-1.,0.));
#29998=DIRECTION('',(-3.84592537276713E-16,-1.,0.));
#29999=DIRECTION('center_axis',(0.,0.,-1.));
#30000=DIRECTION('ref_axis',(-1.,0.,0.));
#30001=DIRECTION('center_axis',(0.,0.,-1.));
#30002=DIRECTION('ref_axis',(-1.,0.,0.));
#30003=DIRECTION('center_axis',(0.,0.,1.));
#30004=DIRECTION('ref_axis',(1.,0.,0.));
#30005=DIRECTION('center_axis',(0.,0.,1.));
#30006=DIRECTION('ref_axis',(1.,0.,0.));
#30007=DIRECTION('',(0.707106781186547,8.65956056235493E-17,-0.707106781186548));
#30008=DIRECTION('center_axis',(0.,0.,1.));
#30009=DIRECTION('ref_axis',(0.952262827709432,-0.305279391644502,0.));
#30010=DIRECTION('center_axis',(0.,0.,1.));
#30011=DIRECTION('ref_axis',(1.,0.,0.));
#30012=DIRECTION('center_axis',(0.,0.,1.));
#30013=DIRECTION('ref_axis',(1.,0.,0.));
#30014=DIRECTION('center_axis',(0.,0.,1.));
#30015=DIRECTION('ref_axis',(1.,0.,0.));
#30016=DIRECTION('',(0.707106781186548,8.65956056235494E-17,-0.707106781186547));
#30017=DIRECTION('center_axis',(0.,0.,-1.));
#30018=DIRECTION('ref_axis',(-1.,0.,0.));
#30019=DIRECTION('center_axis',(0.,0.,1.));
#30020=DIRECTION('ref_axis',(1.,0.,0.));
#38705=CARTESIAN_POINT('',(0.,0.,0.));
#38706=CARTESIAN_POINT('Origin',(0.,0.,-0.387));
#38707=CARTESIAN_POINT('',(-0.146224572111309,-0.000111330236089668,-0.701584495415709));
#38708=CARTESIAN_POINT('',(-0.146224247785679,-0.000114915057078579,-0.708715504584291));
#38709=CARTESIAN_POINT('',(-0.14635,-1.79227059055215E-17,-0.387));
#38710=CARTESIAN_POINT('',(0.0262121662178374,-0.144200775921424,-0.73765));
#38711=CARTESIAN_POINT('Ctrl Pts',(-0.146224572111309,-0.000111330236089668,
-0.701584495415709));
#38712=CARTESIAN_POINT('Ctrl Pts',(-0.145989829674467,0.0324236203490019,
-0.703350319592403));
#38713=CARTESIAN_POINT('Ctrl Pts',(-0.135250992528874,0.0650987548480176,
-0.705116143769096));
#38714=CARTESIAN_POINT('Ctrl Pts',(-0.115283301657821,0.090528281986044,
-0.70688196794579));
#38715=CARTESIAN_POINT('Ctrl Pts',(-0.085590235853855,0.12834340179881,
-0.709507846612251));
#38716=CARTESIAN_POINT('Ctrl Pts',(-0.0354890897229695,0.150136061895647,
-0.712133725278713));
#38717=CARTESIAN_POINT('Ctrl Pts',(0.012418606607114,0.146058623298872,
-0.714759603945174));
#38718=CARTESIAN_POINT('Ctrl Pts',(0.0603263029371975,0.141981184702096,
-0.717385482611635));
#38719=CARTESIAN_POINT('Ctrl Pts',(0.106040549466479,0.112033647411709,
-0.720011361278096));
#38720=CARTESIAN_POINT('Ctrl Pts',(0.128919625858718,0.0697558642001005,
-0.722637239944558));
#38721=CARTESIAN_POINT('Ctrl Pts',(0.151798702250957,0.0274780809884917,
-0.725263118611019));
#38722=CARTESIAN_POINT('Ctrl Pts',(0.151842608506152,-0.0271299481443382,
-0.727888997277481));
#38723=CARTESIAN_POINT('Ctrl Pts',(0.129056444743052,-0.0694756899781577,
-0.730514875943942));
#38724=CARTESIAN_POINT('Ctrl Pts',(0.108418006355686,-0.107830105091238,
-0.732893250629295));
#38725=CARTESIAN_POINT('Ctrl Pts',(0.069050400143189,-0.136124873582162,
-0.735271625314647));
#38726=CARTESIAN_POINT('Ctrl Pts',(0.0262121662178374,-0.144200775921424,
-0.73765));
#38727=CARTESIAN_POINT('',(-0.14635,-1.79227059055215E-17,-0.73765));
#38728=CARTESIAN_POINT('Origin',(0.,0.,-0.73765));
#38729=CARTESIAN_POINT('',(-0.14635,-1.79227059055215E-17,-0.76765));
#38730=CARTESIAN_POINT('',(-0.14635,-1.79227059055215E-17,-0.387));
#38731=CARTESIAN_POINT('Origin',(0.,0.,-0.76765));
#38732=CARTESIAN_POINT('',(0.128823493644034,-0.0694465980833158,-0.73765));
#38733=CARTESIAN_POINT('Origin',(0.,0.,-0.73765));
#38734=CARTESIAN_POINT('Ctrl Pts',(0.128823493644033,-0.0694465980833164,
-0.73765));
#38735=CARTESIAN_POINT('Ctrl Pts',(0.15173931854053,-0.0269377250156972,
-0.735024121333539));
#38736=CARTESIAN_POINT('Ctrl Pts',(0.151797682753626,0.0274336672197081,
-0.732398242667077));
#38737=CARTESIAN_POINT('Ctrl Pts',(0.128963169514332,0.0696551524900372,
-0.729772364000616));
#38738=CARTESIAN_POINT('Ctrl Pts',(0.106128656275037,0.111876637760367,
-0.727146485334154));
#38739=CARTESIAN_POINT('Ctrl Pts',(0.0604012655833517,0.141948216065621,
-0.724520606667693));
#38740=CARTESIAN_POINT('Ctrl Pts',(0.0124881793788399,0.146075689420542,
-0.721894728001232));
#38741=CARTESIAN_POINT('Ctrl Pts',(-0.0354249068256719,0.150203162775464,
-0.719268849334771));
#38742=CARTESIAN_POINT('Ctrl Pts',(-0.0855236885430102,0.128386531180054,
-0.716642970668309));
#38743=CARTESIAN_POINT('Ctrl Pts',(-0.115232990782446,0.0905747836436524,
-0.714017092001848));
#38744=CARTESIAN_POINT('Ctrl Pts',(-0.135227118836764,0.0651277732727103,
-0.712249896195996));
#38745=CARTESIAN_POINT('Ctrl Pts',(-0.14598647497743,0.0324362794117622,
-0.710482700390144));
#38746=CARTESIAN_POINT('Ctrl Pts',(-0.146224247785679,-0.000114915057078579,
-0.708715504584291));
#38747=CARTESIAN_POINT('Origin',(0.,0.,-0.387));
#38748=CARTESIAN_POINT('',(-0.146579286092913,1.69649698835653E-5,-0.651584495415709));
#38749=CARTESIAN_POINT('',(-0.146579188640296,1.75704817259698E-5,-0.658715504584291));
#38750=CARTESIAN_POINT('',(-0.14635,-1.79227059055215E-17,-0.387));
#38751=CARTESIAN_POINT('Ctrl Pts',(-0.146579286092913,1.69649698835653E-5,
-0.651584495415709));
#38752=CARTESIAN_POINT('Ctrl Pts',(-0.146580846380414,0.000957028414167882,
-0.65163583559384));
#38753=CARTESIAN_POINT('Ctrl Pts',(-0.146572572236328,0.0018970636499291,
-0.651687175771971));
#38754=CARTESIAN_POINT('Ctrl Pts',(-0.146554379287511,0.00283690686036914,
-0.651738515950102));
#38755=CARTESIAN_POINT('Ctrl Pts',(-0.145623870708881,0.0509067485703208,
-0.654364394616563));
#38756=CARTESIAN_POINT('Ctrl Pts',(-0.118745958487551,0.0984742557093859,
-0.656990273283025));
#38757=CARTESIAN_POINT('Ctrl Pts',(-0.0780494861654621,0.124074549119317,
-0.659616151949486));
#38758=CARTESIAN_POINT('Ctrl Pts',(-0.0373530138433729,0.149674842529248,
-0.662242030615947));
#38759=CARTESIAN_POINT('Ctrl Pts',(0.0171620185794759,0.153307922210045,
-0.664867909282409));
#38760=CARTESIAN_POINT('Ctrl Pts',(0.0608956254433934,0.133334057017124,
-0.66749378794887));
#38761=CARTESIAN_POINT('Ctrl Pts',(0.104629232307311,0.113360191824202,
-0.670119666615332));
#38762=CARTESIAN_POINT('Ctrl Pts',(0.137581413612297,0.0697793817575608,
-0.672745545281793));
#38763=CARTESIAN_POINT('Ctrl Pts',(0.144882088293867,0.0222581942498008,
-0.675371423948254));
#38764=CARTESIAN_POINT('Ctrl Pts',(0.152182762975438,-0.0252629932579592,
-0.677997302614715));
#38765=CARTESIAN_POINT('Ctrl Pts',(0.133831931033593,-0.076724558206838,
-0.680623181281177));
#38766=CARTESIAN_POINT('Ctrl Pts',(0.0981110027231639,-0.108905303707465,
-0.683249059947638));
#38767=CARTESIAN_POINT('Ctrl Pts',(0.0623900744127351,-0.141086049208091,
-0.685874938614099));
#38768=CARTESIAN_POINT('Ctrl Pts',(0.00929904973372216,-0.153985975260466,
-0.688500817280561));
#38769=CARTESIAN_POINT('Ctrl Pts',(-0.0372055231842157,-0.141781954215198,
-0.691126695947022));
#38770=CARTESIAN_POINT('Ctrl Pts',(-0.0837100961021536,-0.12957793316993,
-0.693752574613483));
#38771=CARTESIAN_POINT('Ctrl Pts',(-0.123628217259017,-0.0922699650270199,
-0.696378453279944));
#38772=CARTESIAN_POINT('Ctrl Pts',(-0.138944785098925,-0.0466971911912179,
-0.699004331946406));
#38773=CARTESIAN_POINT('Ctrl Pts',(-0.143961423189176,-0.0317707327644562,
-0.699864386436174));
#38774=CARTESIAN_POINT('Ctrl Pts',(-0.146338904721208,-0.0159576589331395,
-0.700724440925942));
#38775=CARTESIAN_POINT('Ctrl Pts',(-0.146224572111309,-0.000111330236089668,
-0.701584495415709));
#38776=CARTESIAN_POINT('Ctrl Pts',(-0.146224247785679,-0.000114915057078579,
-0.708715504584291));
#38777=CARTESIAN_POINT('Ctrl Pts',(-0.146339781918618,-0.0159315849983372,
-0.707856821723683));
#38778=CARTESIAN_POINT('Ctrl Pts',(-0.143971168753899,-0.0317151302334793,
-0.706998138863074));
#38779=CARTESIAN_POINT('Ctrl Pts',(-0.138970783508294,-0.046618358270845,
-0.706139456002465));
#38780=CARTESIAN_POINT('Ctrl Pts',(-0.123679451233175,-0.0921928891715474,
-0.703513577336003));
#38781=CARTESIAN_POINT('Ctrl Pts',(-0.0837769639214024,-0.129535087495559,
-0.700887698669541));
#38782=CARTESIAN_POINT('Ctrl Pts',(-0.0372778401516794,-0.141766375685469,
-0.69826182000308));
#38783=CARTESIAN_POINT('Ctrl Pts',(0.00922128361804363,-0.153997663875379,
-0.695635941336619));
#38784=CARTESIAN_POINT('Ctrl Pts',(0.0623170438457172,-0.141118041931188,
-0.693010062670158));
#38785=CARTESIAN_POINT('Ctrl Pts',(0.0980541504731311,-0.108954078842552,
-0.690384184003697));
#38786=CARTESIAN_POINT('Ctrl Pts',(0.133791257100545,-0.0767901157539168,
-0.687758305337235));
#38787=CARTESIAN_POINT('Ctrl Pts',(0.152169710127699,-0.0253418115208371,
-0.685132426670773));
#38788=CARTESIAN_POINT('Ctrl Pts',(0.144893849521265,0.0221822521721539,
-0.682506548004312));
#38789=CARTESIAN_POINT('Ctrl Pts',(0.137617988914832,0.0697063158651454,
-0.679880669337851));
#38790=CARTESIAN_POINT('Ctrl Pts',(0.104687814674811,0.113306139018048,
-0.67725479067139));
#38791=CARTESIAN_POINT('Ctrl Pts',(0.0609644168294508,0.133303084391365,
-0.674628912004929));
#38792=CARTESIAN_POINT('Ctrl Pts',(0.0172410189840913,0.153300029764682,
-0.672003033338467));
#38793=CARTESIAN_POINT('Ctrl Pts',(-0.0372756024666062,0.149694097358414,
-0.669377154672006));
#38794=CARTESIAN_POINT('Ctrl Pts',(-0.0779852394339466,0.124114604981169,
-0.666751276005544));
#38795=CARTESIAN_POINT('Ctrl Pts',(-0.118694876401287,0.0985351126039237,
-0.664125397339083));
#38796=CARTESIAN_POINT('Ctrl Pts',(-0.14559752888527,0.050982060255701,
-0.661499518672622));
#38797=CARTESIAN_POINT('Ctrl Pts',(-0.146552928848993,0.00291283741010483,
-0.65887364000616));
#38798=CARTESIAN_POINT('Ctrl Pts',(-0.146572107518371,0.00194789731459742,
-0.658820928198871));
#38799=CARTESIAN_POINT('Ctrl Pts',(-0.146580830372945,0.000982749220839569,
-0.658768216391581));
#38800=CARTESIAN_POINT('Ctrl Pts',(-0.146579188640296,1.75704817259698E-5,
-0.658715504584291));
#38801=CARTESIAN_POINT('Origin',(0.,0.,-0.387));
#38802=CARTESIAN_POINT('',(-0.146183638882289,9.23670094306398E-5,-0.601584495415709));
#38803=CARTESIAN_POINT('',(-0.146183142687711,9.20871909961158E-5,-0.608715504584291));
#38804=CARTESIAN_POINT('',(-0.14635,-1.79227059055215E-17,-0.387));
#38805=CARTESIAN_POINT('Ctrl Pts',(-0.146183638882289,9.23670094306398E-5,
-0.601584495415709));
#38806=CARTESIAN_POINT('Ctrl Pts',(-0.146288013988482,0.0178439142218399,
-0.602547230261739));
#38807=CARTESIAN_POINT('Ctrl Pts',(-0.143291093723304,0.0355614332192032,
-0.603509965107768));
#38808=CARTESIAN_POINT('Ctrl Pts',(-0.137032927084621,0.0520404416997214,
-0.604472699953798));
#38809=CARTESIAN_POINT('Ctrl Pts',(-0.119963651639312,0.0969872689511545,
-0.60709857862026));
#38810=CARTESIAN_POINT('Ctrl Pts',(-0.0786327707208103,0.132720363140831,
-0.609724457286721));
#38811=CARTESIAN_POINT('Ctrl Pts',(-0.0316910142969177,0.143115023213958,
-0.612350335953183));
#38812=CARTESIAN_POINT('Ctrl Pts',(0.0152507421269743,0.153509683287086,
-0.614976214619644));
#38813=CARTESIAN_POINT('Ctrl Pts',(0.0678033740562569,0.138565909243665,
-0.617602093286105));
#38814=CARTESIAN_POINT('Ctrl Pts',(0.102252295370017,0.105027133840093,
-0.620227971952566));
#38815=CARTESIAN_POINT('Ctrl Pts',(0.136701216683777,0.0714883584365206,
-0.622853850619027));
#38816=CARTESIAN_POINT('Ctrl Pts',(0.153046427382013,0.0193545816727964,
-0.625479729285489));
#38817=CARTESIAN_POINT('Ctrl Pts',(0.143912078720802,-0.027848605678599,
-0.62810560795195));
#38818=CARTESIAN_POINT('Ctrl Pts',(0.134777730059591,-0.0750517930299941,
-0.630731486618412));
#38819=CARTESIAN_POINT('Ctrl Pts',(0.100163822038932,-0.117324390969061,
-0.633357365284873));
#38820=CARTESIAN_POINT('Ctrl Pts',(0.0556900327358894,-0.135590739689116,
-0.635983243951334));
#38821=CARTESIAN_POINT('Ctrl Pts',(0.0112162434328469,-0.153857088409171,
-0.638609122617795));
#38822=CARTESIAN_POINT('Ctrl Pts',(-0.0431174271525793,-0.148117187910216,
-0.641235001284257));
#38823=CARTESIAN_POINT('Ctrl Pts',(-0.0827927099773264,-0.120961149520319,
-0.643860879950718));
#38824=CARTESIAN_POINT('Ctrl Pts',(-0.121692276805127,-0.094336055635236,
-0.646435418439049));
#38825=CARTESIAN_POINT('Ctrl Pts',(-0.146501042885148,-0.047124077521472,
-0.649009956927379));
#38826=CARTESIAN_POINT('Ctrl Pts',(-0.146579286092913,1.69649698835653E-5,
-0.651584495415709));
#38827=CARTESIAN_POINT('Ctrl Pts',(-0.146579188640296,1.75704817259698E-5,
-0.658715504584291));
#38828=CARTESIAN_POINT('Ctrl Pts',(-0.146499046215644,-0.0470983618370304,
-0.656142337725119));
#38829=CARTESIAN_POINT('Ctrl Pts',(-0.121720317494026,-0.0942873213731057,
-0.653569170865948));
#38830=CARTESIAN_POINT('Ctrl Pts',(-0.0828552235665306,-0.120918396970429,
-0.650996004006776));
#38831=CARTESIAN_POINT('Ctrl Pts',(-0.0431939708768843,-0.148095015162397,
-0.648370125340315));
#38832=CARTESIAN_POINT('Ctrl Pts',(0.0111366819458703,-0.153862858203364,
-0.645744246673854));
#38833=CARTESIAN_POINT('Ctrl Pts',(0.0556198997683811,-0.13561947345926,
-0.643118368007392));
#38834=CARTESIAN_POINT('Ctrl Pts',(0.100103117590892,-0.117376088715157,
-0.640492489340931));
#38835=CARTESIAN_POINT('Ctrl Pts',(0.134738900413159,-0.0751214761859832,
-0.637866610674469));
#38836=CARTESIAN_POINT('Ctrl Pts',(0.143897661097196,-0.0279230386888887,
-0.635240732008008));
#38837=CARTESIAN_POINT('Ctrl Pts',(0.153056421781233,0.0192753988082057,
-0.632614853341547));
#38838=CARTESIAN_POINT('Ctrl Pts',(0.136738160327041,0.071417661273221,
-0.629988974675086));
#38839=CARTESIAN_POINT('Ctrl Pts',(0.102306584507141,0.104974254510237,
-0.627363096008625));
#38840=CARTESIAN_POINT('Ctrl Pts',(0.0678750086872403,0.138530847747253,
-0.624737217342164));
#38841=CARTESIAN_POINT('Ctrl Pts',(0.0153301185016322,0.15350177175627,
-0.622111338675701));
#38842=CARTESIAN_POINT('Ctrl Pts',(-0.031617003941353,0.143131381312434,
-0.61948546000924));
#38843=CARTESIAN_POINT('Ctrl Pts',(-0.0785641263843382,0.132760990868598,
-0.616859581342778));
#38844=CARTESIAN_POINT('Ctrl Pts',(-0.119913481084701,0.0970492859719075,
-0.614233702676318));
#38845=CARTESIAN_POINT('Ctrl Pts',(-0.137005996168408,0.0521112951099759,
-0.611607824009857));
#38846=CARTESIAN_POINT('Ctrl Pts',(-0.143281611519541,0.0356120529609342,
-0.610643717534669));
#38847=CARTESIAN_POINT('Ctrl Pts',(-0.146287323594326,0.017869076542175,
-0.60967961105948));
#38848=CARTESIAN_POINT('Ctrl Pts',(-0.146183142687711,9.20871909961158E-5,
-0.608715504584291));
#38849=CARTESIAN_POINT('Origin',(0.,0.,-0.387));
#38850=CARTESIAN_POINT('',(-0.146276019243273,-0.00012357004413352,-0.55158449541571));
#38851=CARTESIAN_POINT('',(-0.146276703831537,-0.000123683174109515,-0.558715504584291));
#38852=CARTESIAN_POINT('',(-0.14635,-1.79227059055215E-17,-0.387));
#38853=CARTESIAN_POINT('Ctrl Pts',(-0.146276019243273,-0.00012357004413352,
-0.55158449541571));
#38854=CARTESIAN_POINT('Ctrl Pts',(-0.145991697039028,0.0343777221702149,
-0.553458624929638));
#38855=CARTESIAN_POINT('Ctrl Pts',(-0.133769924250195,0.0690603428635732,
-0.555332754443566));
#38856=CARTESIAN_POINT('Ctrl Pts',(-0.111492926407665,0.0951606952569379,
-0.557206883957495));
#38857=CARTESIAN_POINT('Ctrl Pts',(-0.0802801991373442,0.131730397632097,
-0.559832762623956));
#38858=CARTESIAN_POINT('Ctrl Pts',(-0.0293277101925237,0.151451950914244,
-0.562458641290417));
#38859=CARTESIAN_POINT('Ctrl Pts',(0.0183720222342842,0.145425923930635,
-0.565084519956878));
#38860=CARTESIAN_POINT('Ctrl Pts',(0.066071754661092,0.139399896947026,
-0.56771039862334));
#38861=CARTESIAN_POINT('Ctrl Pts',(0.110518730569887,0.107626289697661,
-0.570336277289801));
#38862=CARTESIAN_POINT('Ctrl Pts',(0.131656071121403,0.0644430717323258,
-0.572962155956262));
#38863=CARTESIAN_POINT('Ctrl Pts',(0.152793411672919,0.021259853766991,
-0.575588034622724));
#38864=CARTESIAN_POINT('Ctrl Pts',(0.150621116867156,-0.0333329749143135,
-0.578213913289185));
#38865=CARTESIAN_POINT('Ctrl Pts',(0.126119443458436,-0.0747001777727409,
-0.580839791955647));
#38866=CARTESIAN_POINT('Ctrl Pts',(0.101617770049717,-0.116067380631168,
-0.583465670622108));
#38867=CARTESIAN_POINT('Ctrl Pts',(0.0547867180380415,-0.144208957666719,
-0.586091549288569));
#38868=CARTESIAN_POINT('Ctrl Pts',(0.00675899061544872,-0.146425908097131,
-0.58871742795503));
#38869=CARTESIAN_POINT('Ctrl Pts',(-0.0412687368071444,-0.148642858527543,
-0.591343306621491));
#38870=CARTESIAN_POINT('Ctrl Pts',(-0.0904931396406548,-0.124935182352816,
-0.593969185287953));
#38871=CARTESIAN_POINT('Ctrl Pts',(-0.118701506071351,-0.086001064108858,
-0.596595063954414));
#38872=CARTESIAN_POINT('Ctrl Pts',(-0.136567742966793,-0.0613414943471455,
-0.598258207774846));
#38873=CARTESIAN_POINT('Ctrl Pts',(-0.146003328785914,-0.0305737880291827,
-0.599921351595278));
#38874=CARTESIAN_POINT('Ctrl Pts',(-0.146183638882289,9.23670094306398E-5,
-0.601584495415709));
#38875=CARTESIAN_POINT('Ctrl Pts',(-0.146183142687711,9.20871909961158E-5,
-0.608715504584291));
#38876=CARTESIAN_POINT('Ctrl Pts',(-0.146003572341562,-0.0305490373202445,
-0.607053732393019));
#38877=CARTESIAN_POINT('Ctrl Pts',(-0.136584715823453,-0.0612912120020383,
-0.605391960201745));
#38878=CARTESIAN_POINT('Ctrl Pts',(-0.118745956960722,-0.0859396723257687,
-0.603730188010472));
#38879=CARTESIAN_POINT('Ctrl Pts',(-0.0905577272022776,-0.124888372072408,
-0.601104309344011));
#38880=CARTESIAN_POINT('Ctrl Pts',(-0.0413455922183362,-0.148621494738514,
-0.59847843067755));
#38881=CARTESIAN_POINT('Ctrl Pts',(0.00668327362850226,-0.146429378651901,
-0.595852552011089));
#38882=CARTESIAN_POINT('Ctrl Pts',(0.0547121394753407,-0.144237262565288,
-0.593226673344627));
#38883=CARTESIAN_POINT('Ctrl Pts',(0.101557736185076,-0.116119907725956,
-0.590600794678166));
#38884=CARTESIAN_POINT('Ctrl Pts',(0.126080796403966,-0.0747653815530347,
-0.587974916011705));
#38885=CARTESIAN_POINT('Ctrl Pts',(0.150603856622856,-0.0334108553801132,
-0.585349037345243));
#38886=CARTESIAN_POINT('Ctrl Pts',(0.152804380350901,0.021180842126398,
-0.582723158678783));
#38887=CARTESIAN_POINT('Ctrl Pts',(0.131689372842645,0.0643749832966417,
-0.580097280012321));
#38888=CARTESIAN_POINT('Ctrl Pts',(0.110574365334389,0.107569124466885,
-0.57747140134586));
#38889=CARTESIAN_POINT('Ctrl Pts',(0.0661438265898331,0.139365709300861,
-0.574845522679397));
#38890=CARTESIAN_POINT('Ctrl Pts',(0.0184472178872199,0.145416400350861,
-0.572219644012936));
#38891=CARTESIAN_POINT('Ctrl Pts',(-0.0292493908153934,0.15146709140086,
-0.569593765346475));
#38892=CARTESIAN_POINT('Ctrl Pts',(-0.080212069476064,0.131771888666882,
-0.566967886680015));
#38893=CARTESIAN_POINT('Ctrl Pts',(-0.111443701633747,0.0952183320922368,
-0.564342008013553));
#38894=CARTESIAN_POINT('Ctrl Pts',(-0.133750506041868,0.069110409431805,
-0.562466506870466));
#38895=CARTESIAN_POINT('Ctrl Pts',(-0.145991807584391,0.0344024457716816,
-0.560591005727379));
#38896=CARTESIAN_POINT('Ctrl Pts',(-0.146276703831537,-0.000123683174109515,
-0.558715504584291));
#38897=CARTESIAN_POINT('Origin',(0.,0.,-0.387));
#38898=CARTESIAN_POINT('',(-0.146558953229823,5.11349905732411E-5,-0.501584495415709));
#38899=CARTESIAN_POINT('',(-0.146558577250774,5.15455280380561E-5,-0.508715504584291));
#38900=CARTESIAN_POINT('',(-0.14635,-1.79227059055215E-17,-0.387));
#38901=CARTESIAN_POINT('Ctrl Pts',(-0.146558953229823,5.11349905732411E-5,
-0.501584495415709));
#38902=CARTESIAN_POINT('Ctrl Pts',(-0.146572307834264,0.00297540766026488,
-0.501744140931075));
#38903=CARTESIAN_POINT('Ctrl Pts',(-0.146492243279588,0.00589893547541245,
-0.501903786446441));
#38904=CARTESIAN_POINT('Ctrl Pts',(-0.14631642585259,0.00881669344130144,
-0.502063431961807));
#38905=CARTESIAN_POINT('Ctrl Pts',(-0.143424548622659,0.0568085106807304,
-0.504689310628268));
#38906=CARTESIAN_POINT('Ctrl Pts',(-0.114627428195741,0.103239337167309,
-0.507315189294729));
#38907=CARTESIAN_POINT('Ctrl Pts',(-0.0729198824504026,0.127157073342488,
-0.509941067961191));
#38908=CARTESIAN_POINT('Ctrl Pts',(-0.0312123367050647,0.151074809517666,
-0.512566946627652));
#38909=CARTESIAN_POINT('Ctrl Pts',(0.0234056343586937,0.152479455381444,
-0.515192825294113));
#38910=CARTESIAN_POINT('Ctrl Pts',(0.0662874488469095,0.130737158768342,
-0.517818703960575));
#38911=CARTESIAN_POINT('Ctrl Pts',(0.109169263335126,0.108994862155241,
-0.520444582627036));
#38912=CARTESIAN_POINT('Ctrl Pts',(0.140314921247799,0.0641056230652594,
-0.523070461293497));
#38913=CARTESIAN_POINT('Ctrl Pts',(0.145669817601684,0.0163258934620395,
-0.525696339959959));
#38914=CARTESIAN_POINT('Ctrl Pts',(0.151024713955569,-0.0314538361411797,
-0.52832221862642));
#38915=CARTESIAN_POINT('Ctrl Pts',(0.130588848750667,-0.0821240562576371,
-0.530948097292881));
#38916=CARTESIAN_POINT('Ctrl Pts',(0.093583989390229,-0.112819623682389,
-0.533573975959343));
#38917=CARTESIAN_POINT('Ctrl Pts',(0.0565791300297904,-0.143515191107141,
-0.536199854625804));
#38918=CARTESIAN_POINT('Ctrl Pts',(0.00300527651381574,-0.154236105840187,
-0.538825733292265));
#38919=CARTESIAN_POINT('Ctrl Pts',(-0.0429621515554171,-0.140144511453598,
-0.541451611958726));
#38920=CARTESIAN_POINT('Ctrl Pts',(-0.0889295796246497,-0.126052917067009,
-0.544077490625188));
#38921=CARTESIAN_POINT('Ctrl Pts',(-0.12729058224714,-0.0871488135607851,
-0.546703369291649));
#38922=CARTESIAN_POINT('Ctrl Pts',(-0.140734600760475,-0.040987836073588,
-0.54932924795811));
#38923=CARTESIAN_POINT('Ctrl Pts',(-0.144583418930606,-0.0277726498011545,
-0.550080997110644));
#38924=CARTESIAN_POINT('Ctrl Pts',(-0.146390066311258,-0.0139626974847263,
-0.550832746263176));
#38925=CARTESIAN_POINT('Ctrl Pts',(-0.146276019243273,-0.00012357004413352,
-0.55158449541571));
#38926=CARTESIAN_POINT('Ctrl Pts',(-0.146276703831537,-0.000123683174109515,
-0.558715504584291));
#38927=CARTESIAN_POINT('Ctrl Pts',(-0.146390689227462,-0.0139373943656652,
-0.557965127060917));
#38928=CARTESIAN_POINT('Ctrl Pts',(-0.144590746625787,-0.0277219982676888,
-0.557214749537542));
#38929=CARTESIAN_POINT('Ctrl Pts',(-0.140755772561096,-0.0409150567738682,
-0.556464372014168));
#38930=CARTESIAN_POINT('Ctrl Pts',(-0.127335625676068,-0.0870829786500136,
-0.553838493347707));
#38931=CARTESIAN_POINT('Ctrl Pts',(-0.088994746251319,-0.126006911986991,
-0.551212614681246));
#38932=CARTESIAN_POINT('Ctrl Pts',(-0.0430346122416979,-0.140122273475387,
-0.548586736014785));
#38933=CARTESIAN_POINT('Ctrl Pts',(0.00292552176792324,-0.154237634963784,
-0.545960857348324));
#38934=CARTESIAN_POINT('Ctrl Pts',(0.0565049103624161,-0.1435444246036,
-0.543334978681862));
#38935=CARTESIAN_POINT('Ctrl Pts',(0.0935256361956055,-0.112867997047911,
-0.540709100015401));
#38936=CARTESIAN_POINT('Ctrl Pts',(0.130546362028795,-0.082191569492223,
-0.538083221348939));
#38937=CARTESIAN_POINT('Ctrl Pts',(0.151008425100681,-0.0315319247410302,
-0.535457342682478));
#38938=CARTESIAN_POINT('Ctrl Pts',(0.145678236122874,0.0162505661438082,
-0.532831464016017));
#38939=CARTESIAN_POINT('Ctrl Pts',(0.140348047145067,0.0640330570286466,
-0.530205585349556));
#38940=CARTESIAN_POINT('Ctrl Pts',(0.109225606117568,0.108938394047131,
-0.527579706683094));
#38941=CARTESIAN_POINT('Ctrl Pts',(0.0663550413048699,0.130702860997484,
-0.524953828016633));
#38942=CARTESIAN_POINT('Ctrl Pts',(0.0234844764921716,0.152467327947837,
-0.522327949350172));
#38943=CARTESIAN_POINT('Ctrl Pts',(-0.0311342121057257,0.151090924830058,
-0.519702070683711));
#38944=CARTESIAN_POINT('Ctrl Pts',(-0.0728541188021517,0.127194759146169,
-0.517076192017249));
#38945=CARTESIAN_POINT('Ctrl Pts',(-0.114574025498578,0.103298593462279,
-0.514450313350788));
#38946=CARTESIAN_POINT('Ctrl Pts',(-0.143395150293532,0.0568826652122784,
-0.511824434684326));
#38947=CARTESIAN_POINT('Ctrl Pts',(-0.146311843240925,0.0088923510696771,
-0.509198556017865));
#38948=CARTESIAN_POINT('Ctrl Pts',(-0.146490692924973,0.00594961672068545,
-0.50903753887334));
#38949=CARTESIAN_POINT('Ctrl Pts',(-0.146572140355928,0.00300096258414241,
-0.508876521728815));
#38950=CARTESIAN_POINT('Ctrl Pts',(-0.146558577250774,5.15455280380561E-5,
-0.508715504584291));
#38951=CARTESIAN_POINT('Origin',(0.,0.,-0.387));
#38952=CARTESIAN_POINT('',(-0.146149944725445,6.74938752725091E-5,-0.45158449541571));
#38953=CARTESIAN_POINT('',(-0.146149585450786,6.71495220561266E-5,-0.458715504584291));
#38954=CARTESIAN_POINT('',(-0.14635,-1.79227059055215E-17,-0.387));
#38955=CARTESIAN_POINT('Ctrl Pts',(-0.146149944725445,6.74938752725091E-5,
-0.45158449541571));
#38956=CARTESIAN_POINT('Ctrl Pts',(-0.146233574579168,0.0198274883748786,
-0.452655535598974));
#38957=CARTESIAN_POINT('Ctrl Pts',(-0.142499208073291,0.0395571999694397,
-0.453726575782238));
#38958=CARTESIAN_POINT('Ctrl Pts',(-0.134794490127502,0.0575905894118108,
-0.454797615965503));
#38959=CARTESIAN_POINT('Ctrl Pts',(-0.115904765165658,0.101803209405565,
-0.457423494631964));
#38960=CARTESIAN_POINT('Ctrl Pts',(-0.0731497494270609,0.135819447032232,
-0.460049373298425));
#38961=CARTESIAN_POINT('Ctrl Pts',(-0.0258228178984385,0.144289336519784,
-0.462675251964887));
#38962=CARTESIAN_POINT('Ctrl Pts',(0.0215041136301832,0.152759226007335,
-0.465301130631348));
#38963=CARTESIAN_POINT('Ctrl Pts',(0.07340296094883,0.135682767355774,-0.467927009297809));
#38964=CARTESIAN_POINT('Ctrl Pts',(0.106454157828814,0.100765782081473,
-0.470552887964271));
#38965=CARTESIAN_POINT('Ctrl Pts',(0.139505354708799,0.0658487968071709,
-0.473178766630732));
#38966=CARTESIAN_POINT('Ctrl Pts',(0.153708901150121,0.0130912849101291,
-0.475804645297193));
#38967=CARTESIAN_POINT('Ctrl Pts',(0.142655388972272,-0.0336997114928278,
-0.478430523963655));
#38968=CARTESIAN_POINT('Ctrl Pts',(0.131601876794424,-0.080490707895784,
-0.481056402630116));
#38969=CARTESIAN_POINT('Ctrl Pts',(0.0952913059974063,-0.121315188804656,
-0.483682281296577));
#38970=CARTESIAN_POINT('Ctrl Pts',(0.0501089695407642,-0.137750940937284,
-0.486308159963038));
#38971=CARTESIAN_POINT('Ctrl Pts',(0.00492663308412149,-0.154186693069913,
-0.4889340386295));
#38972=CARTESIAN_POINT('Ctrl Pts',(-0.0491274690321459,-0.146233716426298,
-0.491559917295961));
#38973=CARTESIAN_POINT('Ctrl Pts',(-0.0876612030738067,-0.117480824108352,
-0.494185795962423));
#38974=CARTESIAN_POINT('Ctrl Pts',(-0.123852202125988,-0.09047602105705,
-0.496652029113518));
#38975=CARTESIAN_POINT('Ctrl Pts',(-0.146352648855303,-0.0451235646200959,
-0.499118262264614));
#38976=CARTESIAN_POINT('Ctrl Pts',(-0.146558953229823,5.11349905732411E-5,
-0.501584495415709));
#38977=CARTESIAN_POINT('Ctrl Pts',(-0.146558577250774,5.15455280380561E-5,
-0.508715504584291));
#38978=CARTESIAN_POINT('Ctrl Pts',(-0.146350952304311,-0.0450983336056391,
-0.506250643062354));
#38979=CARTESIAN_POINT('Ctrl Pts',(-0.123878846251419,-0.0904269929973202,
-0.503785781540418));
#38980=CARTESIAN_POINT('Ctrl Pts',(-0.0877219373438008,-0.117435476278519,
-0.501320920018481));
#38981=CARTESIAN_POINT('Ctrl Pts',(-0.0492030773994497,-0.146208289448912,
-0.49869504135202));
#38982=CARTESIAN_POINT('Ctrl Pts',(0.00484690358908479,-0.154189215754497,
-0.496069162685559));
#38983=CARTESIAN_POINT('Ctrl Pts',(0.0500377315628808,-0.137776829693206,
-0.493443284019097));
#38984=CARTESIAN_POINT('Ctrl Pts',(0.0952285595366766,-0.121364443631916,
-0.490817405352636));
#38985=CARTESIAN_POINT('Ctrl Pts',(0.131560234495734,-0.08055874520375,
-0.488191526686174));
#38986=CARTESIAN_POINT('Ctrl Pts',(0.142637940141625,-0.0337734720206651,
-0.485565648019713));
#38987=CARTESIAN_POINT('Ctrl Pts',(0.153715645787515,0.0130118011624195,
-0.482939769353252));
#38988=CARTESIAN_POINT('Ctrl Pts',(0.13953938212024,0.0657766491004227,
-0.480313890686791));
#38989=CARTESIAN_POINT('Ctrl Pts',(0.106506245857298,0.100710719258534,
-0.477688012020329));
#38990=CARTESIAN_POINT('Ctrl Pts',(0.0734731095943562,0.135644789416646,
-0.475062133353868));
#38991=CARTESIAN_POINT('Ctrl Pts',(0.0215831007357463,0.152748081794866,
-0.472436254687406));
#38992=CARTESIAN_POINT('Ctrl Pts',(-0.0257482028808791,0.144302666048177,
-0.469810376020945));
#38993=CARTESIAN_POINT('Ctrl Pts',(-0.0730795064975037,0.135857250301488,
-0.467184497354483));
#38994=CARTESIAN_POINT('Ctrl Pts',(-0.115852104872144,0.101863126429891,
-0.464558618688023));
#38995=CARTESIAN_POINT('Ctrl Pts',(-0.134764688781975,0.0576602812834753,
-0.461932740021561));
#38996=CARTESIAN_POINT('Ctrl Pts',(-0.142488609406108,0.0396077894135385,
-0.460860328209138));
#38997=CARTESIAN_POINT('Ctrl Pts',(-0.14623288284995,0.0198525697897848,
-0.459787916396715));
#38998=CARTESIAN_POINT('Ctrl Pts',(-0.146149585450786,6.71495220561266E-5,
-0.458715504584291));
#38999=CARTESIAN_POINT('Origin',(0.,0.,-0.387));
#39000=CARTESIAN_POINT('',(-0.146332552080289,-0.000128504436232912,-0.401584495415709));
#39001=CARTESIAN_POINT('',(-0.146333285427459,-0.000128513713091357,-0.408715504584291));
#39002=CARTESIAN_POINT('',(-0.14635,-1.79227059055215E-17,-0.387));
#39003=CARTESIAN_POINT('Ctrl Pts',(-0.146332552080289,-0.000128504436232912,
-0.401584495415709));
#39004=CARTESIAN_POINT('Ctrl Pts',(-0.146009415250695,0.0363306749157212,
-0.403566930266872));
#39005=CARTESIAN_POINT('Ctrl Pts',(-0.132187350767056,0.0730085897307187,
-0.405549365118036));
#39006=CARTESIAN_POINT('Ctrl Pts',(-0.10751565831347,0.0996323932009806,
-0.407531799969199));
#39007=CARTESIAN_POINT('Ctrl Pts',(-0.07483621321526,0.134897550848709,
-0.41015767863566));
#39008=CARTESIAN_POINT('Ctrl Pts',(-0.0231211795979774,0.152522847755272,
-0.412783557302122));
#39009=CARTESIAN_POINT('Ctrl Pts',(0.0242928229910914,0.144554796906423,
-0.415409435968583));
#39010=CARTESIAN_POINT('Ctrl Pts',(0.0717068255801609,0.136586746057574,
-0.418035314635044));
#39011=CARTESIAN_POINT('Ctrl Pts',(0.114819797141016,0.103025347453312,
-0.420661193301506));
#39012=CARTESIAN_POINT('Ctrl Pts',(0.134176833664228,0.0590153189042965,
-0.423287071967967));
#39013=CARTESIAN_POINT('Ctrl Pts',(0.153533870187439,0.0150052903552816,
-0.425912950634428));
#39014=CARTESIAN_POINT('Ctrl Pts',(0.149134971673008,-0.0394533681384863,
-0.428538829300889));
#39015=CARTESIAN_POINT('Ctrl Pts',(0.122965158991617,-0.0797859651298404,
-0.431164707967351));
#39016=CARTESIAN_POINT('Ctrl Pts',(0.0967953463102253,-0.120118562121195,
-0.433790586633812));
#39017=CARTESIAN_POINT('Ctrl Pts',(0.0488546194618744,-0.146325097610136,
-0.436416465300273));
#39018=CARTESIAN_POINT('Ctrl Pts',(0.000776426692189965,-0.146579765722031,
-0.439042343966735));
#39019=CARTESIAN_POINT('Ctrl Pts',(-0.0473017660774945,-0.146834433833927,
-0.441668222633196));
#39020=CARTESIAN_POINT('Ctrl Pts',(-0.0955174247685125,-0.121137234568778,
-0.444294101299657));
#39021=CARTESIAN_POINT('Ctrl Pts',(-0.122113037021476,-0.0810841337557813,
-0.446919979966119));
#39022=CARTESIAN_POINT('Ctrl Pts',(-0.137860863432212,-0.057367842782088,
-0.448474818449316));
#39023=CARTESIAN_POINT('Ctrl Pts',(-0.146028538528979,-0.0286182644705103,
-0.450029656932513));
#39024=CARTESIAN_POINT('Ctrl Pts',(-0.146149944725445,6.74938752725091E-5,
-0.45158449541571));
#39025=CARTESIAN_POINT('Ctrl Pts',(-0.146149585450786,6.71495220561266E-5,
-0.458715504584291));
#39026=CARTESIAN_POINT('Ctrl Pts',(-0.146028923082908,-0.0285934771356052,
-0.457162037730253));
#39027=CARTESIAN_POINT('Ctrl Pts',(-0.137876624263401,-0.0573174757341037,
-0.455608570876215));
#39028=CARTESIAN_POINT('Ctrl Pts',(-0.122154945305088,-0.0810209770226571,
-0.454055104022177));
#39029=CARTESIAN_POINT('Ctrl Pts',(-0.0955800484733484,-0.121087823761136,
-0.451429225355716));
#39030=CARTESIAN_POINT('Ctrl Pts',(-0.0473776853648489,-0.146809950816859,
-0.448803346689255));
#39031=CARTESIAN_POINT('Ctrl Pts',(0.000700631346777343,-0.146580143593576,
-0.446177468022793));
#39032=CARTESIAN_POINT('Ctrl Pts',(0.0487789480584043,-0.146350336370292,
-0.443551589356332));
#39033=CARTESIAN_POINT('Ctrl Pts',(0.0967332183731576,-0.120168594868002,
-0.44092571068987));
#39034=CARTESIAN_POINT('Ctrl Pts',(0.122923882501041,-0.0798495365738923,
-0.438299832023409));
#39035=CARTESIAN_POINT('Ctrl Pts',(0.149114546628924,-0.0395304782797837,
-0.435673953356947));
#39036=CARTESIAN_POINT('Ctrl Pts',(0.153541604569938,0.0149258968061441,
-0.433048074690487));
#39037=CARTESIAN_POINT('Ctrl Pts',(0.134207328397462,0.0589459276338191,
-0.430422196024026));
#39038=CARTESIAN_POINT('Ctrl Pts',(0.114873052224986,0.102965958461495,
-0.427796317357564));
#39039=CARTESIAN_POINT('Ctrl Pts',(0.0717774419390191,0.136549645030918,
-0.425170438691102));
#39040=CARTESIAN_POINT('Ctrl Pts',(0.0243675672029892,0.144542211996371,
-0.422544560024641));
#39041=CARTESIAN_POINT('Ctrl Pts',(-0.0230423075330403,0.152534778961823,
-0.419918681358179));
#39042=CARTESIAN_POINT('Ctrl Pts',(-0.0747664467191323,0.134936226323305,
-0.417292802691719));
#39043=CARTESIAN_POINT('Ctrl Pts',(-0.107464121882991,0.0996879726351853,
-0.414666924025257));
#39044=CARTESIAN_POINT('Ctrl Pts',(-0.132166656965825,0.0730585190432724,
-0.412683117544935));
#39045=CARTESIAN_POINT('Ctrl Pts',(-0.146009753208469,0.0363554201922197,
-0.410699311064613));
#39046=CARTESIAN_POINT('Ctrl Pts',(-0.146333285427459,-0.000128513713091357,
-0.408715504584291));
#39047=CARTESIAN_POINT('Origin',(0.,0.,-0.387));
#39048=CARTESIAN_POINT('',(-0.146522325141606,8.10297640452141E-5,-0.35158449541571));
#39049=CARTESIAN_POINT('',(-0.146521772955861,8.13712719715056E-5,-0.358715504584291));
#39050=CARTESIAN_POINT('',(-0.14635,-1.79227059055215E-17,-0.387));
#39051=CARTESIAN_POINT('Ctrl Pts',(-0.146522325141606,8.10297640452141E-5,
-0.35158449541571));
#39052=CARTESIAN_POINT('Ctrl Pts',(-0.146555231621681,0.00499241344169051,
-0.35185244626831));
#39053=CARTESIAN_POINT('Ctrl Pts',(-0.146329339568258,0.00990073582968819,
-0.352120397120911));
#39054=CARTESIAN_POINT('Ctrl Pts',(-0.145834593749664,0.0147818071765353,
-0.352388347973511));
#39055=CARTESIAN_POINT('Ctrl Pts',(-0.140986158009458,0.0626155833887401,
-0.355014226639972));
#39056=CARTESIAN_POINT('Ctrl Pts',(-0.110317787182484,0.107832248722449,
-0.357640105306433));
#39057=CARTESIAN_POINT('Ctrl Pts',(-0.0676687085120385,0.130027598785206,
-0.360265983972895));
#39058=CARTESIAN_POINT('Ctrl Pts',(-0.0250196298415937,0.152222948847963,
-0.362891862639356));
#39059=CARTESIAN_POINT('Ctrl Pts',(0.0296101566723226,0.151396983639769,
-0.365517741305818));
#39060=CARTESIAN_POINT('Ctrl Pts',(0.071568737366472,0.127922423324852,
-0.368143619972279));
#39061=CARTESIAN_POINT('Ctrl Pts',(0.113527318060621,0.104447863009936,
-0.37076949863874));
#39062=CARTESIAN_POINT('Ctrl Pts',(0.142814692935004,0.0583247075882974,
-0.373395377305201));
#39063=CARTESIAN_POINT('Ctrl Pts',(0.146214814794519,0.0103662187965668,
-0.376021255971663));
#39064=CARTESIAN_POINT('Ctrl Pts',(0.149614936654034,-0.0375922699951634,
-0.378647134638124));
#39065=CARTESIAN_POINT('Ctrl Pts',(0.127127805498682,-0.0873860921569855,
-0.381273013304586));
#39066=CARTESIAN_POINT('Ctrl Pts',(0.0889008308489892,-0.116545582635693,
-0.383898891971047));
#39067=CARTESIAN_POINT('Ctrl Pts',(0.0506738561992962,-0.145705073114401,
-0.386524770637508));
#39068=CARTESIAN_POINT('Ctrl Pts',(-0.00329296194473747,-0.154230231909994,
-0.38915064930397));
#39069=CARTESIAN_POINT('Ctrl Pts',(-0.0486468770969522,-0.138274046394281,
-0.391776527970431));
#39070=CARTESIAN_POINT('Ctrl Pts',(-0.0940007922491663,-0.122317860878569,
-0.394402406636892));
#39071=CARTESIAN_POINT('Ctrl Pts',(-0.130741804409562,-0.0818803310515519,
-0.397028285303353));
#39072=CARTESIAN_POINT('Ctrl Pts',(-0.14229038220019,-0.0352090569435971,
-0.399654163969815));
#39073=CARTESIAN_POINT('Ctrl Pts',(-0.145120239135235,-0.0237727544744814,
-0.400297607785113));
#39074=CARTESIAN_POINT('Ctrl Pts',(-0.146437433405582,-0.0119621510506967,
-0.400941051600411));
#39075=CARTESIAN_POINT('Ctrl Pts',(-0.146332552080289,-0.000128504436232912,
-0.401584495415709));
#39076=CARTESIAN_POINT('Ctrl Pts',(-0.146333285427459,-0.000128513713091357,
-0.408715504584291));
#39077=CARTESIAN_POINT('Ctrl Pts',(-0.146437998785942,-0.0119367820265121,
-0.408073432398151));
#39078=CARTESIAN_POINT('Ctrl Pts',(-0.145126488659511,-0.0237220920150426,
-0.407431360212012));
#39079=CARTESIAN_POINT('Ctrl Pts',(-0.142308565599436,-0.0351354740572363,
-0.406789288025873));
#39080=CARTESIAN_POINT('Ctrl Pts',(-0.130784123010399,-0.0818127123238171,
-0.404163409359411));
#39081=CARTESIAN_POINT('Ctrl Pts',(-0.0940640266907015,-0.122269234119258,
-0.401537530692951));
#39082=CARTESIAN_POINT('Ctrl Pts',(-0.0487183696599885,-0.13824886921009,
-0.398911652026489));
#39083=CARTESIAN_POINT('Ctrl Pts',(-0.00337271262927494,-0.154228504300922,
-0.396285773360028));
#39084=CARTESIAN_POINT('Ctrl Pts',(0.0505985051124538,-0.145731252687143,
-0.393659894693567));
#39085=CARTESIAN_POINT('Ctrl Pts',(0.0888405517426594,-0.116591533767489,
-0.391034016027105));
#39086=CARTESIAN_POINT('Ctrl Pts',(0.127082598372864,-0.087451814847836,
-0.388408137360644));
#39087=CARTESIAN_POINT('Ctrl Pts',(0.149595473891547,-0.0376696286223078,
-0.385782258694183));
#39088=CARTESIAN_POINT('Ctrl Pts',(0.146220151529374,0.0102906106195329,
-0.383156380027721));
#39089=CARTESIAN_POINT('Ctrl Pts',(0.142844829167201,0.0582508498613742,
-0.38053050136126));
#39090=CARTESIAN_POINT('Ctrl Pts',(0.113581308924171,0.104389142119528,
-0.377904622694799));
#39091=CARTESIAN_POINT('Ctrl Pts',(0.0716348734958325,0.127885395098236,
-0.375278744028337));
#39092=CARTESIAN_POINT('Ctrl Pts',(0.0296884380674942,0.151381648076943,
-0.372652865361876));
#39093=CARTESIAN_POINT('Ctrl Pts',(-0.0249409125461535,0.152235861776206,
-0.370026986695415));
#39094=CARTESIAN_POINT('Ctrl Pts',(-0.0676014613836439,0.130062568785149,
-0.367401108028953));
#39095=CARTESIAN_POINT('Ctrl Pts',(-0.110262010221135,0.107889275794091,
-0.364775229362492));
#39096=CARTESIAN_POINT('Ctrl Pts',(-0.140953757282468,0.062688476112713,
-0.362149350696031));
#39097=CARTESIAN_POINT('Ctrl Pts',(-0.145826926703387,0.0148572146932371,
-0.359523472029569));
#39098=CARTESIAN_POINT('Ctrl Pts',(-0.146326741907813,0.00995141527618409,
-0.35925414954781));
#39099=CARTESIAN_POINT('Ctrl Pts',(-0.146554958079519,0.00501794466540278,
-0.35898482706605));
#39100=CARTESIAN_POINT('Ctrl Pts',(-0.146521772955861,8.13712719715056E-5,
-0.358715504584291));
#39101=CARTESIAN_POINT('Origin',(0.,0.,-0.387));
#39102=CARTESIAN_POINT('',(-0.146127820803365,3.85940253507244E-5,-0.301584495415709));
#39103=CARTESIAN_POINT('',(-0.14612761578604,3.82095679274467E-5,-0.308715504584291));
#39104=CARTESIAN_POINT('',(-0.14635,-1.79227059055215E-17,-0.387));
#39105=CARTESIAN_POINT('Ctrl Pts',(-0.146127820803365,3.85940253507244E-5,
-0.301584495415709));
#39106=CARTESIAN_POINT('Ctrl Pts',(-0.146180003049472,0.0218050073068917,
-0.302763840936209));
#39107=CARTESIAN_POINT('Ctrl Pts',(-0.141618666722499,0.0435506356661818,
-0.303943186456708));
#39108=CARTESIAN_POINT('Ctrl Pts',(-0.132331368584888,0.0630447416204224,
-0.305122531977207));
#39109=CARTESIAN_POINT('Ctrl Pts',(-0.111652680596745,0.106449457250585,
-0.307748410643668));
#39110=CARTESIAN_POINT('Ctrl Pts',(-0.067544796154219,0.138692135847224,
-0.31037428931013));
#39111=CARTESIAN_POINT('Ctrl Pts',(-0.0199115777567349,0.145223137374079,
-0.313000167976591));
#39112=CARTESIAN_POINT('Ctrl Pts',(0.02772164064075,0.151754138900935,-0.315626046643052));
#39113=CARTESIAN_POINT('Ctrl Pts',(0.0788801929931927,0.132573463358006,
-0.318251925309514));
#39114=CARTESIAN_POINT('Ctrl Pts',(0.110478574190537,0.0963364687040155,
-0.320877803975975));
#39115=CARTESIAN_POINT('Ctrl Pts',(0.142076955387881,0.0600994740500249,
-0.323503682642436));
#39116=CARTESIAN_POINT('Ctrl Pts',(0.154115165430126,0.00680616028497251,
-0.326129561308898));
#39117=CARTESIAN_POINT('Ctrl Pts',(0.141160913005902,-0.0394946476990751,
-0.328755439975359));
#39118=CARTESIAN_POINT('Ctrl Pts',(0.128206660581679,-0.085795455683122,
-0.33138131864182));
#39119=CARTESIAN_POINT('Ctrl Pts',(0.0902599456909862,-0.125103757886164,
-0.334007197308282));
#39120=CARTESIAN_POINT('Ctrl Pts',(0.0444443779794659,-0.139681522842329,
-0.336633075974743));
#39121=CARTESIAN_POINT('Ctrl Pts',(-0.00137118973205505,-0.154259287798493,
-0.339258954641204));
#39122=CARTESIAN_POINT('Ctrl Pts',(-0.0550556102644042,-0.14410651550778,
-0.341884833307666));
#39123=CARTESIAN_POINT('Ctrl Pts',(-0.0923835702038583,-0.113804685817072,
-0.344510711974127));
#39124=CARTESIAN_POINT('Ctrl Pts',(-0.125902497068263,-0.086594926298794,
-0.346868639787988));
#39125=CARTESIAN_POINT('Ctrl Pts',(-0.146232752991076,-0.0431384191224556,
-0.349226567601849));
#39126=CARTESIAN_POINT('Ctrl Pts',(-0.146522325141606,8.10297640452141E-5,
-0.35158449541571));
#39127=CARTESIAN_POINT('Ctrl Pts',(-0.146521772955861,8.13712719715056E-5,
-0.358715504584291));
#39128=CARTESIAN_POINT('Ctrl Pts',(-0.146231405037506,-0.0431133612491548,
-0.356358948399589));
#39129=CARTESIAN_POINT('Ctrl Pts',(-0.12592776423548,-0.0865456474357522,
-0.354002392214887));
#39130=CARTESIAN_POINT('Ctrl Pts',(-0.0924424028114175,-0.113756896681685,
-0.351645836030186));
#39131=CARTESIAN_POINT('Ctrl Pts',(-0.0551301177180251,-0.144078023479557,
-0.349019957363724));
#39132=CARTESIAN_POINT('Ctrl Pts',(-0.00145095575073629,-0.154258553917727,
-0.346394078697263));
#39133=CARTESIAN_POINT('Ctrl Pts',(0.0443721426256257,-0.139704482172216,
-0.343768200030801));
#39134=CARTESIAN_POINT('Ctrl Pts',(0.090195241001987,-0.125150410426704,
-0.34114232136434));
#39135=CARTESIAN_POINT('Ctrl Pts',(0.128162275787421,-0.0858617364975109,
-0.338516442697879));
#39136=CARTESIAN_POINT('Ctrl Pts',(0.141140467901028,-0.0395676345119932,
-0.335890564031418));
#39137=CARTESIAN_POINT('Ctrl Pts',(0.154118660014635,0.00672646747352509,
-0.333264685364956));
#39138=CARTESIAN_POINT('Ctrl Pts',(0.142108009456413,0.0600259975153678,
-0.330638806698495));
#39139=CARTESIAN_POINT('Ctrl Pts',(0.110528371208319,0.0962793256012516,
-0.328012928032033));
#39140=CARTESIAN_POINT('Ctrl Pts',(0.0789487329602256,0.132532653687135,
-0.325387049365572));
#39141=CARTESIAN_POINT('Ctrl Pts',(0.0278001070222592,0.15173977981706,
-0.322761170699111));
#39142=CARTESIAN_POINT('Ctrl Pts',(-0.0198364808304775,0.145233410097187,
-0.32013529203265));
#39143=CARTESIAN_POINT('Ctrl Pts',(-0.0674730686832152,0.138727040377315,
-0.317509413366188));
#39144=CARTESIAN_POINT('Ctrl Pts',(-0.111597618450724,0.106507174807645,
-0.314883534699727));
#39145=CARTESIAN_POINT('Ctrl Pts',(-0.132298747337815,0.0631131589531134,
-0.312257656033265));
#39146=CARTESIAN_POINT('Ctrl Pts',(-0.141606937471067,0.0436011916385575,
-0.311076938883607));
#39147=CARTESIAN_POINT('Ctrl Pts',(-0.146179334127518,0.0218300125590762,
-0.309896221733949));
#39148=CARTESIAN_POINT('Ctrl Pts',(-0.14612761578604,3.82095679274467E-5,
-0.308715504584291));
#39149=CARTESIAN_POINT('Origin',(0.,0.,-0.387));
#39150=CARTESIAN_POINT('',(-0.146391321186674,-0.000125022356020285,-0.251584495415709));
#39151=CARTESIAN_POINT('',(-0.146392060940901,-0.000124923264760741,-0.258715504584291));
#39152=CARTESIAN_POINT('',(-0.14635,-1.79227059055215E-17,-0.387));
#39153=CARTESIAN_POINT('Ctrl Pts',(-0.146391321186674,-0.000125022356020285,
-0.251584495415709));
#39154=CARTESIAN_POINT('Ctrl Pts',(-0.146046214648355,0.038286396641969,
-0.253675235604107));
#39155=CARTESIAN_POINT('Ctrl Pts',(-0.130503182125338,0.0769451781813335,
-0.255765975792505));
#39156=CARTESIAN_POINT('Ctrl Pts',(-0.103359175644828,0.103938016950627,
-0.257856715980903));
#39157=CARTESIAN_POINT('Ctrl Pts',(-0.0692674850871064,0.13783984744341,
-0.260482594647365));
#39158=CARTESIAN_POINT('Ctrl Pts',(-0.0168761089937022,0.153339508863856,
-0.263108473313826));
#39159=CARTESIAN_POINT('Ctrl Pts',(0.0301731307904698,0.143442715868794,
-0.265734351980287));
#39160=CARTESIAN_POINT('Ctrl Pts',(0.0772223705746437,0.133545922873731,
-0.268360230646749));
#39161=CARTESIAN_POINT('Ctrl Pts',(0.118929474049585,0.0982526754631585,
-0.27098610931321));
#39162=CARTESIAN_POINT('Ctrl Pts',(0.136473940905855,0.0534891952748376,
-0.273611987979671));
#39163=CARTESIAN_POINT('Ctrl Pts',(0.154018407762125,0.00872571508651834,
-0.276237866646132));
#39164=CARTESIAN_POINT('Ctrl Pts',(0.147400237999727,-0.0455079978795489,
-0.278863745312594));
#39165=CARTESIAN_POINT('Ctrl Pts',(0.119605907678566,-0.0847387597615798,
-0.281489623979055));
#39166=CARTESIAN_POINT('Ctrl Pts',(0.0918115773574051,-0.123969521643612,
-0.284115502645516));
#39167=CARTESIAN_POINT('Ctrl Pts',(0.0428410864774815,-0.148197332441607,
-0.286741381311978));
#39168=CARTESIAN_POINT('Ctrl Pts',(-0.00520743150216466,-0.146489293856856,
-0.289367259978439));
#39169=CARTESIAN_POINT('Ctrl Pts',(-0.0532559494818108,-0.144781255272105,
-0.291993138644901));
#39170=CARTESIAN_POINT('Ctrl Pts',(-0.100382494561179,-0.117137367304608,
-0.294619017311362));
#39171=CARTESIAN_POINT('Ctrl Pts',(-0.125321021333984,-0.0760320469890165,
-0.297244895977823));
#39172=CARTESIAN_POINT('Ctrl Pts',(-0.139059053501684,-0.0533881186646286,
-0.298691429123785));
#39173=CARTESIAN_POINT('Ctrl Pts',(-0.146063816364198,-0.0266591274932147,
-0.300137962269747));
#39174=CARTESIAN_POINT('Ctrl Pts',(-0.146127820803365,3.85940253507244E-5,
-0.301584495415709));
#39175=CARTESIAN_POINT('Ctrl Pts',(-0.14612761578604,3.82095679274467E-5,
-0.308715504584291));
#39176=CARTESIAN_POINT('Ctrl Pts',(-0.146064314124979,-0.0266342877983396,
-0.307270343067488));
#39177=CARTESIAN_POINT('Ctrl Pts',(-0.139073622120044,-0.0533376818630241,
-0.305825181550685));
#39178=CARTESIAN_POINT('Ctrl Pts',(-0.125360316707312,-0.0759672322467926,
-0.304380020033882));
#39179=CARTESIAN_POINT('Ctrl Pts',(-0.100443049183043,-0.117085441452778,
-0.30175414136742));
#39180=CARTESIAN_POINT('Ctrl Pts',(-0.0533308061278312,-0.144753693725355,
-0.299128262700959));
#39181=CARTESIAN_POINT('Ctrl Pts',(-0.0052831791013535,-0.146486577537938,
-0.296502384034497));
#39182=CARTESIAN_POINT('Ctrl Pts',(0.0427644479251232,-0.14821946135052,
-0.293876505368036));
#39183=CARTESIAN_POINT('Ctrl Pts',(0.0917474589228652,-0.124016976703108,
-0.291250626701575));
#39184=CARTESIAN_POINT('Ctrl Pts',(0.119562070678756,-0.0848005933658808,
-0.288624748035114));
#39185=CARTESIAN_POINT('Ctrl Pts',(0.147376682434647,-0.045584210028653,
-0.285998869368652));
#39186=CARTESIAN_POINT('Ctrl Pts',(0.154022894948687,0.00864607199839097,
-0.283372990702191));
#39187=CARTESIAN_POINT('Ctrl Pts',(0.136501577754921,0.0534186170788067,
-0.280747112035729));
#39188=CARTESIAN_POINT('Ctrl Pts',(0.118980260561155,0.0981911621592217,
-0.278121233369268));
#39189=CARTESIAN_POINT('Ctrl Pts',(0.0772914136595841,0.133505970293009,
-0.275495354702807));
#39190=CARTESIAN_POINT('Ctrl Pts',(0.0302472990068507,0.143427090477993,
-0.272869476036346));
#39191=CARTESIAN_POINT('Ctrl Pts',(-0.0167968156458838,0.153348210662977,
-0.270243597369885));
#39192=CARTESIAN_POINT('Ctrl Pts',(-0.0691961980497802,0.137875642899156,
-0.267617718703423));
#39193=CARTESIAN_POINT('Ctrl Pts',(-0.103305413480267,0.103991446407277,
-0.264991840036961));
#39194=CARTESIAN_POINT('Ctrl Pts',(-0.130481190335898,0.0769949485056395,
-0.262899728219404));
#39195=CARTESIAN_POINT('Ctrl Pts',(-0.146046808768056,0.0383111911777933,
-0.260807616401848));
#39196=CARTESIAN_POINT('Ctrl Pts',(-0.146392060940901,-0.000124923264760741,
-0.258715504584291));
#39197=CARTESIAN_POINT('Origin',(0.,0.,-0.387));
#39198=CARTESIAN_POINT('',(-0.146474049564045,0.000104587793401157,-0.201584495415709));
#39199=CARTESIAN_POINT('',(-0.146473378794998,0.000104839022694492,-0.208715504584291));
#39200=CARTESIAN_POINT('',(-0.14635,-1.79227059055215E-17,-0.387));
#39201=CARTESIAN_POINT('Ctrl Pts',(-0.146474049564045,0.000104587793401157,
-0.201584495415709));
#39202=CARTESIAN_POINT('Ctrl Pts',(-0.146530019115592,0.00700710845801674,
-0.201960751605545));
#39203=CARTESIAN_POINT('Ctrl Pts',(-0.14608358854416,0.0139023584599612,
-0.20233700779538));
#39204=CARTESIAN_POINT('Ctrl Pts',(-0.145109674382301,0.0207222815519516,
-0.202713263985215));
#39205=CARTESIAN_POINT('Ctrl Pts',(-0.138312761827298,0.0683182840575807,
-0.205339142651677));
#39206=CARTESIAN_POINT('Ctrl Pts',(-0.105824260807261,0.11224541798416,
-0.207965021318138));
#39207=CARTESIAN_POINT('Ctrl Pts',(-0.0623047396710364,0.132681385187423,
-0.210590899984599));
#39208=CARTESIAN_POINT('Ctrl Pts',(-0.0187852185348116,0.153117352390686,
-0.213216778651061));
#39209=CARTESIAN_POINT('Ctrl Pts',(0.0357653227176007,0.150062152870633,
-0.215842657317522));
#39210=CARTESIAN_POINT('Ctrl Pts',(0.0767307301398749,0.124894457881073,
-0.218468535983983));
#39211=CARTESIAN_POINT('Ctrl Pts',(0.117696137562149,0.0997267628915141,
-0.221094414650445));
#39212=CARTESIAN_POINT('Ctrl Pts',(0.145076411154285,0.0524465724324491,
-0.223720293316906));
#39213=CARTESIAN_POINT('Ctrl Pts',(0.146516090957969,0.00438926499935377,
-0.226346171983367));
#39214=CARTESIAN_POINT('Ctrl Pts',(0.147955770761653,-0.043668042433743,
-0.228972050649829));
#39215=CARTESIAN_POINT('Ctrl Pts',(0.123454856776884,-0.0925024668408702,
-0.23159792931629));
#39216=CARTESIAN_POINT('Ctrl Pts',(0.08406948621946,-0.120077275305623,
-0.234223807982751));
#39217=CARTESIAN_POINT('Ctrl Pts',(0.0446841156620375,-0.147652083770375,
-0.236849686649213));
#39218=CARTESIAN_POINT('Ctrl Pts',(-0.00958571146803889,-0.153967276292754,
-0.239475565315674));
#39219=CARTESIAN_POINT('Ctrl Pts',(-0.0542505146411621,-0.136173096530155,
-0.242101443982135));
#39220=CARTESIAN_POINT('Ctrl Pts',(-0.0989153178142867,-0.118378916767556,
-0.244727322648597));
#39221=CARTESIAN_POINT('Ctrl Pts',(-0.133975097030458,-0.0764753647199769,
-0.247353201315058));
#39222=CARTESIAN_POINT('Ctrl Pts',(-0.143608984127524,-0.029371588913627,
-0.249979079981519));
#39223=CARTESIAN_POINT('Ctrl Pts',(-0.145572313105669,-0.0197721191369005,
-0.250514218459583));
#39224=CARTESIAN_POINT('Ctrl Pts',(-0.146479653437955,-0.00995667356591409,
-0.251049356937646));
#39225=CARTESIAN_POINT('Ctrl Pts',(-0.146391321186674,-0.000125022356020285,
-0.251584495415709));
#39226=CARTESIAN_POINT('Ctrl Pts',(-0.146392060940901,-0.000124923264760741,
-0.258715504584291));
#39227=CARTESIAN_POINT('Ctrl Pts',(-0.146480146177469,-0.00993124600428374,
-0.258181737735387));
#39228=CARTESIAN_POINT('Ctrl Pts',(-0.145577494117458,-0.019721448958086,
-0.257647970886482));
#39229=CARTESIAN_POINT('Ctrl Pts',(-0.143624148806805,-0.029297325128882,
-0.257114204037578));
#39230=CARTESIAN_POINT('Ctrl Pts',(-0.134014620245779,-0.0764060749532282,
-0.254488325371117));
#39231=CARTESIAN_POINT('Ctrl Pts',(-0.0989765146666498,-0.118327749381984,
-0.251862446704655));
#39232=CARTESIAN_POINT('Ctrl Pts',(-0.0543209199166082,-0.13614502208891,
-0.249236568038194));
#39233=CARTESIAN_POINT('Ctrl Pts',(-0.00966532516656721,-0.153962294795835,
-0.246610689371732));
#39234=CARTESIAN_POINT('Ctrl Pts',(0.0446077587543858,-0.14767516578093,
-0.243984810705271));
#39235=CARTESIAN_POINT('Ctrl Pts',(0.0840073816803498,-0.120120727618016,
-0.24135893203881));
#39236=CARTESIAN_POINT('Ctrl Pts',(0.123407004606315,-0.0925662894551019,
-0.238733053372349));
#39237=CARTESIAN_POINT('Ctrl Pts',(0.14793316653729,-0.0437445421441763,
-0.236107174705887));
#39238=CARTESIAN_POINT('Ctrl Pts',(0.146518337011597,0.0043135019958444,
-0.233481296039426));
#39239=CARTESIAN_POINT('Ctrl Pts',(0.145103507485905,0.0523715461358634,
-0.230855417372964));
#39240=CARTESIAN_POINT('Ctrl Pts',(0.117747686503548,0.0996658871049781,
-0.228229538706503));
#39241=CARTESIAN_POINT('Ctrl Pts',(0.076795299696999,0.124854760920646,
-0.225603660040042));
#39242=CARTESIAN_POINT('Ctrl Pts',(0.0358429128904488,0.150043634736315,
-0.222977781373581));
#39243=CARTESIAN_POINT('Ctrl Pts',(-0.0187060397402936,0.153127041398535,
-0.220351902707119));
#39244=CARTESIAN_POINT('Ctrl Pts',(-0.0622361211473401,0.132713581088084,
-0.217726024040658));
#39245=CARTESIAN_POINT('Ctrl Pts',(-0.105766202554386,0.112300120777634,
-0.215100145374196));
#39246=CARTESIAN_POINT('Ctrl Pts',(-0.138277412737736,0.0683897934945145,
-0.212474266707735));
#39247=CARTESIAN_POINT('Ctrl Pts',(-0.145098935695872,0.0207973132741649,
-0.209848388041274));
#39248=CARTESIAN_POINT('Ctrl Pts',(-0.146079939452749,0.0139530349243349,
-0.20947076022228));
#39249=CARTESIAN_POINT('Ctrl Pts',(-0.146529646082409,0.00703260472180356,
-0.209093132403285));
#39250=CARTESIAN_POINT('Ctrl Pts',(-0.146473378794998,0.000104839022694492,
-0.208715504584291));
#39251=CARTESIAN_POINT('Origin',(0.,0.,-0.387));
#39252=CARTESIAN_POINT('',(-0.146118283015211,7.41336224649447E-6,-0.151584495415709));
#39253=CARTESIAN_POINT('',(-0.146118240456221,7.01092482352256E-6,-0.158715504584291));
#39254=CARTESIAN_POINT('',(-0.14635,-1.79227059055215E-17,-0.387));
#39255=CARTESIAN_POINT('Ctrl Pts',(-0.146118283015211,7.41336224649447E-6,
-0.151584495415709));
#39256=CARTESIAN_POINT('Ctrl Pts',(-0.14612918343829,0.0237766293842829,
-0.152872146273443));
#39257=CARTESIAN_POINT('Ctrl Pts',(-0.14064821628497,0.0475411064603244,
-0.154159797131177));
#39258=CARTESIAN_POINT('Ctrl Pts',(-0.129647667122561,0.0683938057602947,
-0.155447447988912));
#39259=CARTESIAN_POINT('Ctrl Pts',(-0.107214484096722,0.110918266409727,
-0.158073326655373));
#39260=CARTESIAN_POINT('Ctrl Pts',(-0.061827254568182,0.141333643007611,
-0.160699205321834));
#39261=CARTESIAN_POINT('Ctrl Pts',(-0.0139671480261764,0.14591487057081,
-0.163325083988295));
#39262=CARTESIAN_POINT('Ctrl Pts',(0.0338929585158298,0.150496098134008,
-0.165950962654757));
#39263=CARTESIAN_POINT('Ctrl Pts',(0.084225942071302,0.129243176662519,
-0.168576841321218));
#39264=CARTESIAN_POINT('Ctrl Pts',(0.114318837396064,0.0917465748018712,
-0.17120271998768));
#39265=CARTESIAN_POINT('Ctrl Pts',(0.144411732720825,0.0542499729412243,
-0.173828598654141));
#39266=CARTESIAN_POINT('Ctrl Pts',(0.154264539814876,0.000509690691419144,
-0.176454477320602));
#39267=CARTESIAN_POINT('Ctrl Pts',(0.139431140093356,-0.0452237513755338,
-0.179080355987063));
#39268=CARTESIAN_POINT('Ctrl Pts',(0.124597740371835,-0.0909571934424881,
-0.181706234653525));
#39269=CARTESIAN_POINT('Ctrl Pts',(0.0850781338347429,-0.128683795326589,
-0.184332113319986));
#39270=CARTESIAN_POINT('Ctrl Pts',(0.0387057034970471,-0.141379273920697,
-0.186957991986448));
#39271=CARTESIAN_POINT('Ctrl Pts',(-0.00766672684064738,-0.154074752514805,
-0.189583870652909));
#39272=CARTESIAN_POINT('Ctrl Pts',(-0.0608919809789443,-0.141739107818921,
-0.19220974931937));
#39273=CARTESIAN_POINT('Ctrl Pts',(-0.0969519460031083,-0.10993884992864,
-0.194835627985831));
#39274=CARTESIAN_POINT('Ctrl Pts',(-0.127844960543657,-0.0826951787620337,
-0.197085250462457));
#39275=CARTESIAN_POINT('Ctrl Pts',(-0.146139409591153,-0.0411653395911477,
-0.199334872939083));
#39276=CARTESIAN_POINT('Ctrl Pts',(-0.146474049564045,0.000104587793401157,
-0.201584495415709));
#39277=CARTESIAN_POINT('Ctrl Pts',(-0.146473378794998,0.000104839022694492,
-0.208715504584291));
#39278=CARTESIAN_POINT('Ctrl Pts',(-0.146138384998877,-0.0411404144269961,
-0.206467253736824));
#39279=CARTESIAN_POINT('Ctrl Pts',(-0.127868873563498,-0.0826456784984334,
-0.204219002889357));
#39280=CARTESIAN_POINT('Ctrl Pts',(-0.0970087788541284,-0.109888699169191,
-0.20197075204189));
#39281=CARTESIAN_POINT('Ctrl Pts',(-0.0609652633213293,-0.141707598234614,
-0.199344873375428));
#39282=CARTESIAN_POINT('Ctrl Pts',(-0.00774639652281044,-0.154070763207882,
-0.196718994708967));
#39283=CARTESIAN_POINT('Ctrl Pts',(0.0386325911211531,-0.141399265509641,
-0.194093116042506));
#39284=CARTESIAN_POINT('Ctrl Pts',(0.085011578765118,-0.128727767811399,
-0.191467237376045));
#39285=CARTESIAN_POINT('Ctrl Pts',(0.124550687254527,-0.091021607441645,
-0.188841358709583));
#39286=CARTESIAN_POINT('Ctrl Pts',(0.139407732894378,-0.0452958428992574,
-0.186215480043122));
#39287=CARTESIAN_POINT('Ctrl Pts',(0.154264778534229,0.000429921643130132,
-0.183589601376661));
#39288=CARTESIAN_POINT('Ctrl Pts',(0.144439761324521,0.0541752903581515,
-0.180963722710199));
#39289=CARTESIAN_POINT('Ctrl Pts',(0.11436626020644,0.0916874468314653,
-0.178337844043738));
#39290=CARTESIAN_POINT('Ctrl Pts',(0.0842927590883588,0.129199603304779,
-0.175711965377277));
#39291=CARTESIAN_POINT('Ctrl Pts',(0.0339707740619053,0.150478547536385,
-0.173086086710815));
#39292=CARTESIAN_POINT('Ctrl Pts',(-0.0138916940039819,0.145922069057284,
-0.170460208044354));
#39293=CARTESIAN_POINT('Ctrl Pts',(-0.0617541620698691,0.141365590578183,
-0.167834329377893));
#39294=CARTESIAN_POINT('Ctrl Pts',(-0.10715711317519,0.110973689388375,
-0.165208450711431));
#39295=CARTESIAN_POINT('Ctrl Pts',(-0.129612281041003,0.0684608350966334,
-0.16258257204497));
#39296=CARTESIAN_POINT('Ctrl Pts',(-0.140635340368035,0.0475916205879853,
-0.161293549558077));
#39297=CARTESIAN_POINT('Ctrl Pts',(-0.146128561593049,0.0238015614994364,
-0.160004527071184));
#39298=CARTESIAN_POINT('Ctrl Pts',(-0.146118240456221,7.01092482352256E-6,
-0.158715504584291));
#39299=CARTESIAN_POINT('Origin',(0.,0.,-0.387));
#39300=CARTESIAN_POINT('',(-0.146448857461917,-0.000112937673885413,-0.101584495415709));
#39301=CARTESIAN_POINT('',(-0.146449480434,-0.000112796118272305,-0.108715504584291));
#39302=CARTESIAN_POINT('',(-0.14635,-1.79227059055215E-17,-0.387));
#39303=CARTESIAN_POINT('Ctrl Pts',(-0.146448857461917,-0.000112937673885413,
-0.101584495415709));
#39304=CARTESIAN_POINT('Ctrl Pts',(-0.146104431800015,0.0402472859926994,
-0.103783540941342));
#39305=CARTESIAN_POINT('Ctrl Pts',(-0.128715625084515,0.0808682927490122,
-0.105982586466975));
#39306=CARTESIAN_POINT('Ctrl Pts',(-0.0990303696629292,0.10807035631605,
-0.108181631992607));
#39307=CARTESIAN_POINT('Ctrl Pts',(-0.0635832277045705,0.140552320682775,
-0.110807510659069));
#39308=CARTESIAN_POINT('Ctrl Pts',(-0.0106029105929107,0.153900575233485,
-0.11343338932553));
#39309=CARTESIAN_POINT('Ctrl Pts',(0.0360031244180305,0.142091552039598,
-0.116059267991992));
#39310=CARTESIAN_POINT('Ctrl Pts',(0.082609159428971,0.130282528845712,
-0.118685146658453));
#39311=CARTESIAN_POINT('Ctrl Pts',(0.122840912339193,0.0933162279072309,
-0.121311025324914));
#39312=CARTESIAN_POINT('Ctrl Pts',(0.138543574148993,0.0478739029189084,
-0.123936903991376));
#39313=CARTESIAN_POINT('Ctrl Pts',(0.154246235958793,0.00243157793058653,
-0.126562782657837));
#39314=CARTESIAN_POINT('Ctrl Pts',(0.145419806668172,-0.0514867711075763,
-0.129188661324298));
#39315=CARTESIAN_POINT('Ctrl Pts',(0.116047283516059,-0.0895503010832982,
-0.13181453999076));
#39316=CARTESIAN_POINT('Ctrl Pts',(0.0866747603639465,-0.127613831059021,
-0.134440418657221));
#39317=CARTESIAN_POINT('Ctrl Pts',(0.0367561433503418,-0.149822541972302,
-0.137066297323682));
#39318=CARTESIAN_POINT('Ctrl Pts',(-0.011182606745029,-0.146154645996528,
-0.139692175990144));
#39319=CARTESIAN_POINT('Ctrl Pts',(-0.0591213568403991,-0.142486750020755,
-0.142318054656605));
#39320=CARTESIAN_POINT('Ctrl Pts',(-0.105080240017535,-0.112942247155927,
-0.144943933323066));
#39321=CARTESIAN_POINT('Ctrl Pts',(-0.128320113344536,-0.070853223373023,
-0.147569811989528));
#39322=CARTESIAN_POINT('Ctrl Pts',(-0.140163861174438,-0.0494033739234423,
-0.148908039798255));
#39323=CARTESIAN_POINT('Ctrl Pts',(-0.14610695444023,-0.0246954210134512,
-0.150246267606982));
#39324=CARTESIAN_POINT('Ctrl Pts',(-0.146118283015211,7.41336224649447E-6,
-0.151584495415709));
#39325=CARTESIAN_POINT('Ctrl Pts',(-0.146118240456221,7.01092482352256E-6,
-0.158715504584291));
#39326=CARTESIAN_POINT('Ctrl Pts',(-0.146107536317474,-0.0246705197615437,
-0.157378648404722));
#39327=CARTESIAN_POINT('Ctrl Pts',(-0.140177254795957,-0.0493528814635679,
-0.156041792225154));
#39328=CARTESIAN_POINT('Ctrl Pts',(-0.128356728993014,-0.0707868597717533,
-0.154704936045586));
#39329=CARTESIAN_POINT('Ctrl Pts',(-0.105138624452908,-0.11288789295472,
-0.152079057379125));
#39330=CARTESIAN_POINT('Ctrl Pts',(-0.0591950307463908,-0.142456151926979,
-0.149453178712664));
#39331=CARTESIAN_POINT('Ctrl Pts',(-0.0112581828339444,-0.146148837901321,
-0.146827300046202));
#39332=CARTESIAN_POINT('Ctrl Pts',(0.0366786650785026,-0.149841523875664,
-0.144201421379741));
#39333=CARTESIAN_POINT('Ctrl Pts',(0.0866087671968788,-0.12765863685209,
-0.141575542713279));
#39334=CARTESIAN_POINT('Ctrl Pts',(0.116000963822744,-0.0896102977953412,
-0.138949664046818));
#39335=CARTESIAN_POINT('Ctrl Pts',(0.145393160448608,-0.0515619587385927,
-0.136323785380357));
#39336=CARTESIAN_POINT('Ctrl Pts',(0.154247451581962,0.00235183235133025,
-0.133697906713896));
#39337=CARTESIAN_POINT('Ctrl Pts',(0.138568298030551,0.0478022630729415,
-0.131072028047434));
#39338=CARTESIAN_POINT('Ctrl Pts',(0.122889144479139,0.0932526937945534,
-0.128446149380973));
#39339=CARTESIAN_POINT('Ctrl Pts',(0.0826765462429627,0.130239764147853,
-0.125820270714511));
#39340=CARTESIAN_POINT('Ctrl Pts',(0.0360766101420983,0.142072897713786,
-0.12319439204805));
#39341=CARTESIAN_POINT('Ctrl Pts',(-0.0105233259587662,0.153906031279718,
-0.120568513381589));
#39342=CARTESIAN_POINT('Ctrl Pts',(-0.0635105999243186,0.140585228058283,
-0.117942634715127));
#39343=CARTESIAN_POINT('Ctrl Pts',(-0.0989745039313167,0.108121574286461,
-0.115316756048666));
#39344=CARTESIAN_POINT('Ctrl Pts',(-0.128692321342145,0.0809178875437671,
-0.113116338893874));
#39345=CARTESIAN_POINT('Ctrl Pts',(-0.146105230934553,0.0402720939482578,
-0.110915921739083));
#39346=CARTESIAN_POINT('Ctrl Pts',(-0.146449480434,-0.000112796118272305,
-0.108715504584291));
#39347=CARTESIAN_POINT('Origin',(0.,0.,-0.387));
#39348=CARTESIAN_POINT('',(-0.146419470807316,0.000121292426834327,-0.0515844954157089));
#39349=CARTESIAN_POINT('',(-0.146417921947427,0.000120753153388515,-0.0587155045842908));
#39350=CARTESIAN_POINT('',(-0.14635,-1.79227059055215E-17,-0.387));
#39351=CARTESIAN_POINT('Ctrl Pts',(-0.146419470807316,0.000121292426834327,
-0.0515844954157089));
#39352=CARTESIAN_POINT('Ctrl Pts',(-0.146499213746489,0.00902035961397621,
-0.0520690569427793));
#39353=CARTESIAN_POINT('Ctrl Pts',(-0.145757375492163,0.017906185955658,
-0.0525536184698496));
#39354=CARTESIAN_POINT('Ctrl Pts',(-0.144146186685956,0.0266311864910578,
-0.0530381799969199));
#39355=CARTESIAN_POINT('Ctrl Pts',(-0.135415022370369,0.0739126801525337,
-0.0556640586633812));
#39356=CARTESIAN_POINT('Ctrl Pts',(-0.101154118446619,0.116471290797761,
-0.0582899373298425));
#39357=CARTESIAN_POINT('Ctrl Pts',(-0.0568351738065945,0.135112443908202,
-0.0609158159963038));
#39358=CARTESIAN_POINT('Ctrl Pts',(-0.0125162291665695,0.153753597018643,
-0.0635416946627651));
#39359=CARTESIAN_POINT('Ctrl Pts',(0.0418607561897289,0.148477292594297,
-0.0661675733292264));
#39360=CARTESIAN_POINT('Ctrl Pts',(0.0817639052896394,0.121659133496513,
-0.0687934519956878));
#39361=CARTESIAN_POINT('Ctrl Pts',(0.121667054389549,0.0948409743987301,
-0.0714193306621491));
#39362=CARTESIAN_POINT('Ctrl Pts',(0.147096367233071,0.0464809606275097,
-0.0740452093286105));
#39363=CARTESIAN_POINT('Ctrl Pts',(0.146573626794785,-0.00159543872172704,
-0.0766710879950718));
#39364=CARTESIAN_POINT('Ctrl Pts',(0.146050886356499,-0.0496718380709638,
-0.0792969666615331));
#39365=CARTESIAN_POINT('Ctrl Pts',(0.119576092636403,-0.0974646229982186,
-0.0819228453279944));
#39366=CARTESIAN_POINT('Ctrl Pts',(0.0790977545786269,-0.123408586620134,
-0.0845487239944557));
#39367=CARTESIAN_POINT('Ctrl Pts',(0.0386194165208501,-0.14935255024205,
-0.0871746026609171));
#39368=CARTESIAN_POINT('Ctrl Pts',(-0.0158624658746058,-0.153447692558627,
-0.0898004813273783));
#39369=CARTESIAN_POINT('Ctrl Pts',(-0.0597635898992248,-0.13384528397374,
-0.0924263599938397));
#39370=CARTESIAN_POINT('Ctrl Pts',(-0.103664713923843,-0.114242875388853,
-0.095052238660301));
#39371=CARTESIAN_POINT('Ctrl Pts',(-0.136985079577624,-0.0709429159024997,
-0.0976781173267624));
#39372=CARTESIAN_POINT('Ctrl Pts',(-0.144688279001984,-0.0234850990679547,
-0.100303995993224));
#39373=CARTESIAN_POINT('Ctrl Pts',(-0.145940423987479,-0.0157708930480517,
-0.100730829134052));
#39374=CARTESIAN_POINT('Ctrl Pts',(-0.146515710232966,-0.00794682780091699,
-0.101157662274881));
#39375=CARTESIAN_POINT('Ctrl Pts',(-0.146448857461917,-0.000112937673885413,
-0.101584495415709));
#39376=CARTESIAN_POINT('Ctrl Pts',(-0.146449480434,-0.000112796118272305,
-0.108715504584291));
#39377=CARTESIAN_POINT('Ctrl Pts',(-0.146516042772921,-0.00792141383373452,
-0.108290043072621));
#39378=CARTESIAN_POINT('Ctrl Pts',(-0.145944473964313,-0.0157202773759087,
-0.107864581560952));
#39379=CARTESIAN_POINT('Ctrl Pts',(-0.144700337830555,-0.0234103305235109,
-0.107439120049282));
#39380=CARTESIAN_POINT('Ctrl Pts',(-0.137021733674351,-0.0708720772394546,
-0.104813241382821));
#39381=CARTESIAN_POINT('Ctrl Pts',(-0.103723991313499,-0.114189066349136,
-0.10218736271636));
#39382=CARTESIAN_POINT('Ctrl Pts',(-0.0598329080582324,-0.13381425959949,
-0.0995614840498983));
#39383=CARTESIAN_POINT('Ctrl Pts',(-0.0159418248029649,-0.153439452849846,
-0.096935605383437));
#39384=CARTESIAN_POINT('Ctrl Pts',(0.0385425993467187,-0.149372850240874,
-0.0943097267169755));
#39385=CARTESIAN_POINT('Ctrl Pts',(0.0790341514413548,-0.123449656692746,
-0.0916838480505142));
#39386=CARTESIAN_POINT('Ctrl Pts',(0.11952570353599,-0.0975264631446175,
-0.0890579693840529));
#39387=CARTESIAN_POINT('Ctrl Pts',(0.146024383575578,-0.0497466786573349,
-0.0864320907175918));
#39388=CARTESIAN_POINT('Ctrl Pts',(0.146572354104826,-0.00167087112836006,
-0.0838062120511305));
#39389=CARTESIAN_POINT('Ctrl Pts',(0.147120324634074,0.0464049364006154,
-0.0811803333846691));
#39390=CARTESIAN_POINT('Ctrl Pts',(0.121717585652978,0.0947767669712817,
-0.0785544547182077));
#39391=CARTESIAN_POINT('Ctrl Pts',(0.081827606874047,0.12161615159699,-0.0759285760517464));
#39392=CARTESIAN_POINT('Ctrl Pts',(0.0419376280951157,0.148455536222698,
-0.0733026973852851));
#39393=CARTESIAN_POINT('Ctrl Pts',(-0.0124395904816524,0.153762474903448,
-0.0706768187188237));
#39394=CARTESIAN_POINT('Ctrl Pts',(-0.056766830003724,0.135143108409308,
-0.0680509400523624));
#39395=CARTESIAN_POINT('Ctrl Pts',(-0.101094069525796,0.116523741915167,
-0.0654250613859011));
#39396=CARTESIAN_POINT('Ctrl Pts',(-0.135371329993171,0.0739780702461364,
-0.0627991827194396));
#39397=CARTESIAN_POINT('Ctrl Pts',(-0.144129485340515,0.0267032560390048,
-0.0601733040529783));
#39398=CARTESIAN_POINT('Ctrl Pts',(-0.14575022971269,0.017954794058933,
-0.0596873708967491));
#39399=CARTESIAN_POINT('Ctrl Pts',(-0.146497059078279,0.00904438013685962,
-0.05920143774052));
#39400=CARTESIAN_POINT('Ctrl Pts',(-0.146417921947427,0.000120753153388515,
-0.0587155045842908));
#39401=CARTESIAN_POINT('Origin',(0.,0.,-0.860086711473615));
#39402=CARTESIAN_POINT('',(-0.11783090655505,9.76099458120806E-5,-0.0350867114736151));
#39403=CARTESIAN_POINT('',(-0.117565879451543,-5.36239120088947E-5,-0.0252132885263834));
#39404=CARTESIAN_POINT('',(-0.117775,-1.1488940921122E-14,-0.860086711473615));
#39405=CARTESIAN_POINT('',(0.106341965058147,-0.0510185301167581,-0.01365));
#39406=CARTESIAN_POINT('Ctrl Pts',(-0.11783090655505,9.76099458120895E-5,
-0.0350867114736151));
#39407=CARTESIAN_POINT('Ctrl Pts',(-0.117547320619057,-0.0315497098533478,
-0.0329453943342242));
#39408=CARTESIAN_POINT('Ctrl Pts',(-0.0881713273287959,-0.102469121142594,
-0.0281781985283719));
#39409=CARTESIAN_POINT('Ctrl Pts',(0.0271354482247726,-0.134172264119296,
-0.0210326280371669));
#39410=CARTESIAN_POINT('Ctrl Pts',(0.090961439762511,-0.0825484450221484,
-0.0160283746853528));
#39411=CARTESIAN_POINT('Ctrl Pts',(0.106341965058147,-0.0510185301167582,
-0.01365));
#39412=CARTESIAN_POINT('',(-0.0138313775859342,-0.116960008631478,-0.0136500000000001));
#39413=CARTESIAN_POINT('Origin',(0.,0.,-0.0136499999999999));
#39414=CARTESIAN_POINT('Ctrl Pts',(-0.117565879451543,-5.36239120088964E-5,
-0.0252132885263835));
#39415=CARTESIAN_POINT('Ctrl Pts',(-0.117583343244632,-0.0183158611289637,
-0.0239847376840503));
#39416=CARTESIAN_POINT('Ctrl Pts',(-0.10502991826055,-0.075546691227487,
-0.0201303081752559));
#39417=CARTESIAN_POINT('Ctrl Pts',(-0.0524255658063026,-0.112395963227031,
-0.0162758786664614));
#39418=CARTESIAN_POINT('Ctrl Pts',(-0.0138313775859342,-0.116960008631478,
-0.0136500000000001));
#39419=CARTESIAN_POINT('Origin',(0.,0.,-0.860086711473615));
#39420=CARTESIAN_POINT('',(-0.117854555432711,-9.08864676626378E-5,-0.0850867114736154));
#39421=CARTESIAN_POINT('',(-0.117829660111775,9.71759660986608E-5,-0.0752132885263837));
#39422=CARTESIAN_POINT('',(-0.117775,-1.1488940921122E-14,-0.860086711473615));
#39423=CARTESIAN_POINT('Ctrl Pts',(-0.117854555432711,-9.08864676626335E-5,
-0.0850867114736154));
#39424=CARTESIAN_POINT('Ctrl Pts',(-0.117908355125983,-0.00639520084901597,
-0.084659878332787));
#39425=CARTESIAN_POINT('Ctrl Pts',(-0.114597257003647,-0.0514271270458079,
-0.0816071665254972));
#39426=CARTESIAN_POINT('Ctrl Pts',(-0.0566095361633514,-0.126782421437836,
-0.0759285760517461));
#39427=CARTESIAN_POINT('Ctrl Pts',(0.0749231669276979,-0.116895737741183,
-0.0680509400523622));
#39428=CARTESIAN_POINT('Ctrl Pts',(0.138839849477423,-0.00151216593098895,
-0.0601733040529782));
#39429=CARTESIAN_POINT('Ctrl Pts',(0.0774472156514042,0.115240836226281,
-0.0522956680535942));
#39430=CARTESIAN_POINT('Ctrl Pts',(-0.0538322401122725,0.127979136607092,
-0.0444180320542103));
#39431=CARTESIAN_POINT('Ctrl Pts',(-0.114062929272019,0.053161074172187,
-0.0386817131942172));
#39432=CARTESIAN_POINT('Ctrl Pts',(-0.117895079596807,0.0072591243835695,
-0.0355712730006855));
#39433=CARTESIAN_POINT('Ctrl Pts',(-0.11783090655505,9.76099458120895E-5,
-0.0350867114736151));
#39434=CARTESIAN_POINT('Ctrl Pts',(-0.117829660111775,9.71759660986617E-5,
-0.0752132885263837));
#39435=CARTESIAN_POINT('Ctrl Pts',(-0.117549202734137,-0.0315276377698398,
-0.0730733430161518));
#39436=CARTESIAN_POINT('Ctrl Pts',(-0.0882161036909192,-0.102417796622243,
-0.0683075188394586));
#39437=CARTESIAN_POINT('Ctrl Pts',(0.0310918033177442,-0.135313955894808,
-0.0609158159963039));
#39438=CARTESIAN_POINT('Ctrl Pts',(0.13019812432102,-0.0482707014283373,
-0.0530381799969201));
#39439=CARTESIAN_POINT('Ctrl Pts',(0.111769783231296,0.0823751383704014,
-0.045160543997536));
#39440=CARTESIAN_POINT('Ctrl Pts',(-0.00747498868383688,0.138604580907157,
-0.037282907998152));
#39441=CARTESIAN_POINT('Ctrl Pts',(-0.102520577346041,0.0805987077592062,
-0.0306338228411012));
#39442=CARTESIAN_POINT('Ctrl Pts',(-0.117546016501506,0.0207174596400722,
-0.0266106163505116));
#39443=CARTESIAN_POINT('Ctrl Pts',(-0.117565879451543,-5.36239120088964E-5,
-0.0252132885263835));
#39444=CARTESIAN_POINT('Origin',(0.,0.,-0.860086711473615));
#39445=CARTESIAN_POINT('',(-0.117588526013778,5.9658950325018E-6,-0.135086711473615));
#39446=CARTESIAN_POINT('',(-0.117855056768803,-9.0772550948498E-5,-0.125213288526384));
#39447=CARTESIAN_POINT('',(-0.117775,-1.1488940921122E-14,-0.860086711473615));
#39448=CARTESIAN_POINT('Ctrl Pts',(-0.117588526013778,5.96589503251525E-6,
-0.135086711473615));
#39449=CARTESIAN_POINT('Ctrl Pts',(-0.11757940935564,-0.0198736126399706,
-0.133748483664888));
#39450=CARTESIAN_POINT('Ctrl Pts',(-0.103412073402492,-0.0787732216373988,
-0.1297843771897));
#39451=CARTESIAN_POINT('Ctrl Pts',(-0.01059248606553,-0.138441959744445,
-0.12319439204805));
#39452=CARTESIAN_POINT('Ctrl Pts',(0.10992336877787,-0.0848246534005071,
-0.115316756048666));
#39453=CARTESIAN_POINT('Ctrl Pts',(0.131232546291422,0.045347541159856,
-0.107439120049282));
#39454=CARTESIAN_POINT('Ctrl Pts',(0.034103170842127,0.134593310063775,
-0.099561484049898));
#39455=CARTESIAN_POINT('Ctrl Pts',(-0.0868739814205058,0.104113427887564,
-0.0921106811913426));
#39456=CARTESIAN_POINT('Ctrl Pts',(-0.117577379263731,0.0323889587139717,
-0.0872857569992483));
#39457=CARTESIAN_POINT('Ctrl Pts',(-0.117854555432711,-9.08864676626335E-5,
-0.0850867114736154));
#39458=CARTESIAN_POINT('Ctrl Pts',(-0.117855056768803,-9.07725509484815E-5,
-0.125213288526384));
#39459=CARTESIAN_POINT('Ctrl Pts',(-0.117908622737142,-0.00637474898714989,
-0.124787827014714));
#39460=CARTESIAN_POINT('Ctrl Pts',(-0.114609797901413,-0.0513861008242438,
-0.121736486836584));
#39461=CARTESIAN_POINT('Ctrl Pts',(-0.0566754456467214,-0.126752823243337,
-0.116059267991992));
#39462=CARTESIAN_POINT('Ctrl Pts',(0.0748633938659991,-0.116935041440705,
-0.108181631992608));
#39463=CARTESIAN_POINT('Ctrl Pts',(0.138837743882996,-0.00158285589939853,
-0.100303995993224));
#39464=CARTESIAN_POINT('Ctrl Pts',(0.077509265915822,0.115198674926568,
-0.0924263599938399));
#39465=CARTESIAN_POINT('Ctrl Pts',(-0.0537707528995959,0.128010933958857,
-0.0845487239944558));
#39466=CARTESIAN_POINT('Ctrl Pts',(-0.11404460569689,0.0531977337096131,
-0.0788110335053037));
#39467=CARTESIAN_POINT('Ctrl Pts',(-0.117893345629958,0.00727845487268427,
-0.0756992216826131));
#39468=CARTESIAN_POINT('Ctrl Pts',(-0.117829660111775,9.71759660986617E-5,
-0.0752132885263837));
#39469=CARTESIAN_POINT('Origin',(0.,0.,-0.860086711473615));
#39470=CARTESIAN_POINT('',(-0.117874828748926,8.41669106047294E-5,-0.185086711473615));
#39471=CARTESIAN_POINT('',(-0.117588491764479,5.64203395312518E-6,-0.175213288526384));
#39472=CARTESIAN_POINT('',(-0.117775,-1.1488940921122E-14,-0.860086711473615));
#39473=CARTESIAN_POINT('Ctrl Pts',(-0.117874828748926,8.41669106047436E-5,
-0.185086711473615));
#39474=CARTESIAN_POINT('Ctrl Pts',(-0.117605527602309,-0.0331277613279678,
-0.18283708899699));
#39475=CARTESIAN_POINT('Ctrl Pts',(-0.085698280103056,-0.105559724356163,
-0.177961587853902));
#39476=CARTESIAN_POINT('Ctrl Pts',(0.0366631742567891,-0.133918582381201,
-0.170460208044354));
#39477=CARTESIAN_POINT('Ctrl Pts',(0.132073252696953,-0.042837259451921,
-0.16258257204497));
#39478=CARTESIAN_POINT('Ctrl Pts',(0.108286145990386,0.0869050379577989,
-0.154704936045586));
#39479=CARTESIAN_POINT('Ctrl Pts',(-0.0132300918964409,0.138214832825673,
-0.146827300046202));
#39480=CARTESIAN_POINT('Ctrl Pts',(-0.104191641877288,0.0772587042552975,
-0.140287891855545));
#39481=CARTESIAN_POINT('Ctrl Pts',(-0.117597298117148,0.0191342160965729,
-0.13637436233135));
#39482=CARTESIAN_POINT('Ctrl Pts',(-0.117588526013778,5.96589503251525E-6,
-0.135086711473615));
#39483=CARTESIAN_POINT('Ctrl Pts',(-0.117588491764479,5.64203395314773E-6,
-0.175213288526384));
#39484=CARTESIAN_POINT('Ctrl Pts',(-0.117579877620705,-0.019853573385154,
-0.173876432346816));
#39485=CARTESIAN_POINT('Ctrl Pts',(-0.103433474728503,-0.0787321665347216,
-0.169913697500786));
#39486=CARTESIAN_POINT('Ctrl Pts',(-0.0106640792440769,-0.138436453663531,
-0.163325083988296));
#39487=CARTESIAN_POINT('Ctrl Pts',(0.10987950347526,-0.0848814925592979,
-0.155447447988912));
#39488=CARTESIAN_POINT('Ctrl Pts',(0.13125594634982,0.04527969798971,-0.147569811989528));
#39489=CARTESIAN_POINT('Ctrl Pts',(0.0341728150085339,0.134575609384171,
-0.139692175990144));
#39490=CARTESIAN_POINT('Ctrl Pts',(-0.0868424965679614,0.104152811009239,
-0.132240001502429));
#39491=CARTESIAN_POINT('Ctrl Pts',(-0.117578022366365,0.0324089228886563,
-0.127413705681176));
#39492=CARTESIAN_POINT('Ctrl Pts',(-0.117855056768803,-9.07725509484815E-5,
-0.125213288526384));
#39493=CARTESIAN_POINT('Origin',(0.,0.,-0.860086711473615));
#39494=CARTESIAN_POINT('',(-0.117808253179095,-0.000100611602195776,-0.235086711473615));
#39495=CARTESIAN_POINT('',(-0.117874288948281,8.43690870912656E-5,-0.225213288526384));
#39496=CARTESIAN_POINT('',(-0.117775,-1.1488940921122E-14,-0.860086711473615));
#39497=CARTESIAN_POINT('Ctrl Pts',(-0.117808253179095,-0.000100611602195775,
-0.235086711473615));
#39498=CARTESIAN_POINT('Ctrl Pts',(-0.117879338460233,-0.00801262199676357,
-0.234551572995552));
#39499=CARTESIAN_POINT('Ctrl Pts',(-0.113566221109939,-0.0546711547288069,
-0.231390555851028));
#39500=CARTESIAN_POINT('Ctrl Pts',(-0.0513876737847133,-0.128987138809037,
-0.225603660040042));
#39501=CARTESIAN_POINT('Ctrl Pts',(0.0796330755882605,-0.113740706298137,
-0.217726024040658));
#39502=CARTESIAN_POINT('Ctrl Pts',(0.138784325562075,0.004157640156581,
-0.209848388041274));
#39503=CARTESIAN_POINT('Ctrl Pts',(0.0726815912474743,0.118303682479431,
-0.20197075204189));
#39504=CARTESIAN_POINT('Ctrl Pts',(-0.0590168712602702,0.125679687743678,
-0.194093116042506));
#39505=CARTESIAN_POINT('Ctrl Pts',(-0.11505331136728,0.0499137972881179,
-0.188465102519748));
#39506=CARTESIAN_POINT('Ctrl Pts',(-0.117919870183388,0.00563896275122834,
-0.185462967663451));
#39507=CARTESIAN_POINT('Ctrl Pts',(-0.117874828748926,8.41669106047436E-5,
-0.185086711473615));
#39508=CARTESIAN_POINT('Ctrl Pts',(-0.117874288948281,8.4369087091269E-5,
-0.225213288526384));
#39509=CARTESIAN_POINT('Ctrl Pts',(-0.11760470306281,-0.0331077028297975,
-0.222965037678917));
#39510=CARTESIAN_POINT('Ctrl Pts',(-0.0857304791730737,-0.105520590514,
-0.218090908164989));
#39511=CARTESIAN_POINT('Ctrl Pts',(0.0365939199639361,-0.133937518903554,
-0.210590899984599));
#39512=CARTESIAN_POINT('Ctrl Pts',(0.132051080927517,-0.0429055468321947,
-0.202713263985216));
#39513=CARTESIAN_POINT('Ctrl Pts',(0.108331065856659,0.0868490305592283,
-0.194835627985831));
#39514=CARTESIAN_POINT('Ctrl Pts',(-0.0131586188681242,0.138221650789034,
-0.186957991986448));
#39515=CARTESIAN_POINT('Ctrl Pts',(-0.104170762439501,0.0772997942322291,
-0.180417212166632));
#39516=CARTESIAN_POINT('Ctrl Pts',(-0.117596797687883,0.0191542801885525,
-0.176502311013277));
#39517=CARTESIAN_POINT('Ctrl Pts',(-0.117588491764479,5.64203395314773E-6,
-0.175213288526384));
#39518=CARTESIAN_POINT('Origin',(0.,0.,-0.860086711473615));
#39519=CARTESIAN_POINT('',(-0.117596201538205,3.10584990424738E-5,-0.285086711473616));
#39520=CARTESIAN_POINT('',(-0.117808848495488,-0.000100531858621397,-0.275213288526384));
#39521=CARTESIAN_POINT('',(-0.117775,-1.1488940921122E-14,-0.860086711473615));
#39522=CARTESIAN_POINT('Ctrl Pts',(-0.117596201538205,3.10584990424884E-5,
-0.285086711473616));
#39523=CARTESIAN_POINT('Ctrl Pts',(-0.117544694036852,-0.0214539032491567,
-0.283640178327653));
#39524=CARTESIAN_POINT('Ctrl Pts',(-0.10167468688571,-0.082011168264245,
-0.27956776651523));
#39525=CARTESIAN_POINT('Ctrl Pts',(-0.00493263138706642,-0.138758942569485,
-0.272869476036346));
#39526=CARTESIAN_POINT('Ctrl Pts',(0.113294213096355,-0.0802670310546098,
-0.264991840036961));
#39527=CARTESIAN_POINT('Ctrl Pts',(0.129272107399731,0.0506665298182005,
-0.257114204037578));
#39528=CARTESIAN_POINT('Ctrl Pts',(0.0285808717640413,0.1358731348154,-0.249236568038194));
#39529=CARTESIAN_POINT('Ctrl Pts',(-0.0893124882611786,0.100995120524423,
-0.241894070516873));
#39530=CARTESIAN_POINT('Ctrl Pts',(-0.117530529075574,0.0308109351862458,
-0.237177451662014));
#39531=CARTESIAN_POINT('Ctrl Pts',(-0.117808253179095,-0.000100611602195775,
-0.235086711473615));
#39532=CARTESIAN_POINT('Ctrl Pts',(-0.117808848495488,-0.000100531858621394,
-0.275213288526384));
#39533=CARTESIAN_POINT('Ctrl Pts',(-0.11787973499181,-0.00799215919477956,
-0.274679521677479));
#39534=CARTESIAN_POINT('Ctrl Pts',(-0.113579744177213,-0.0546300439782162,
-0.271519876162114));
#39535=CARTESIAN_POINT('Ctrl Pts',(-0.0514543637190464,-0.128960545878442,
-0.265734351980287));
#39536=CARTESIAN_POINT('Ctrl Pts',(0.0795742483504507,-0.113781865596983,
-0.257856715980903));
#39537=CARTESIAN_POINT('Ctrl Pts',(0.138786453094293,0.00408587522045665,
-0.249979079981519));
#39538=CARTESIAN_POINT('Ctrl Pts',(0.0727427534113967,0.118266080365061,
-0.242101443982136));
#39539=CARTESIAN_POINT('Ctrl Pts',(-0.0589518737717736,0.125710184628324,
-0.234223807982751));
#39540=CARTESIAN_POINT('Ctrl Pts',(-0.115041149280448,0.0499548242228102,
-0.228594422830834));
#39541=CARTESIAN_POINT('Ctrl Pts',(-0.117919569985349,0.00565948084119541,
-0.225590916345378));
#39542=CARTESIAN_POINT('Ctrl Pts',(-0.117874288948281,8.4369087091269E-5,
-0.225213288526384));
#39543=CARTESIAN_POINT('Origin',(0.,0.,-0.860086711473615));
#39544=CARTESIAN_POINT('',(-0.117913678466366,6.52086126365611E-5,-0.335086711473616));
#39545=CARTESIAN_POINT('',(-0.117596036550741,3.07491073512287E-5,-0.325213288526384));
#39546=CARTESIAN_POINT('',(-0.117775,-1.1488940921122E-14,-0.860086711473615));
#39547=CARTESIAN_POINT('Ctrl Pts',(-0.117913678466366,6.52086126365584E-5,
-0.335086711473616));
#39548=CARTESIAN_POINT('Ctrl Pts',(-0.117680645599752,-0.0347155948899763,
-0.332728783659755));
#39549=CARTESIAN_POINT('Ctrl Pts',(-0.0830999363091226,-0.10863285629369,
-0.327744977179433));
#39550=CARTESIAN_POINT('Ctrl Pts',(0.0420990144004436,-0.132310422801546,
-0.320135292032649));
#39551=CARTESIAN_POINT('Ctrl Pts',(0.133711744422676,-0.0374104851459921,
-0.312257656033266));
#39552=CARTESIAN_POINT('Ctrl Pts',(0.104648535928131,0.0912527200882886,
-0.304380020033881));
#39553=CARTESIAN_POINT('Ctrl Pts',(-0.0188608286767674,0.137559602125903,
-0.296502384034497));
#39554=CARTESIAN_POINT('Ctrl Pts',(-0.105794378680474,0.0740115415589361,
-0.290071281181076));
#39555=CARTESIAN_POINT('Ctrl Pts',(-0.11763819514282,0.0175475554189854,
-0.286266056994115));
#39556=CARTESIAN_POINT('Ctrl Pts',(-0.117596201538205,3.10584990424884E-5,
-0.285086711473616));
#39557=CARTESIAN_POINT('Ctrl Pts',(-0.117596036550741,3.07491073512287E-5,
-0.325213288526384));
#39558=CARTESIAN_POINT('Ctrl Pts',(-0.117545094609287,-0.0214339135322908,
-0.323768127009581));
#39559=CARTESIAN_POINT('Ctrl Pts',(-0.101697273673151,-0.0819702105434217,
-0.319697086826317));
#39560=CARTESIAN_POINT('Ctrl Pts',(-0.00500438172789432,-0.138756369592802,
-0.31300016797659));
#39561=CARTESIAN_POINT('Ctrl Pts',(0.113252689408266,-0.0803256016526085,
-0.305122531977208));
#39562=CARTESIAN_POINT('Ctrl Pts',(0.12929828583138,0.0505996760870913,
-0.297244895977823));
#39563=CARTESIAN_POINT('Ctrl Pts',(0.0286511260671305,0.135858333988494,
-0.289367259978439));
#39564=CARTESIAN_POINT('Ctrl Pts',(-0.0892822767652217,0.101034782961183,
-0.28202339082796));
#39565=CARTESIAN_POINT('Ctrl Pts',(-0.117531007192745,0.0308308885614153,
-0.277305400343941));
#39566=CARTESIAN_POINT('Ctrl Pts',(-0.117808848495488,-0.000100531858621394,
-0.275213288526384));
#39567=CARTESIAN_POINT('Origin',(0.,0.,-0.860086711473615));
#39568=CARTESIAN_POINT('',(-0.117760958805986,-0.000103413802380578,-0.385086711473616));
#39569=CARTESIAN_POINT('',(-0.117913234095501,6.54834407544293E-5,-0.375213288526384));
#39570=CARTESIAN_POINT('',(-0.117775,-1.1488940921122E-14,-0.860086711473615));
#39571=CARTESIAN_POINT('Ctrl Pts',(-0.117760958805986,-0.000103413802380574,
-0.385086711473616));
#39572=CARTESIAN_POINT('Ctrl Pts',(-0.11784536193606,-0.00962652777585667,
-0.384443267658318));
#39573=CARTESIAN_POINT('Ctrl Pts',(-0.112459473549584,-0.0579190182986298,
-0.381173945176558));
#39574=CARTESIAN_POINT('Ctrl Pts',(-0.0460797444479301,-0.130977219954565,
-0.375278744028337));
#39575=CARTESIAN_POINT('Ctrl Pts',(0.0842094664898252,-0.110395383730082,
-0.367401108028953));
#39576=CARTESIAN_POINT('Ctrl Pts',(0.138498947975746,0.0098191855581053,
-0.359523472029569));
#39577=CARTESIAN_POINT('Ctrl Pts',(0.0677920007431425,0.121171859895995,
-0.351645836030185));
#39578=CARTESIAN_POINT('Ctrl Pts',(-0.0640977793732191,0.123165943648539,
-0.343768200030801));
#39579=CARTESIAN_POINT('Ctrl Pts',(-0.115976893950903,0.0466766976138206,
-0.338248491845278));
#39580=CARTESIAN_POINT('Ctrl Pts',(-0.117940159919669,0.00401763917385966,
-0.335354662326216));
#39581=CARTESIAN_POINT('Ctrl Pts',(-0.117913678466366,6.52086126365584E-5,
-0.335086711473616));
#39582=CARTESIAN_POINT('Ctrl Pts',(-0.117913234095501,6.54834407544259E-5,
-0.375213288526384));
#39583=CARTESIAN_POINT('Ctrl Pts',(-0.117679560835611,-0.034695429594265,
-0.372856732341682));
#39584=CARTESIAN_POINT('Ctrl Pts',(-0.0831335314732004,-0.108594147982193,
-0.36787429749052));
#39585=CARTESIAN_POINT('Ctrl Pts',(0.042030590961085,-0.132332170550159,
-0.360265983972894));
#39586=CARTESIAN_POINT('Ctrl Pts',(0.133692378221512,-0.0374796203893622,
-0.352388347973512));
#39587=CARTESIAN_POINT('Ctrl Pts',(0.104695705119469,0.0911985924704521,
-0.344510711974126));
#39588=CARTESIAN_POINT('Ctrl Pts',(-0.0187896946723457,0.137569332749615,
-0.336633075974744));
#39589=CARTESIAN_POINT('Ctrl Pts',(-0.105774639104889,0.0740526910848505,
-0.330200601492162));
#39590=CARTESIAN_POINT('Ctrl Pts',(-0.117637656828621,0.0175676783679118,
-0.326394005676042));
#39591=CARTESIAN_POINT('Ctrl Pts',(-0.117596036550741,3.07491073512287E-5,
-0.325213288526384));
#39592=CARTESIAN_POINT('Origin',(0.,0.,-0.860086711473615));
#39593=CARTESIAN_POINT('',(-0.117614005739933,5.43156211771659E-5,-0.435086711473616));
#39594=CARTESIAN_POINT('',(-0.117761548966307,-0.000103421267928797,-0.425213288526384));
#39595=CARTESIAN_POINT('',(-0.117775,-1.1488940921122E-14,-0.860086711473615));
#39596=CARTESIAN_POINT('Ctrl Pts',(-0.117614005739933,5.43156211771697E-5,
-0.435086711473616));
#39597=CARTESIAN_POINT('Ctrl Pts',(-0.11751630423813,-0.023030516556304,
-0.433531872990419));
#39598=CARTESIAN_POINT('Ctrl Pts',(-0.0998427317906378,-0.085240110976336,
-0.429351155840761));
#39599=CARTESIAN_POINT('Ctrl Pts',(0.000735454065993374,-0.138844640165656,
-0.42254456002464));
#39600=CARTESIAN_POINT('Ctrl Pts',(0.116476194166392,-0.0755755991569081,
-0.414666924025258));
#39601=CARTESIAN_POINT('Ctrl Pts',(0.127096220251881,0.0559010357068483,
-0.406789288025873));
#39602=CARTESIAN_POINT('Ctrl Pts',(0.0230108722727937,0.136926530492298,
-0.39891165202649));
#39603=CARTESIAN_POINT('Ctrl Pts',(-0.0916440184411212,0.0978503402769418,
-0.391677459842403));
#39604=CARTESIAN_POINT('Ctrl Pts',(-0.117500914801167,0.0292370702985872,
-0.387069146324779));
#39605=CARTESIAN_POINT('Ctrl Pts',(-0.117760958805986,-0.000103413802380574,
-0.385086711473616));
#39606=CARTESIAN_POINT('Ctrl Pts',(-0.117761548966307,-0.000103421267928784,
-0.425213288526384));
#39607=CARTESIAN_POINT('Ctrl Pts',(-0.117845816925276,-0.00960611208181708,
-0.424571216340245));
#39608=CARTESIAN_POINT('Ctrl Pts',(-0.112473969195758,-0.0578778634222503,
-0.421303265487644));
#39609=CARTESIAN_POINT('Ctrl Pts',(-0.0461474642941204,-0.130953371389504,
-0.415409435968583));
#39610=CARTESIAN_POINT('Ctrl Pts',(0.0841523683577151,-0.110438909985756,
-0.407531799969199));
#39611=CARTESIAN_POINT('Ctrl Pts',(0.13850400308705,0.00974756728199353,
-0.399654163969815));
#39612=CARTESIAN_POINT('Ctrl Pts',(0.0678546468187308,0.121136785677018,
-0.391776527970431));
#39613=CARTESIAN_POINT('Ctrl Pts',(-0.0640340809268605,0.123199068255027,
-0.383898891971047));
#39614=CARTESIAN_POINT('Ctrl Pts',(-0.115965640736743,0.0467176601612722,
-0.378377812156364));
#39615=CARTESIAN_POINT('Ctrl Pts',(-0.117939939786918,0.00403818539778824,
-0.375482611008143));
#39616=CARTESIAN_POINT('Ctrl Pts',(-0.117913234095501,6.54834407544259E-5,
-0.375213288526384));
#39617=CARTESIAN_POINT('Origin',(0.,0.,-0.860086711473615));
#39618=CARTESIAN_POINT('',(-0.117943154879689,4.11508268803651E-5,-0.485086711473616));
#39619=CARTESIAN_POINT('',(-0.117613716614051,5.40385033010807E-5,-0.475213288526384));
#39620=CARTESIAN_POINT('',(-0.117775,-1.1488940921122E-14,-0.860086711473615));
#39621=CARTESIAN_POINT('Ctrl Pts',(-0.117943154879689,4.11508268803695E-5,
-0.485086711473616));
#39622=CARTESIAN_POINT('Ctrl Pts',(-0.117777131663363,-0.036313138524991,
-0.48262047832252));
#39623=CARTESIAN_POINT('Ctrl Pts',(-0.0803905871069344,-0.111670381593164,
-0.477528366504963));
#39624=CARTESIAN_POINT('Ctrl Pts',(0.0474646811631436,-0.130481719169871,
-0.469810376020945));
#39625=CARTESIAN_POINT('Ctrl Pts',(0.135127355757309,-0.0319213521242443,
-0.461932740021561));
#39626=CARTESIAN_POINT('Ctrl Pts',(0.10083649107415,0.0954482952349766,
-0.454055104022177));
#39627=CARTESIAN_POINT('Ctrl Pts',(-0.024460128186944,0.136675078651873,
-0.446177468022793));
#39628=CARTESIAN_POINT('Ctrl Pts',(-0.107308137190071,0.0707605300904387,
-0.439854670506606));
#39629=CARTESIAN_POINT('Ctrl Pts',(-0.117681306771859,0.0159561492541893,
-0.43615775165688));
#39630=CARTESIAN_POINT('Ctrl Pts',(-0.117614005739933,5.43156211771697E-5,
-0.435086711473616));
#39631=CARTESIAN_POINT('Ctrl Pts',(-0.117613716614051,5.40385033010841E-5,
-0.475213288526384));
#39632=CARTESIAN_POINT('Ctrl Pts',(-0.117516613707476,-0.0230105689760668,
-0.473659821672346));
#39633=CARTESIAN_POINT('Ctrl Pts',(-0.0998665302895594,-0.0851992819494425,
-0.469480476151846));
#39634=CARTESIAN_POINT('Ctrl Pts',(0.000663658498523691,-0.138844998096641,
-0.462675251964888));
#39635=CARTESIAN_POINT('Ctrl Pts',(0.11643709586757,-0.0756358158875735,
-0.454797615965502));
#39636=CARTESIAN_POINT('Ctrl Pts',(0.127125105754884,0.0558353062664104,
-0.446919979966119));
#39637=CARTESIAN_POINT('Ctrl Pts',(0.0230816721758652,0.136914609697508,
-0.439042343966735));
#39638=CARTESIAN_POINT('Ctrl Pts',(-0.0916151488647261,0.09789031515504,
-0.43180678015349));
#39639=CARTESIAN_POINT('Ctrl Pts',(-0.117501186772313,0.0292569840323692,
-0.427197095006706));
#39640=CARTESIAN_POINT('Ctrl Pts',(-0.117761548966307,-0.000103421267928784,
-0.425213288526384));
#39641=CARTESIAN_POINT('Origin',(0.,0.,-0.860086711473615));
#39642=CARTESIAN_POINT('',(-0.117715464068169,-9.94428558149901E-5,-0.535086711473616));
#39643=CARTESIAN_POINT('',(-0.117942852310966,4.1481206443531E-5,-0.525213288526384));
#39644=CARTESIAN_POINT('',(-0.117775,-1.1488940921122E-14,-0.860086711473615));
#39645=CARTESIAN_POINT('Ctrl Pts',(-0.117715464068169,-9.94428558149935E-5,
-0.535086711473616));
#39646=CARTESIAN_POINT('Ctrl Pts',(-0.117807243319497,-0.0112364652973298,
-0.534334962321083));
#39647=CARTESIAN_POINT('Ctrl Pts',(-0.111274845462934,-0.0611698966227711,
-0.530957334502088));
#39648=CARTESIAN_POINT('Ctrl Pts',(-0.0406950061935692,-0.13274897914597,
-0.524953828016632));
#39649=CARTESIAN_POINT('Ctrl Pts',(0.0886454911998817,-0.106866046463675,
-0.51707619201725));
#39650=CARTESIAN_POINT('Ctrl Pts',(0.137982710697811,0.0154643636671598,
-0.509198556017864));
#39651=CARTESIAN_POINT('Ctrl Pts',(0.0627894098300584,0.12383805961159,
-0.501320920018481));
#39652=CARTESIAN_POINT('Ctrl Pts',(-0.0690718448751183,0.120446898013915,
-0.493443284019097));
#39653=CARTESIAN_POINT('Ctrl Pts',(-0.116829683066834,0.0434448969256025,
-0.488031881170809));
#39654=CARTESIAN_POINT('Ctrl Pts',(-0.117953901982784,0.00239445601084412,
-0.485246356988981));
#39655=CARTESIAN_POINT('Ctrl Pts',(-0.117943154879689,4.11508268803695E-5,
-0.485086711473616));
#39656=CARTESIAN_POINT('Ctrl Pts',(-0.117942852310966,4.14812064435314E-5,
-0.525213288526384));
#39657=CARTESIAN_POINT('Ctrl Pts',(-0.117775766365834,-0.0362928338941266,
-0.522748427004448));
#39658=CARTESIAN_POINT('Ctrl Pts',(-0.0804255975098662,-0.111632149146056,
-0.517657686816049));
#39659=CARTESIAN_POINT('Ctrl Pts',(0.0473972024675744,-0.130506241756924,
-0.509941067961191));
#39660=CARTESIAN_POINT('Ctrl Pts',(0.135110827714643,-0.0319912202527791,
-0.502063431961806));
#39661=CARTESIAN_POINT('Ctrl Pts',(0.100885830377846,0.0953961381189002,
-0.494185795962423));
#39662=CARTESIAN_POINT('Ctrl Pts',(-0.0243894506605435,0.136687704770994,
-0.486308159963038));
#39663=CARTESIAN_POINT('Ctrl Pts',(-0.107289510134903,0.070801717063382,
-0.479983990817693));
#39664=CARTESIAN_POINT('Ctrl Pts',(-0.11768075010354,0.0159763334949808,
-0.476285700338808));
#39665=CARTESIAN_POINT('Ctrl Pts',(-0.117613716614051,5.40385033010841E-5,
-0.475213288526384));
#39666=CARTESIAN_POINT('Origin',(0.,0.,-0.860086711473615));
#39667=CARTESIAN_POINT('',(-0.117641121075241,7.43322482763471E-5,-0.585086711473616));
#39668=CARTESIAN_POINT('',(-0.117716014989814,-9.95338970442156E-5,-0.575213288526384));
#39669=CARTESIAN_POINT('',(-0.117775,-1.1488940921122E-14,-0.860086711473615));
#39670=CARTESIAN_POINT('Ctrl Pts',(-0.117641121075241,7.43322482763594E-5,
-0.585086711473616));
#39671=CARTESIAN_POINT('Ctrl Pts',(-0.11749601672539,-0.0246042219688241,
-0.583423567653184));
#39672=CARTESIAN_POINT('Ctrl Pts',(-0.0979139840066323,-0.0884576215721144,
-0.579134545166291));
#39673=CARTESIAN_POINT('Ctrl Pts',(0.00640231340113165,-0.138698901431908,
-0.572219644012936));
#39674=CARTESIAN_POINT('Ctrl Pts',(0.119464024723476,-0.0707581928149885,
-0.564342008013553));
#39675=CARTESIAN_POINT('Ctrl Pts',(0.124708480222252,0.0610423619770983,
-0.556464372014168));
#39676=CARTESIAN_POINT('Ctrl Pts',(0.0174025166897942,0.137751687439221,
-0.548586736014785));
#39677=CARTESIAN_POINT('Ctrl Pts',(-0.0938705497883859,0.0946825900337148,
-0.541460849167934));
#39678=CARTESIAN_POINT('Ctrl Pts',(-0.117486656090001,0.0276654337451075,
-0.536960840987544));
#39679=CARTESIAN_POINT('Ctrl Pts',(-0.117715464068169,-9.94428558149935E-5,
-0.535086711473616));
#39680=CARTESIAN_POINT('Ctrl Pts',(-0.117716014989814,-9.95338970442277E-5,
-0.575213288526384));
#39681=CARTESIAN_POINT('Ctrl Pts',(-0.117807744610619,-0.0112161026403652,
-0.574462911003011));
#39682=CARTESIAN_POINT('Ctrl Pts',(-0.111290340970323,-0.061128709613193,
-0.571086654813175));
#39683=CARTESIAN_POINT('Ctrl Pts',(-0.0407636430850622,-0.132727914643187,
-0.565084519956878));
#39684=CARTESIAN_POINT('Ctrl Pts',(0.0885902173532643,-0.10691186715079,
-0.557206883957495));
#39685=CARTESIAN_POINT('Ctrl Pts',(0.137990684964291,0.0153930114396808,
-0.54932924795811));
#39686=CARTESIAN_POINT('Ctrl Pts',(0.0628534353842331,0.123805571754376,
-0.541451611958728));
#39687=CARTESIAN_POINT('Ctrl Pts',(-0.0690095516253471,0.120482595112153,
-0.533573975959342));
#39688=CARTESIAN_POINT('Ctrl Pts',(-0.116819314516747,0.043485790171169,
-0.528161201481895));
#39689=CARTESIAN_POINT('Ctrl Pts',(-0.117953767204779,0.00241502130745575,
-0.525374305670909));
#39690=CARTESIAN_POINT('Ctrl Pts',(-0.117942852310966,4.14812064435314E-5,
-0.525213288526384));
#39691=CARTESIAN_POINT('Origin',(0.,0.,-0.860086711473615));
#39692=CARTESIAN_POINT('',(-0.117959517728684,1.36525406724091E-5,-0.635086711473616));
#39693=CARTESIAN_POINT('',(-0.117640721763206,7.41070646922068E-5,-0.625213288526384));
#39694=CARTESIAN_POINT('',(-0.117775,-1.1488940921122E-14,-0.860086711473615));
#39695=CARTESIAN_POINT('Ctrl Pts',(-0.117959517728684,1.36525406724122E-5,
-0.635086711473616));
#39696=CARTESIAN_POINT('Ctrl Pts',(-0.11789655159411,-0.0379230490610994,
-0.632512172985285));
#39697=CARTESIAN_POINT('Ctrl Pts',(-0.0775687689381847,-0.11466827637256,
-0.627311755830493));
#39698=CARTESIAN_POINT('Ctrl Pts',(0.0527512205227371,-0.128435499614995,
-0.619485460009241));
#39699=CARTESIAN_POINT('Ctrl Pts',(0.136317732660755,-0.0263790208529794,
-0.611607824009857));
#39700=CARTESIAN_POINT('Ctrl Pts',(0.0968563621793423,0.099484776038326,
-0.603730188010473));
#39701=CARTESIAN_POINT('Ctrl Pts',(-0.030018654400187,0.135562732744109,
-0.595852552011088));
#39702=CARTESIAN_POINT('Ctrl Pts',(-0.108735202118669,0.0675074251532259,
-0.589638059832136));
#39703=CARTESIAN_POINT('Ctrl Pts',(-0.117725116826057,0.0143598701569989,
-0.586049446319646));
#39704=CARTESIAN_POINT('Ctrl Pts',(-0.117641121075241,7.43322482763594E-5,
-0.585086711473616));
#39705=CARTESIAN_POINT('Ctrl Pts',(-0.117640721763206,7.41070646922016E-5,
-0.625213288526384));
#39706=CARTESIAN_POINT('Ctrl Pts',(-0.117496212726526,-0.0245843038632945,
-0.623551516335112));
#39707=CARTESIAN_POINT('Ctrl Pts',(-0.0979390209757794,-0.0884169574269978,
-0.619263865477377));
#39708=CARTESIAN_POINT('Ctrl Pts',(0.00633059155599267,-0.138702186982091,
-0.612350335953182));
#39709=CARTESIAN_POINT('Ctrl Pts',(0.119427417367179,-0.0708199567217074,
-0.604472699953798));
#39710=CARTESIAN_POINT('Ctrl Pts',(0.124740024447541,0.0609778671354031,
-0.596595063954414));
#39711=CARTESIAN_POINT('Ctrl Pts',(0.0174737442840939,0.137742666154633,
-0.588717427955029));
#39712=CARTESIAN_POINT('Ctrl Pts',(-0.0938429978234783,0.0947228355430488,
-0.581590169479021));
#39713=CARTESIAN_POINT('Ctrl Pts',(-0.117486745051261,0.0276853300359315,
-0.577088789669472));
#39714=CARTESIAN_POINT('Ctrl Pts',(-0.117716014989814,-9.95338970442277E-5,
-0.575213288526384));
#39715=CARTESIAN_POINT('Origin',(0.,0.,-0.860086711473615));
#39716=CARTESIAN_POINT('',(-0.117674062045845,-8.95928838821694E-5,-0.685086711473616));
#39717=CARTESIAN_POINT('',(-0.117959439303798,1.41398256485216E-5,-0.675213288526384));
#39718=CARTESIAN_POINT('',(-0.117775,-1.1488940921122E-14,-0.860086711473615));
#39719=CARTESIAN_POINT('Ctrl Pts',(-0.117674062045845,-8.959288388217E-5,
-0.685086711473616));
#39720=CARTESIAN_POINT('Ctrl Pts',(-0.117766071086712,-0.0128419083078311,
-0.684226656983848));
#39721=CARTESIAN_POINT('Ctrl Pts',(-0.110011270651638,-0.0644205347554902,
-0.680740723827619));
#39722=CARTESIAN_POINT('Ctrl Pts',(-0.0352415432127178,-0.134301243779432,
-0.674628912004927));
#39723=CARTESIAN_POINT('Ctrl Pts',(0.0929332862694289,-0.103157640277856,
-0.666751276005546));
#39724=CARTESIAN_POINT('Ctrl Pts',(0.137236721157382,0.0210832714786364,
-0.65887364000616));
#39725=CARTESIAN_POINT('Ctrl Pts',(0.0576820272073694,0.126298097011918,
-0.650996004006777));
#39726=CARTESIAN_POINT('Ctrl Pts',(-0.0739307082268856,0.11752694649454,
-0.643118368007392));
#39727=CARTESIAN_POINT('Ctrl Pts',(-0.117613549182942,0.0402187154116586,
-0.637815270496339));
#39728=CARTESIAN_POINT('Ctrl Pts',(-0.117960773368318,0.000770167553659683,
-0.635138051651747));
#39729=CARTESIAN_POINT('Ctrl Pts',(-0.117959517728684,1.36525406724122E-5,
-0.635086711473616));
#39730=CARTESIAN_POINT('Ctrl Pts',(-0.117959439303798,1.41398256485209E-5,
-0.675213288526384));
#39731=CARTESIAN_POINT('Ctrl Pts',(-0.117894944776542,-0.037902354392603,
-0.672640121667213));
#39732=CARTESIAN_POINT('Ctrl Pts',(-0.0776051478672742,-0.114630810377079,
-0.66744107614158));
#39733=CARTESIAN_POINT('Ctrl Pts',(0.052684764963274,-0.128462629580122,
-0.659616151949486));
#39734=CARTESIAN_POINT('Ctrl Pts',(0.136304088268209,-0.0264495720340304,
-0.651738515950102));
#39735=CARTESIAN_POINT('Ctrl Pts',(0.0969077799094599,0.0994347114333518,
-0.643860879950719));
#39736=CARTESIAN_POINT('Ctrl Pts',(-0.0299485461911899,0.135578214853137,
-0.635983243951333));
#39737=CARTESIAN_POINT('Ctrl Pts',(-0.108717659726821,0.0675486323374574,
-0.629767380143224));
#39738=CARTESIAN_POINT('Ctrl Pts',(-0.117724561232128,0.0143801195063431,
-0.626177395001573));
#39739=CARTESIAN_POINT('Ctrl Pts',(-0.117640721763206,7.41070646922016E-5,
-0.625213288526384));
#39740=CARTESIAN_POINT('Origin',(0.,0.,-0.860086711473615));
#39741=CARTESIAN_POINT('',(-0.11756447877375,-3.1000136807011E-5,-0.735086711473616));
#39742=CARTESIAN_POINT('',(-0.117673801045155,-9.24777646016256E-5,-0.725213288526384));
#39743=CARTESIAN_POINT('',(-0.117775,-1.1488940921122E-14,-0.860086711473615));
#39744=CARTESIAN_POINT('Ctrl Pts',(-0.11756447877375,-3.10001368070065E-5,
-0.735086711473616));
#39745=CARTESIAN_POINT('Ctrl Pts',(-0.117424235421919,-0.0262843339558975,
-0.733315262315949));
#39746=CARTESIAN_POINT('Ctrl Pts',(-0.0959617948024944,-0.0915157796904448,
-0.728917934491822));
#39747=CARTESIAN_POINT('Ctrl Pts',(0.0121016636501963,-0.138407426356883,
-0.721894728001232));
#39748=CARTESIAN_POINT('Ctrl Pts',(0.122230504106716,-0.0657785464558806,
-0.714017092001848));
#39749=CARTESIAN_POINT('Ctrl Pts',(0.122124503576362,0.0660587059756678,
-0.706139456002464));
#39750=CARTESIAN_POINT('Ctrl Pts',(0.0117590361697431,0.138359448122069,
-0.69826182000308));
#39751=CARTESIAN_POINT('Ctrl Pts',(-0.0959918518471737,0.0914906904383485,
-0.691244238493464));
#39752=CARTESIAN_POINT('Ctrl Pts',(-0.117485153330444,0.0260928724742271,
-0.68685253565031));
#39753=CARTESIAN_POINT('Ctrl Pts',(-0.117674062045845,-8.959288388217E-5,
-0.685086711473616));
#39754=CARTESIAN_POINT('Ctrl Pts',(-0.117673801045155,-9.24777646016256E-5,
-0.725213288526384));
#39755=CARTESIAN_POINT('Ctrl Pts',(-0.117766777010352,-0.0128209253377562,
-0.724354605665775));
#39756=CARTESIAN_POINT('Ctrl Pts',(-0.110031606923338,-0.0643651828756224,
-0.720870044138706));
#39757=CARTESIAN_POINT('Ctrl Pts',(-0.035307936335489,-0.134294310470789,
-0.714759603945173));
#39758=CARTESIAN_POINT('Ctrl Pts',(0.0928783259292375,-0.103199726094761,
-0.70688196794579));
#39759=CARTESIAN_POINT('Ctrl Pts',(0.137248444930391,0.0210091710227868,
-0.699004331946405));
#39760=CARTESIAN_POINT('Ctrl Pts',(0.0577468814636623,0.126269898836241,
-0.691126695947023));
#39761=CARTESIAN_POINT('Ctrl Pts',(-0.0738696902757825,0.117564288535968,
-0.683249059947637));
#39762=CARTESIAN_POINT('Ctrl Pts',(-0.117604048723001,0.040259560390861,
-0.677944590807425));
#39763=CARTESIAN_POINT('Ctrl Pts',(-0.117960760486325,0.000790866344265062,
-0.675266000333674));
#39764=CARTESIAN_POINT('Ctrl Pts',(-0.117959439303798,1.41398256485209E-5,
-0.675213288526384));
#39765=CARTESIAN_POINT('Origin',(3.28582941601228E-18,0.,-0.01365));
#39766=CARTESIAN_POINT('',(-0.00798678478682301,0.146131905375825,-0.0136500000000001));
#39767=CARTESIAN_POINT('Ctrl Pts',(0.106341965058147,-0.0510185301167581,
-0.01365));
#39768=CARTESIAN_POINT('Ctrl Pts',(0.108342566854854,-0.0479029045944487,
-0.01365));
#39769=CARTESIAN_POINT('Ctrl Pts',(0.110183088349928,-0.044695819810311,
-0.0136499999999998));
#39770=CARTESIAN_POINT('Ctrl Pts',(0.111853496790312,-0.0414060369465285,
-0.0136499999999998));
#39771=CARTESIAN_POINT('Ctrl Pts',(0.114271585472934,-0.0366437365899957,
-0.0136499999999998));
#39772=CARTESIAN_POINT('Ctrl Pts',(0.116333554267275,-0.0317083325327904,
-0.01365));
#39773=CARTESIAN_POINT('Ctrl Pts',(0.118049888741346,-0.026638969815401,
-0.01365));
#39774=CARTESIAN_POINT('Ctrl Pts',(0.11924838271765,-0.0230990999518747,
-0.01365));
#39775=CARTESIAN_POINT('Ctrl Pts',(0.120278297505165,-0.0194918553238869,
-0.0136499999999997));
#39776=CARTESIAN_POINT('Ctrl Pts',(0.121138443618246,-0.0158468448199564,
-0.0136499999999997));
#39777=CARTESIAN_POINT('Ctrl Pts',(0.122741275996562,-0.00905457921978598,
-0.0136499999999998));
#39778=CARTESIAN_POINT('Ctrl Pts',(0.123760167768593,-0.00212023278417033,
-0.0136499999999998));
#39779=CARTESIAN_POINT('Ctrl Pts',(0.124213451674144,0.00487494639068494,
-0.0136499999999998));
#39780=CARTESIAN_POINT('Ctrl Pts',(0.124483209002123,0.00903790214498723,
-0.0136499999999997));
#39781=CARTESIAN_POINT('Ctrl Pts',(0.124551731397662,0.0132256840072574,
-0.0136499999999997));
#39782=CARTESIAN_POINT('Ctrl Pts',(0.124422405850686,0.0173967602373136,
-0.0136499999999997));
#39783=CARTESIAN_POINT('Ctrl Pts',(0.124128401004826,0.0268791606815134,
-0.0136499999999999));
#39784=CARTESIAN_POINT('Ctrl Pts',(0.122818528710923,0.0362997013229908,
-0.0136500000000001));
#39785=CARTESIAN_POINT('Ctrl Pts',(0.120525658053403,0.045471105234349,
-0.0136500000000001));
#39786=CARTESIAN_POINT('Ctrl Pts',(0.119627364156967,0.0490642499799099,
-0.0136500000000002));
#39787=CARTESIAN_POINT('Ctrl Pts',(0.118577639382974,0.0526192976583267,
-0.0136499999999998));
#39788=CARTESIAN_POINT('Ctrl Pts',(0.117376297305641,0.0561250923148867,
-0.0136499999999998));
#39789=CARTESIAN_POINT('Ctrl Pts',(0.116377302902627,0.0590403895529535,
-0.0136499999999998));
#39790=CARTESIAN_POINT('Ctrl Pts',(0.115273111640123,0.0619215009930825,
-0.0136500000000001));
#39791=CARTESIAN_POINT('Ctrl Pts',(0.114069691815438,0.0647487244549216,
-0.0136500000000001));
#39792=CARTESIAN_POINT('Ctrl Pts',(0.111990795593586,0.0696327259085989,
-0.0136500000000001));
#39793=CARTESIAN_POINT('Ctrl Pts',(0.109612823724072,0.0743660871426123,
-0.0136499999999997));
#39794=CARTESIAN_POINT('Ctrl Pts',(0.106940366893081,0.0789174960988524,
-0.0136499999999998));
#39795=CARTESIAN_POINT('Ctrl Pts',(0.10367803111746,0.0844735163477981,
-0.0136499999999999));
#39796=CARTESIAN_POINT('Ctrl Pts',(0.0999772058860202,0.0897587318249706,
-0.01365));
#39797=CARTESIAN_POINT('Ctrl Pts',(0.0958886739670196,0.0947554852369029,
-0.01365));
#39798=CARTESIAN_POINT('Ctrl Pts',(0.0939519614645511,0.0971224166920954,
-0.01365));
#39799=CARTESIAN_POINT('Ctrl Pts',(0.0919280942758348,0.0994245574006695,
-0.0136499999999999));
#39800=CARTESIAN_POINT('Ctrl Pts',(0.0898217035368732,0.101659607670364,
-0.0136499999999999));
#39801=CARTESIAN_POINT('Ctrl Pts',(0.0875898148282813,0.104027821396241,
-0.0136499999999999));
#39802=CARTESIAN_POINT('Ctrl Pts',(0.0852708873134785,0.106314590966667,
-0.01365));
#39803=CARTESIAN_POINT('Ctrl Pts',(0.0828754001610831,0.108514666841639,
-0.01365));
#39804=CARTESIAN_POINT('Ctrl Pts',(0.0767368610952631,0.114152456087464,
-0.0136500000000001));
#39805=CARTESIAN_POINT('Ctrl Pts',(0.0700902785826064,0.119229332008775,
-0.0136500000000001));
#39806=CARTESIAN_POINT('Ctrl Pts',(0.0630385493739984,0.123708097010451,
-0.0136500000000001));
#39807=CARTESIAN_POINT('Ctrl Pts',(0.0583362796780647,0.126694649715408,
-0.0136500000000002));
#39808=CARTESIAN_POINT('Ctrl Pts',(0.0534533030596454,0.129415029588119,
-0.0136500000000001));
#39809=CARTESIAN_POINT('Ctrl Pts',(0.0484154076414554,0.13185404772708,
-0.0136500000000001));
#39810=CARTESIAN_POINT('Ctrl Pts',(0.0455727092826764,0.133230295601465,
-0.0136500000000002));
#39811=CARTESIAN_POINT('Ctrl Pts',(0.0426811633551951,0.134516309136496,
-0.0136500000000002));
#39812=CARTESIAN_POINT('Ctrl Pts',(0.0397579206933862,0.135704614292114,
-0.0136500000000002));
#39813=CARTESIAN_POINT('Ctrl Pts',(0.0301875705441006,0.139594984589468,
-0.0136500000000001));
#39814=CARTESIAN_POINT('Ctrl Pts',(0.0202471683700578,0.142457694671499,
-0.0136499999999998));
#39815=CARTESIAN_POINT('Ctrl Pts',(0.0101045343131722,0.144212130069045,
-0.0136499999999998));
#39816=CARTESIAN_POINT('Ctrl Pts',(0.00413458586419398,0.145244789713637,
-0.0136499999999998));
#39817=CARTESIAN_POINT('Ctrl Pts',(-0.00190612190526973,0.145892796544534,
-0.0136499999999999));
#39818=CARTESIAN_POINT('Ctrl Pts',(-0.00798678478682509,0.146131905375825,
-0.0136499999999999));
#39819=CARTESIAN_POINT('',(-0.14635,-1.79227059055215E-17,-0.01365));
#39820=CARTESIAN_POINT('Origin',(0.,0.,-0.01365));
#39821=CARTESIAN_POINT('',(-0.119316161853458,0.0851151957093249,-0.0136499999999998));
#39822=CARTESIAN_POINT('Origin',(0.,0.,-0.01365));
#39823=CARTESIAN_POINT('Ctrl Pts',(-0.119316161853456,0.0851151957093283,
-0.01365));
#39824=CARTESIAN_POINT('Ctrl Pts',(-0.121618076638167,0.0812021306583877,
-0.01365));
#39825=CARTESIAN_POINT('Ctrl Pts',(-0.123722085229027,0.0771843356216899,
-0.0136499999999999));
#39826=CARTESIAN_POINT('Ctrl Pts',(-0.1256140695707,0.0730688966137306,
-0.0136499999999999));
#39827=CARTESIAN_POINT('Ctrl Pts',(-0.128792092093133,0.0661560709793384,
-0.0136499999999999));
#39828=CARTESIAN_POINT('Ctrl Pts',(-0.131372690800445,0.0589676394657173,
-0.0136499999999999));
#39829=CARTESIAN_POINT('Ctrl Pts',(-0.133357756374321,0.0515830681614563,
-0.0136499999999998));
#39830=CARTESIAN_POINT('Ctrl Pts',(-0.134263694945998,0.0482129185463161,
-0.0136499999999998));
#39831=CARTESIAN_POINT('Ctrl Pts',(-0.13504450061239,0.0448044325552989,
-0.01365));
#39832=CARTESIAN_POINT('Ctrl Pts',(-0.135698940481304,0.0413736537756237,
-0.01365));
#39833=CARTESIAN_POINT('Ctrl Pts',(-0.136955087895919,0.0347885355716289,
-0.0136499999999998));
#39834=CARTESIAN_POINT('Ctrl Pts',(-0.137748728715298,0.0281123211991962,
-0.0136499999999999));
#39835=CARTESIAN_POINT('Ctrl Pts',(-0.138080117385458,0.0214001920011799,
-0.0136499999999999));
#39836=CARTESIAN_POINT('Ctrl Pts',(-0.138253918763604,0.017879922873254,
-0.0136499999999999));
#39837=CARTESIAN_POINT('Ctrl Pts',(-0.138300356470715,0.0143477408926489,
-0.0136500000000001));
#39838=CARTESIAN_POINT('Ctrl Pts',(-0.138218634317284,0.0108185068260204,
-0.0136500000000001));
#39839=CARTESIAN_POINT('Ctrl Pts',(-0.137988104065489,0.000862880550021112,
-0.0136500000000001));
#39840=CARTESIAN_POINT('Ctrl Pts',(-0.136743935784425,-0.00901554091696978,
-0.0136500000000002));
#39841=CARTESIAN_POINT('Ctrl Pts',(-0.134486996926361,-0.0186350354119432,
-0.0136500000000003));
#39842=CARTESIAN_POINT('Ctrl Pts',(-0.132955925535783,-0.0251607473338499,
-0.0136500000000003));
#39843=CARTESIAN_POINT('Ctrl Pts',(-0.130957707016009,-0.0315672393290349,
-0.0136500000000003));
#39844=CARTESIAN_POINT('Ctrl Pts',(-0.128480470731525,-0.0377902656536371,
-0.0136500000000003));
#39845=CARTESIAN_POINT('Ctrl Pts',(-0.127462904475702,-0.0403464778473128,
-0.0136500000000002));
#39846=CARTESIAN_POINT('Ctrl Pts',(-0.126364970507356,-0.0428696996823228,
-0.0136500000000001));
#39847=CARTESIAN_POINT('Ctrl Pts',(-0.125189987366655,-0.0453475440721538,
-0.0136500000000001));
#39848=CARTESIAN_POINT('Ctrl Pts',(-0.122981386926095,-0.0500051157610184,
-0.0136500000000001));
#39849=CARTESIAN_POINT('Ctrl Pts',(-0.120497522574337,-0.0545110076612892,
-0.0136500000000001));
#39850=CARTESIAN_POINT('Ctrl Pts',(-0.117735701698672,-0.0588371322340339,
-0.0136500000000001));
#39851=CARTESIAN_POINT('Ctrl Pts',(-0.114499346202997,-0.0639065692707884,
-0.0136500000000001));
#39852=CARTESIAN_POINT('Ctrl Pts',(-0.11088126561812,-0.0687293688896335,
-0.0136500000000003));
#39853=CARTESIAN_POINT('Ctrl Pts',(-0.106920330946986,-0.0732809440582911,
-0.0136500000000003));
#39854=CARTESIAN_POINT('Ctrl Pts',(-0.104866691559283,-0.0756408148510523,
-0.0136500000000003));
#39855=CARTESIAN_POINT('Ctrl Pts',(-0.102720811300817,-0.0779276639257738,
-0.01365));
#39856=CARTESIAN_POINT('Ctrl Pts',(-0.100487766234768,-0.0801372691093224,
-0.01365));
#39857=CARTESIAN_POINT('Ctrl Pts',(-0.0983185592222529,-0.0822837063361919,
-0.0136499999999999));
#39858=CARTESIAN_POINT('Ctrl Pts',(-0.096070846136074,-0.0843533002970022,
-0.01365));
#39859=CARTESIAN_POINT('Ctrl Pts',(-0.0937558409539707,-0.0863381453211609,
-0.01365));
#39860=CARTESIAN_POINT('Ctrl Pts',(-0.0882265183286274,-0.0910788900005786,
-0.01365));
#39861=CARTESIAN_POINT('Ctrl Pts',(-0.0823041470487266,-0.0953470446859006,
-0.0136500000000001));
#39862=CARTESIAN_POINT('Ctrl Pts',(-0.0760595239664612,-0.0990980605043351,
-0.01365));
#39863=CARTESIAN_POINT('Ctrl Pts',(-0.0711801715289065,-0.102028986508334,
-0.01365));
#39864=CARTESIAN_POINT('Ctrl Pts',(-0.0661037637394787,-0.104643891124205,
-0.01365));
#39865=CARTESIAN_POINT('Ctrl Pts',(-0.0608627395111615,-0.106913236962818,
-0.01365));
#39866=CARTESIAN_POINT('Ctrl Pts',(-0.0584349443975771,-0.107964464069964,
-0.01365));
#39867=CARTESIAN_POINT('Ctrl Pts',(-0.0559735570906737,-0.108940481663004,
-0.0136499999999999));
#39868=CARTESIAN_POINT('Ctrl Pts',(-0.0534903959610244,-0.109835670325941,
-0.0136499999999999));
#39869=CARTESIAN_POINT('Ctrl Pts',(-0.0452610837496131,-0.112802367455442,
-0.0136499999999998));
#39870=CARTESIAN_POINT('Ctrl Pts',(-0.0367667177655714,-0.114896564272088,
-0.0136500000000001));
#39871=CARTESIAN_POINT('Ctrl Pts',(-0.0281307376421152,-0.116018109833104,
-0.01365));
#39872=CARTESIAN_POINT('Ctrl Pts',(-0.0233995953608321,-0.116632538253301,
-0.01365));
#39873=CARTESIAN_POINT('Ctrl Pts',(-0.0186259220515163,-0.116954205068862,
-0.0136500000000001));
#39874=CARTESIAN_POINT('Ctrl Pts',(-0.0138313775859342,-0.116960008631478,
-0.0136500000000001));
#39875=CARTESIAN_POINT('Ctrl Pts',(0.103670563470625,-0.0558870726973871,
-0.754147783942094));
#39876=CARTESIAN_POINT('Ctrl Pts',(0.122112048111452,-0.0216781042960277,
-0.751521905275632));
#39877=CARTESIAN_POINT('Ctrl Pts',(0.122205985182819,0.0658325307641024,
-0.746270147942709));
#39878=CARTESIAN_POINT('Ctrl Pts',(0.0118087845259011,0.138432738517456,
-0.738392511943327));
#39879=CARTESIAN_POINT('Ctrl Pts',(-0.10914203235335,0.0857620083606503,
-0.730514875943941));
#39880=CARTESIAN_POINT('Ctrl Pts',(-0.13164238341053,-0.0441410325559887,
-0.722637239944559));
#39881=CARTESIAN_POINT('Ctrl Pts',(-0.035307936335489,-0.134294310470789,
-0.714759603945173));
#39882=CARTESIAN_POINT('Ctrl Pts',(0.0928783259292375,-0.103199726094761,
-0.70688196794579));
#39883=CARTESIAN_POINT('Ctrl Pts',(0.137248444930391,0.0210091710227868,
-0.699004331946405));
#39884=CARTESIAN_POINT('Ctrl Pts',(0.0577468814636623,0.126269898836241,
-0.691126695947023));
#39885=CARTESIAN_POINT('Ctrl Pts',(-0.0738696902757825,0.117564288535968,
-0.683249059947637));
#39886=CARTESIAN_POINT('Ctrl Pts',(-0.138819329421003,0.00275949030613511,
-0.675371423948254));
#39887=CARTESIAN_POINT('Ctrl Pts',(-0.0784828326356314,-0.114537633731478,
-0.66749378794887));
#39888=CARTESIAN_POINT('Ctrl Pts',(0.052684764963274,-0.128462629580122,
-0.659616151949486));
#39889=CARTESIAN_POINT('Ctrl Pts',(0.136304088268209,-0.0264495720340304,
-0.651738515950102));
#39890=CARTESIAN_POINT('Ctrl Pts',(0.0969077799094599,0.0994347114333518,
-0.643860879950719));
#39891=CARTESIAN_POINT('Ctrl Pts',(-0.0299485461911899,0.135578214853137,
-0.635983243951333));
#39892=CARTESIAN_POINT('Ctrl Pts',(-0.129776088039535,0.0493613502639795,
-0.628105607951951));
#39893=CARTESIAN_POINT('Ctrl Pts',(-0.112479641400627,-0.0814045746418012,
-0.620227971952565));
#39894=CARTESIAN_POINT('Ctrl Pts',(0.00633059155599267,-0.138702186982091,
-0.612350335953182));
#39895=CARTESIAN_POINT('Ctrl Pts',(0.119427417367179,-0.0708199567217074,
-0.604472699953798));
#39896=CARTESIAN_POINT('Ctrl Pts',(0.124740024447541,0.0609778671354031,
-0.596595063954414));
#39897=CARTESIAN_POINT('Ctrl Pts',(0.0174737442840939,0.137742666154633,
-0.588717427955029));
#39898=CARTESIAN_POINT('Ctrl Pts',(-0.105562732912909,0.0901935885599426,
-0.580839791955647));
#39899=CARTESIAN_POINT('Ctrl Pts',(-0.133327983520661,-0.0387559382421815,
-0.572962155956263));
#39900=CARTESIAN_POINT('Ctrl Pts',(-0.0407636430850622,-0.132727914643187,
-0.565084519956878));
#39901=CARTESIAN_POINT('Ctrl Pts',(0.0885902173532643,-0.10691186715079,
-0.557206883957495));
#39902=CARTESIAN_POINT('Ctrl Pts',(0.137990684964291,0.0153930114396808,
-0.54932924795811));
#39903=CARTESIAN_POINT('Ctrl Pts',(0.0628534353842331,0.123805571754376,
-0.541451611958728));
#39904=CARTESIAN_POINT('Ctrl Pts',(-0.0690095516253471,0.120482595112153,
-0.533573975959342));
#39905=CARTESIAN_POINT('Ctrl Pts',(-0.138590856156792,0.00842309494862901,
-0.525696339959959));
#39906=CARTESIAN_POINT('Ctrl Pts',(-0.0830927840904983,-0.11123831700858,
-0.517818703960574));
#39907=CARTESIAN_POINT('Ctrl Pts',(0.0473972024675744,-0.130506241756924,
-0.509941067961191));
#39908=CARTESIAN_POINT('Ctrl Pts',(0.135110827714643,-0.0319912202527791,
-0.502063431961806));
#39909=CARTESIAN_POINT('Ctrl Pts',(0.100885830377846,0.0953961381189002,
-0.494185795962423));
#39910=CARTESIAN_POINT('Ctrl Pts',(-0.0243894506605435,0.136687704770994,
-0.486308159963038));
#39911=CARTESIAN_POINT('Ctrl Pts',(-0.127653053808612,0.0546175044503093,
-0.478430523963655));
#39912=CARTESIAN_POINT('Ctrl Pts',(-0.115708736071418,-0.0767454385342013,
-0.470552887964269));
#39913=CARTESIAN_POINT('Ctrl Pts',(0.000663658498523691,-0.138844998096641,
-0.462675251964888));
#39914=CARTESIAN_POINT('Ctrl Pts',(0.11643709586757,-0.0756358158875735,
-0.454797615965502));
#39915=CARTESIAN_POINT('Ctrl Pts',(0.127125105754884,0.0558353062664104,
-0.446919979966119));
#39916=CARTESIAN_POINT('Ctrl Pts',(0.0230816721758652,0.136914609697508,
-0.439042343966735));
#39917=CARTESIAN_POINT('Ctrl Pts',(-0.101793158558169,0.094427362611722,
-0.431164707967351));
#39918=CARTESIAN_POINT('Ctrl Pts',(-0.134798834517268,-0.033281348407788,
-0.423287071967966));
#39919=CARTESIAN_POINT('Ctrl Pts',(-0.0461474642941204,-0.130953371389504,
-0.415409435968583));
#39920=CARTESIAN_POINT('Ctrl Pts',(0.0841523683577151,-0.110438909985756,
-0.407531799969199));
#39921=CARTESIAN_POINT('Ctrl Pts',(0.13850400308705,0.00974756728199353,
-0.399654163969815));
#39922=CARTESIAN_POINT('Ctrl Pts',(0.0678546468187308,0.121136785677018,
-0.391776527970431));
#39923=CARTESIAN_POINT('Ctrl Pts',(-0.0640340809268605,0.123199068255027,
-0.383898891971047));
#39924=CARTESIAN_POINT('Ctrl Pts',(-0.138131529033763,0.0140731881906393,
-0.376021255971662));
#39925=CARTESIAN_POINT('Ctrl Pts',(-0.0875641470101639,-0.107753858851722,
-0.368143619972279));
#39926=CARTESIAN_POINT('Ctrl Pts',(0.042030590961085,-0.132332170550159,
-0.360265983972894));
#39927=CARTESIAN_POINT('Ctrl Pts',(0.133692378221512,-0.0374796203893622,
-0.352388347973512));
#39928=CARTESIAN_POINT('Ctrl Pts',(0.104695705119469,0.0911985924704521,
-0.344510711974126));
#39929=CARTESIAN_POINT('Ctrl Pts',(-0.0187896946723457,0.137569332749615,
-0.336633075974744));
#39930=CARTESIAN_POINT('Ctrl Pts',(-0.125317241967218,0.0597826296242031,
-0.328755439975358));
#39931=CARTESIAN_POINT('Ctrl Pts',(-0.118744957590436,-0.0719583837082228,
-0.320877803975976));
#39932=CARTESIAN_POINT('Ctrl Pts',(-0.00500438172789432,-0.138756369592802,
-0.31300016797659));
#39933=CARTESIAN_POINT('Ctrl Pts',(0.113252689408266,-0.0803256016526085,
-0.305122531977208));
#39934=CARTESIAN_POINT('Ctrl Pts',(0.12929828583138,0.0505996760870913,
-0.297244895977823));
#39935=CARTESIAN_POINT('Ctrl Pts',(0.0286511260671305,0.135858333988494,
-0.289367259978439));
#39936=CARTESIAN_POINT('Ctrl Pts',(-0.0978539083562148,0.0985037388046721,
-0.281489623979056));
#39937=CARTESIAN_POINT('Ctrl Pts',(-0.136044993399579,-0.0277512830322524,
-0.273611987979671));
#39938=CARTESIAN_POINT('Ctrl Pts',(-0.0514543637190464,-0.128960545878442,
-0.265734351980287));
#39939=CARTESIAN_POINT('Ctrl Pts',(0.0795742483504507,-0.113781865596983,
-0.257856715980903));
#39940=CARTESIAN_POINT('Ctrl Pts',(0.138786453094293,0.00408587522045665,
-0.249979079981519));
#39941=CARTESIAN_POINT('Ctrl Pts',(0.0727427534113967,0.118266080365061,
-0.242101443982136));
#39942=CARTESIAN_POINT('Ctrl Pts',(-0.0589518737717736,0.125710184628324,
-0.234223807982751));
#39943=CARTESIAN_POINT('Ctrl Pts',(-0.137441954660273,0.0196998232527949,
-0.226346171983368));
#39944=CARTESIAN_POINT('Ctrl Pts',(-0.0918895519293831,-0.104089789049232,
-0.218468535983983));
#39945=CARTESIAN_POINT('Ctrl Pts',(0.0365939199639361,-0.133937518903554,
-0.210590899984599));
#39946=CARTESIAN_POINT('Ctrl Pts',(0.132051080927517,-0.0429055468321947,
-0.202713263985216));
#39947=CARTESIAN_POINT('Ctrl Pts',(0.108331065856659,0.0868490305592283,
-0.194835627985831));
#39948=CARTESIAN_POINT('Ctrl Pts',(-0.0131586188681242,0.138221650789034,
-0.186957991986448));
#39949=CARTESIAN_POINT('Ctrl Pts',(-0.122772542334386,0.0648481045786531,
-0.179080355987064));
#39950=CARTESIAN_POINT('Ctrl Pts',(-0.121583247309369,-0.0670513829332748,
-0.17120271998768));
#39951=CARTESIAN_POINT('Ctrl Pts',(-0.0106640792440769,-0.138436453663531,
-0.163325083988296));
#39952=CARTESIAN_POINT('Ctrl Pts',(0.10987950347526,-0.0848814925592979,
-0.155447447988912));
#39953=CARTESIAN_POINT('Ctrl Pts',(0.13125594634982,0.04527969798971,-0.147569811989528));
#39954=CARTESIAN_POINT('Ctrl Pts',(0.0341728150085339,0.134575609384171,
-0.139692175990144));
#39955=CARTESIAN_POINT('Ctrl Pts',(-0.0937515346592391,0.102415904579156,
-0.13181453999076));
#39956=CARTESIAN_POINT('Ctrl Pts',(-0.137064409224776,-0.0221749265765932,
-0.123936903991376));
#39957=CARTESIAN_POINT('Ctrl Pts',(-0.0566754456467214,-0.126752823243337,
-0.116059267991992));
#39958=CARTESIAN_POINT('Ctrl Pts',(0.0748633938659991,-0.116935041440705,
-0.108181631992608));
#39959=CARTESIAN_POINT('Ctrl Pts',(0.138837743882996,-0.00158285589939853,
-0.100303995993224));
#39960=CARTESIAN_POINT('Ctrl Pts',(0.077509265915822,0.115198674926568,
-0.0924263599938399));
#39961=CARTESIAN_POINT('Ctrl Pts',(-0.0537707528995959,0.128010933958857,
-0.0845487239944558));
#39962=CARTESIAN_POINT('Ctrl Pts',(-0.136524514803491,0.0252951878539005,
-0.0766710879950718));
#39963=CARTESIAN_POINT('Ctrl Pts',(-0.0960594476464373,-0.1002551914902,
-0.068793451995688));
#39964=CARTESIAN_POINT('Ctrl Pts',(0.0310918033177442,-0.135313955894808,
-0.0609158159963039));
#39965=CARTESIAN_POINT('Ctrl Pts',(0.13019812432102,-0.0482707014283373,
-0.0530381799969201));
#39966=CARTESIAN_POINT('Ctrl Pts',(0.111769783231296,0.0823751383704014,
-0.045160543997536));
#39967=CARTESIAN_POINT('Ctrl Pts',(-0.00747498868383688,0.138604580907157,
-0.037282907998152));
#39968=CARTESIAN_POINT('Ctrl Pts',(-0.120082141870022,0.0698809680050969,
-0.0294052719987681));
#39969=CARTESIAN_POINT('Ctrl Pts',(-0.12410032159439,-0.0621879015683824,
-0.0215276359993841));
#39970=CARTESIAN_POINT('Ctrl Pts',(-0.0524255658063026,-0.112395963227031,
-0.0162758786664614));
#39971=CARTESIAN_POINT('Ctrl Pts',(-0.0138313775859342,-0.116960008631478,
-0.0136500000000001));
#39972=CARTESIAN_POINT('Ctrl Pts',(0.112054873528428,-0.0604069144926977,
-0.748648522628062));
#39973=CARTESIAN_POINT('Ctrl Pts',(0.131987804921145,-0.0234313112025849,
-0.746022643961601));
#39974=CARTESIAN_POINT('Ctrl Pts',(0.132089339110787,0.0711567069944395,
-0.740770886628678));
#39975=CARTESIAN_POINT('Ctrl Pts',(0.0127638146478229,0.149628423801929,
-0.732893250629295));
#39976=CARTESIAN_POINT('Ctrl Pts',(-0.117968844989016,0.0926979721019815,
-0.72501561462991));
#39977=CARTESIAN_POINT('Ctrl Pts',(-0.142288901788669,-0.0477109186531712,
-0.717137978630527));
#39978=CARTESIAN_POINT('Ctrl Pts',(-0.0381634497602026,-0.145155302253716,
-0.709260342631142));
#39979=CARTESIAN_POINT('Ctrl Pts',(0.100389818643955,-0.111545957392173,
-0.701382706631759));
#39980=CARTESIAN_POINT('Ctrl Pts',(0.148348351005212,0.0227082782526056,
-0.693505070632373));
#39981=CARTESIAN_POINT('Ctrl Pts',(0.062417134454038,0.136481919947811,
-0.685627434632992));
#39982=CARTESIAN_POINT('Ctrl Pts',(-0.0798438681562896,0.127072247341361,
-0.677749798633605));
#39983=CARTESIAN_POINT('Ctrl Pts',(-0.15004628007042,0.00298266283991623,
-0.669872162634224));
#39984=CARTESIAN_POINT('Ctrl Pts',(-0.0848300963236339,-0.123800813194796,
-0.661994526634838));
#39985=CARTESIAN_POINT('Ctrl Pts',(0.0569456215650577,-0.138851986801525,
-0.654116890635456));
#39986=CARTESIAN_POINT('Ctrl Pts',(0.147327619923948,-0.0285886692416235,
-0.64623925463607));
#39987=CARTESIAN_POINT('Ctrl Pts',(0.104745152897256,0.107476448868313,
-0.638361618636687));
#39988=CARTESIAN_POINT('Ctrl Pts',(-0.032370621355452,0.146543041823854,
-0.630483982637303));
#39989=CARTESIAN_POINT('Ctrl Pts',(-0.140271670621378,0.0533534272010589,
-0.622606346637919));
#39990=CARTESIAN_POINT('Ctrl Pts',(-0.121576381662491,-0.0879881328966351,
-0.614728710638534));
#39991=CARTESIAN_POINT('Ctrl Pts',(0.0068425752925302,-0.149919663789601,
-0.606851074639151));
#39992=CARTESIAN_POINT('Ctrl Pts',(0.12908605587639,-0.0765474887766799,
-0.598973438639767));
#39993=CARTESIAN_POINT('Ctrl Pts',(0.134828317658009,0.0659094246345719,
-0.591095802640382));
#39994=CARTESIAN_POINT('Ctrl Pts',(0.0188869254711551,0.148882542148034,
-0.583218166641));
#39995=CARTESIAN_POINT('Ctrl Pts',(-0.114100071320851,0.0974879543509301,
-0.575340530641614));
#39996=CARTESIAN_POINT('Ctrl Pts',(-0.14411082404738,-0.0418903072657999,
-0.567462894642231));
#39997=CARTESIAN_POINT('Ctrl Pts',(-0.0440603843322313,-0.143462224870114,
-0.559585258642847));
#39998=CARTESIAN_POINT('Ctrl Pts',(0.0957549112211459,-0.115558316181665,
-0.551707622643463));
#39999=CARTESIAN_POINT('Ctrl Pts',(0.14915061936705,0.016637914296508,-0.543829986644079));
#40000=CARTESIAN_POINT('Ctrl Pts',(0.0679366786195117,0.133818291524789,
-0.535952350644695));
#40001=CARTESIAN_POINT('Ctrl Pts',(-0.0745906679847724,0.130226570645529,
-0.528074714645311));
#40002=CARTESIAN_POINT('Ctrl Pts',(-0.149799329134024,0.00910430895317851,
-0.520197078645927));
#40003=CARTESIAN_POINT('Ctrl Pts',(-0.0898128755229932,-0.120234665720163,
-0.512319442646543));
#40004=CARTESIAN_POINT('Ctrl Pts',(0.0512304298375893,-0.14106087519131,
-0.504441806647159));
#40005=CARTESIAN_POINT('Ctrl Pts',(0.146037854961359,-0.0345784957603811,
-0.496564170647776));
#40006=CARTESIAN_POINT('Ctrl Pts',(0.109044926402886,0.103111257758742,
-0.488686534648391));
#40007=CARTESIAN_POINT('Ctrl Pts',(-0.0263619364813165,0.147742261238358,
-0.480808898649007));
#40008=CARTESIAN_POINT('Ctrl Pts',(-0.13797693695467,0.0590346704863042,
-0.472931262649624));
#40009=CARTESIAN_POINT('Ctrl Pts',(-0.125066627908228,-0.0829521912579385,
-0.465053626650239));
#40010=CARTESIAN_POINT('Ctrl Pts',(0.000717331580232957,-0.150074024688621,
-0.457175990650856));
#40011=CARTESIAN_POINT('Ctrl Pts',(0.12585389347435,-0.0817528283802863,
-0.449298354651471));
#40012=CARTESIAN_POINT('Ctrl Pts',(0.13740629134024,0.0603509614749642,
-0.441420718652087));
#40013=CARTESIAN_POINT('Ctrl Pts',(0.0249483920015943,0.147987516998452,
-0.433543082652704));
#40014=CARTESIAN_POINT('Ctrl Pts',(-0.110025634340521,0.10206413296941,
-0.42566544665332));
#40015=CARTESIAN_POINT('Ctrl Pts',(-0.145700629454878,-0.0359729624479837,
-0.417787810653936));
#40016=CARTESIAN_POINT('Ctrl Pts',(-0.0498796196530811,-0.141544166231236,
-0.409910174654552));
#40017=CARTESIAN_POINT('Ctrl Pts',(0.0909581531898705,-0.119370607014959,
-0.402032538655167));
#40018=CARTESIAN_POINT('Ctrl Pts',(0.149705451861443,0.0105358973890694,
-0.394154902655784));
#40019=CARTESIAN_POINT('Ctrl Pts',(0.0733423607728681,0.130933668577239,
-0.386277266656399));
#40020=CARTESIAN_POINT('Ctrl Pts',(-0.0692128083378411,0.133162737328507,
-0.378399630657016));
#40021=CARTESIAN_POINT('Ctrl Pts',(-0.149302854137109,0.0152113509375375,
-0.370521994657631));
#40022=CARTESIAN_POINT('Ctrl Pts',(-0.0946458579018804,-0.11646840358161,
-0.362644358658248));
#40023=CARTESIAN_POINT('Ctrl Pts',(0.0454297960462407,-0.143034475152072,
-0.354766722658863));
#40024=CARTESIAN_POINT('Ctrl Pts',(0.144504689005293,-0.040510767782347,
-0.34688908665948));
#40025=CARTESIAN_POINT('Ctrl Pts',(0.11316292304571,0.0985742374993713,
-0.339011450660095));
#40026=CARTESIAN_POINT('Ctrl Pts',(-0.0203093027534662,0.148695190482071,
-0.331133814660713));
#40027=CARTESIAN_POINT('Ctrl Pts',(-0.135452217384223,0.0646175228287937,
-0.323256178661327));
#40028=CARTESIAN_POINT('Ctrl Pts',(-0.128348402473042,-0.0777779855322154,
-0.315378542661945));
#40029=CARTESIAN_POINT('Ctrl Pts',(-0.00540910884280258,-0.149978228394512,
-0.30750090666256));
#40030=CARTESIAN_POINT('Ctrl Pts',(0.122411949579047,-0.0868218984536377,
-0.299623270663176));
#40031=CARTESIAN_POINT('Ctrl Pts',(0.139755226375163,0.0546919020665389,
-0.291745634663792));
#40032=CARTESIAN_POINT('Ctrl Pts',(0.0309682729640912,0.146845815467929,
-0.283867998664408));
#40033=CARTESIAN_POINT('Ctrl Pts',(-0.105767799055369,0.106470184248226,
-0.275990362665024));
#40034=CARTESIAN_POINT('Ctrl Pts',(-0.147047570874689,-0.0299956555296591,
-0.26811272666564));
#40035=CARTESIAN_POINT('Ctrl Pts',(-0.0556157121752046,-0.139390171855875,
-0.260235090666256));
#40036=CARTESIAN_POINT('Ctrl Pts',(0.0860097797920805,-0.12298392265333,
-0.252357454666872));
#40037=CARTESIAN_POINT('Ctrl Pts',(0.150010744885616,0.00441631853588612,
-0.244479818667488));
#40038=CARTESIAN_POINT('Ctrl Pts',(0.0786257907813281,0.127830796268072,
-0.236602182668104));
#40039=CARTESIAN_POINT('Ctrl Pts',(-0.0637195799715275,0.135876939105801,
-0.22872454666872));
#40040=CARTESIAN_POINT('Ctrl Pts',(-0.148557510747211,0.0212930375723279,
-0.220846910669336));
#40041=CARTESIAN_POINT('Ctrl Pts',(-0.0993210779928724,-0.112508003786603,
-0.212969274669952));
#40042=CARTESIAN_POINT('Ctrl Pts',(0.0395534367345272,-0.14476965532942,
-0.205091638670569));
#40043=CARTESIAN_POINT('Ctrl Pts',(0.14273065253299,-0.0463755135787604,
-0.197214002671184));
#40044=CARTESIAN_POINT('Ctrl Pts',(0.11709229194271,0.0938729067305426,
-0.189336366671801));
#40045=CARTESIAN_POINT('Ctrl Pts',(-0.0142228162335986,0.149400264448687,
-0.181458730672416));
#40046=CARTESIAN_POINT('Ctrl Pts',(-0.132701716316428,0.070092665785291,
-0.173581094673032));
#40047=CARTESIAN_POINT('Ctrl Pts',(-0.131416237592721,-0.0724741332830037,
-0.165703458673648));
#40048=CARTESIAN_POINT('Ctrl Pts',(-0.0115265318426756,-0.149632439408767,
-0.157825822674264));
#40049=CARTESIAN_POINT('Ctrl Pts',(0.118765958755258,-0.0917462449823706,
-0.14994818667488));
#40050=CARTESIAN_POINT('Ctrl Pts',(0.141871211804985,0.0489416731402246,
-0.142070550675496));
#40051=CARTESIAN_POINT('Ctrl Pts',(0.0369365260079516,0.145459351089831,
-0.134192914676113));
#40052=CARTESIAN_POINT('Ctrl Pts',(-0.101333647736116,0.110698744665053,
-0.126315278676728));
#40053=CARTESIAN_POINT('Ctrl Pts',(-0.148149431494919,-0.0239683137609865,
-0.118437642677345));
#40054=CARTESIAN_POINT('Ctrl Pts',(-0.0612590467486968,-0.137003900648497,
-0.110560006677961));
#40055=CARTESIAN_POINT('Ctrl Pts',(0.0809179370761331,-0.126392110171104,
-0.102682370678577));
#40056=CARTESIAN_POINT('Ctrl Pts',(0.15006618379372,-0.00171086865628145,
-0.0948047346791928));
#40057=CARTESIAN_POINT('Ctrl Pts',(0.0837777928345086,0.124515315798361,
-0.0869270986798086));
#40058=CARTESIAN_POINT('Ctrl Pts',(-0.0581194382858709,0.138363760500637,
-0.0790494626804247));
#40059=CARTESIAN_POINT('Ctrl Pts',(-0.147565873355843,0.0273409247616357,
-0.0711718266810408));
#40060=CARTESIAN_POINT('Ctrl Pts',(-0.10382821214512,-0.108363284879664,
-0.0632941906816567));
#40061=CARTESIAN_POINT('Ctrl Pts',(0.033606338886425,-0.14625741104147,
-0.0554165546822729));
#40062=CARTESIAN_POINT('Ctrl Pts',(0.14072783889676,-0.0521745726327952,
-0.0475389186828887));
#40063=CARTESIAN_POINT('Ctrl Pts',(0.120809114033913,0.0890371905289917,
-0.0396612826835049));
#40064=CARTESIAN_POINT('Ctrl Pts',(-0.00807952502188328,0.149814163867383,
-0.0317836466841208));
#40065=CARTESIAN_POINT('Ctrl Pts',(-0.129793730928073,0.075532559771165,
-0.0239060106847369));
#40066=CARTESIAN_POINT('Ctrl Pts',(-0.134136879125162,-0.0672173200565058,
-0.0160283746853529));
#40067=CARTESIAN_POINT('Ctrl Pts',(-0.0566654597931856,-0.121485936054349,
-0.0107766173524302));
#40068=CARTESIAN_POINT('Ctrl Pts',(-0.014949984009251,-0.126419096572168,
-0.00815073868596886));
#40069=CARTESIAN_POINT('Ctrl Pts',(0.12043918358623,-0.0649267562880083,
-0.743149261314031));
#40070=CARTESIAN_POINT('Ctrl Pts',(0.141863561730838,-0.0251845181091421,
-0.74052338264757));
#40071=CARTESIAN_POINT('Ctrl Pts',(0.141972693038755,0.0764808832247766,
-0.735271625314647));
#40072=CARTESIAN_POINT('Ctrl Pts',(0.0137188447697446,0.160824109086401,
-0.727393989315264));
#40073=CARTESIAN_POINT('Ctrl Pts',(-0.126795657624682,0.0996339358433128,
-0.719516353315879));
#40074=CARTESIAN_POINT('Ctrl Pts',(-0.152935420166808,-0.0512808047503536,
-0.711638717316496));
#40075=CARTESIAN_POINT('Ctrl Pts',(-0.0410189631849163,-0.156016294036643,
-0.703761081317111));
#40076=CARTESIAN_POINT('Ctrl Pts',(0.107901311358673,-0.119892188689585,
-0.695883445317728));
#40077=CARTESIAN_POINT('Ctrl Pts',(0.159448257080032,0.0244073854824245,
-0.688005809318343));
#40078=CARTESIAN_POINT('Ctrl Pts',(0.0670873874444137,0.146693941059381,
-0.68012817331896));
#40079=CARTESIAN_POINT('Ctrl Pts',(-0.0858180460367966,0.136580206146754,
-0.672250537319575));
#40080=CARTESIAN_POINT('Ctrl Pts',(-0.161273230719836,0.00320583537369734,
-0.664372901320192));
#40081=CARTESIAN_POINT('Ctrl Pts',(-0.0911773600116365,-0.133063992658113,
-0.656495265320807));
#40082=CARTESIAN_POINT('Ctrl Pts',(0.0612064781668413,-0.149241344022927,
-0.648617629321424));
#40083=CARTESIAN_POINT('Ctrl Pts',(0.158351151579687,-0.0307277664492165,
-0.640739993322038));
#40084=CARTESIAN_POINT('Ctrl Pts',(0.112582525885052,0.115518186303275,
-0.632862357322657));
#40085=CARTESIAN_POINT('Ctrl Pts',(-0.0347926965197141,0.157507868794571,
-0.624984721323271));
#40086=CARTESIAN_POINT('Ctrl Pts',(-0.15076725320322,0.0573455041381383,
-0.617107085323888));
#40087=CARTESIAN_POINT('Ctrl Pts',(-0.130673121924355,-0.0945716911514688,
-0.609229449324504));
#40088=CARTESIAN_POINT('Ctrl Pts',(0.00735455902906769,-0.16113714059711,
-0.60135181332512));
#40089=CARTESIAN_POINT('Ctrl Pts',(0.138744694385601,-0.0822750208316521,
-0.593474177325735));
#40090=CARTESIAN_POINT('Ctrl Pts',(0.144916610868477,0.0708409821337405,
-0.585596541326352));
#40091=CARTESIAN_POINT('Ctrl Pts',(0.0203001066582162,0.160022418141436,
-0.577718905326968));
#40092=CARTESIAN_POINT('Ctrl Pts',(-0.122637409728793,0.104782320141917,
-0.569841269327584));
#40093=CARTESIAN_POINT('Ctrl Pts',(-0.154893664574099,-0.0450246762894181,
-0.5619636333282));
#40094=CARTESIAN_POINT('Ctrl Pts',(-0.0473571255794006,-0.154196535097041,
-0.554085997328815));
#40095=CARTESIAN_POINT('Ctrl Pts',(0.102919605089028,-0.12420476521254,
-0.546208361329432));
#40096=CARTESIAN_POINT('Ctrl Pts',(0.160310553769808,0.0178828171533352,
-0.538330725330049));
#40097=CARTESIAN_POINT('Ctrl Pts',(0.0730199218547905,0.143831011295202,
-0.530453089330663));
#40098=CARTESIAN_POINT('Ctrl Pts',(-0.0801717843441979,0.139970546178904,
-0.52257545333128));
#40099=CARTESIAN_POINT('Ctrl Pts',(-0.161007802111255,0.00978552295772822,
-0.514697817331896));
#40100=CARTESIAN_POINT('Ctrl Pts',(-0.0965329669554883,-0.129231014431746,
-0.506820181332512));
#40101=CARTESIAN_POINT('Ctrl Pts',(0.0550636572076045,-0.151615508625695,
-0.498942545333128));
#40102=CARTESIAN_POINT('Ctrl Pts',(0.156964882208075,-0.0371657712679834,
-0.491064909333744));
#40103=CARTESIAN_POINT('Ctrl Pts',(0.117204022427926,0.110826377398585,
-0.48318727333436));
#40104=CARTESIAN_POINT('Ctrl Pts',(-0.0283344223020895,0.158796817705721,
-0.475309637334976));
#40105=CARTESIAN_POINT('Ctrl Pts',(-0.148300820100728,0.0634518365222992,
-0.467432001335592));
#40106=CARTESIAN_POINT('Ctrl Pts',(-0.134424519745038,-0.0891589439816757,
-0.459554365336208));
#40107=CARTESIAN_POINT('Ctrl Pts',(0.000771004661942072,-0.161303051280602,
-0.451676729336824));
#40108=CARTESIAN_POINT('Ctrl Pts',(0.13527069108113,-0.087869840872999,
-0.44379909333744));
#40109=CARTESIAN_POINT('Ctrl Pts',(0.147687476925596,0.0648666166835182,
-0.435921457338057));
#40110=CARTESIAN_POINT('Ctrl Pts',(0.0268151118273235,0.159060424299397,
-0.428043821338672));
#40111=CARTESIAN_POINT('Ctrl Pts',(-0.118258110122872,0.109700903327099,
-0.420166185339288));
#40112=CARTESIAN_POINT('Ctrl Pts',(-0.156602424392488,-0.0386645764881796,
-0.412288549339904));
#40113=CARTESIAN_POINT('Ctrl Pts',(-0.0536117750120421,-0.152134961072968,
-0.404410913340521));
#40114=CARTESIAN_POINT('Ctrl Pts',(0.0977639380220263,-0.128302304044162,
-0.396533277341136));
#40115=CARTESIAN_POINT('Ctrl Pts',(0.160906900635836,0.0113242274961454,
-0.388655641341753));
#40116=CARTESIAN_POINT('Ctrl Pts',(0.0788300747270055,0.14073055147746,
-0.380778005342368));
#40117=CARTESIAN_POINT('Ctrl Pts',(-0.0743915357488216,0.143126406401988,
-0.372900369342985));
#40118=CARTESIAN_POINT('Ctrl Pts',(-0.160474179240455,0.0163495136844361,
-0.3650227333436));
#40119=CARTESIAN_POINT('Ctrl Pts',(-0.101727568793597,-0.125182948311499,
-0.357145097344217));
#40120=CARTESIAN_POINT('Ctrl Pts',(0.0488290011313963,-0.153736779753985,
-0.349267461344832));
#40121=CARTESIAN_POINT('Ctrl Pts',(0.155316999789075,-0.043541915175332,
-0.341389825345449));
#40122=CARTESIAN_POINT('Ctrl Pts',(0.121630140971951,0.105949882528291,
-0.333512189346064));
#40123=CARTESIAN_POINT('Ctrl Pts',(-0.0218289108345867,0.159821048214528,
-0.325634553346681));
#40124=CARTESIAN_POINT('Ctrl Pts',(-0.145587192801227,0.0694524160333842,
-0.317756917347296));
#40125=CARTESIAN_POINT('Ctrl Pts',(-0.137951847355649,-0.0835975873562079,
-0.309879281347913));
#40126=CARTESIAN_POINT('Ctrl Pts',(-0.00581383595771093,-0.161200087196222,
-0.302001645348528));
#40127=CARTESIAN_POINT('Ctrl Pts',(0.131571209749827,-0.0933181952546669,
-0.294124009349145));
#40128=CARTESIAN_POINT('Ctrl Pts',(0.150212166918945,0.0587841280459866,
-0.28624637334976));
#40129=CARTESIAN_POINT('Ctrl Pts',(0.033285419861052,0.157833296947363,
-0.278368737350377));
#40130=CARTESIAN_POINT('Ctrl Pts',(-0.113681689754523,0.114436629691781,
-0.270491101350993));
#40131=CARTESIAN_POINT('Ctrl Pts',(-0.158050148349798,-0.0322400280270659,
-0.262613465351609));
#40132=CARTESIAN_POINT('Ctrl Pts',(-0.059777060631363,-0.149819797833307,
-0.254735829352225));
#40133=CARTESIAN_POINT('Ctrl Pts',(0.0924453112337102,-0.132185979709678,
-0.246858193352841));
#40134=CARTESIAN_POINT('Ctrl Pts',(0.16123503667694,0.00474676185131575,
-0.238980557353457));
#40135=CARTESIAN_POINT('Ctrl Pts',(0.0845088281512594,0.137395512171083,
-0.231102921354073));
#40136=CARTESIAN_POINT('Ctrl Pts',(-0.0684872861712815,0.146043693583278,
-0.223225285354689));
#40137=CARTESIAN_POINT('Ctrl Pts',(-0.159673066834149,0.022886251891861,
-0.215347649355305));
#40138=CARTESIAN_POINT('Ctrl Pts',(-0.106752604056362,-0.120926218523974,
-0.207470013355921));
#40139=CARTESIAN_POINT('Ctrl Pts',(0.0425129535051184,-0.155601791755286,
-0.199592377356537));
#40140=CARTESIAN_POINT('Ctrl Pts',(0.153410224138463,-0.0498454803253261,
-0.191714741357153));
#40141=CARTESIAN_POINT('Ctrl Pts',(0.125853518028762,0.100896782901857,
-0.183837105357769));
#40142=CARTESIAN_POINT('Ctrl Pts',(-0.0152870135990733,0.160578878108339,
-0.175959469358385));
#40143=CARTESIAN_POINT('Ctrl Pts',(-0.14263089029847,0.075337226991929,
-0.168081833359001));
#40144=CARTESIAN_POINT('Ctrl Pts',(-0.141249227876074,-0.0778968836327328,
-0.160204197359617));
#40145=CARTESIAN_POINT('Ctrl Pts',(-0.0123889844412741,-0.160828425154002,
-0.152326561360233));
#40146=CARTESIAN_POINT('Ctrl Pts',(0.127652414035256,-0.0986109974054438,
-0.144448925360849));
#40147=CARTESIAN_POINT('Ctrl Pts',(0.15248647726015,0.0526036482907394,
-0.136571289361465));
#40148=CARTESIAN_POINT('Ctrl Pts',(0.0397002370073691,0.156343092795492,
-0.128693653362081));
#40149=CARTESIAN_POINT('Ctrl Pts',(-0.108915760812993,0.118981584750951,
-0.120816017362697));
#40150=CARTESIAN_POINT('Ctrl Pts',(-0.159234453765061,-0.0257617009453798,
-0.112938381363313));
#40151=CARTESIAN_POINT('Ctrl Pts',(-0.065842647850672,-0.147254978053657,
-0.105060745363929));
#40152=CARTESIAN_POINT('Ctrl Pts',(0.0869724802862671,-0.135849178901503,
-0.0971831093645453));
#40153=CARTESIAN_POINT('Ctrl Pts',(0.161294623704445,-0.00183888141316458,
-0.0893054733651615));
#40154=CARTESIAN_POINT('Ctrl Pts',(0.090046319753195,0.133831956670155,
-0.0814278373657774));
#40155=CARTESIAN_POINT('Ctrl Pts',(-0.0624681236721457,0.148716587042417,
-0.0735502013663936));
#40156=CARTESIAN_POINT('Ctrl Pts',(-0.158607231908194,0.029386661669371,
-0.0656725653670094));
#40157=CARTESIAN_POINT('Ctrl Pts',(-0.111596976643804,-0.116471378269128,
-0.0577949293676256));
#40158=CARTESIAN_POINT('Ctrl Pts',(0.0361208744551059,-0.157200866188131,
-0.0499172933682415));
#40159=CARTESIAN_POINT('Ctrl Pts',(0.151257553472499,-0.0560784438372532,
-0.0420396573688577));
#40160=CARTESIAN_POINT('Ctrl Pts',(0.129848444836529,0.0956992426875821,
-0.0341620213694736));
#40161=CARTESIAN_POINT('Ctrl Pts',(-0.00868406135992968,0.161023746827609,
-0.0262843853700897));
#40162=CARTESIAN_POINT('Ctrl Pts',(-0.139505319986123,0.081184151537233,
-0.0184067493707057));
#40163=CARTESIAN_POINT('Ctrl Pts',(-0.144173436655933,-0.0722467385446291,
-0.0105291133713217));
#40164=CARTESIAN_POINT('Ctrl Pts',(-0.0609053537800685,-0.130575908881668,
-0.00527735603839902));
#40165=CARTESIAN_POINT('Ctrl Pts',(-0.0160685904325677,-0.135878184512858,
-0.00265147737193768));
#40166=CARTESIAN_POINT('Ctrl Pts',(0.128823493644032,-0.0694465980833189,
-0.73765));
#40167=CARTESIAN_POINT('Ctrl Pts',(0.15173931854053,-0.0269377250156994,
-0.735024121333539));
#40168=CARTESIAN_POINT('Ctrl Pts',(0.151856046966723,0.0818050594551139,
-0.729772364000616));
#40169=CARTESIAN_POINT('Ctrl Pts',(0.0146738748916663,0.172019794370874,
-0.721894728001232));
#40170=CARTESIAN_POINT('Ctrl Pts',(-0.135622470260348,0.106569899584644,
-0.714017092001848));
#40171=CARTESIAN_POINT('Ctrl Pts',(-0.163581938544947,-0.0548506908475362,
-0.706139456002465));
#40172=CARTESIAN_POINT('Ctrl Pts',(-0.04387447660963,-0.16687728581957,
-0.698261820003079));
#40173=CARTESIAN_POINT('Ctrl Pts',(0.115412804073391,-0.128238419986997,
-0.690384184003697));
#40174=CARTESIAN_POINT('Ctrl Pts',(0.170548163154853,0.0261064927122433,
-0.682506548004312));
#40175=CARTESIAN_POINT('Ctrl Pts',(0.0717576404347894,0.156905962170951,
-0.674628912004929));
#40176=CARTESIAN_POINT('Ctrl Pts',(-0.0917922239173038,0.146088164952146,
-0.666751276005544));
#40177=CARTESIAN_POINT('Ctrl Pts',(-0.172500181369253,0.00342900790747846,
-0.65887364000616));
#40178=CARTESIAN_POINT('Ctrl Pts',(-0.0975246236996389,-0.142327172121431,
-0.650996004006776));
#40179=CARTESIAN_POINT('Ctrl Pts',(0.0654673347686249,-0.15963070124433,
-0.643118368007393));
#40180=CARTESIAN_POINT('Ctrl Pts',(0.169374683235426,-0.0328668636568096,
-0.635240732008008));
#40181=CARTESIAN_POINT('Ctrl Pts',(0.120419898872848,0.123559923738236,
-0.627363096008626));
#40182=CARTESIAN_POINT('Ctrl Pts',(-0.037214771683976,0.168472695765287,
-0.619485460009239));
#40183=CARTESIAN_POINT('Ctrl Pts',(-0.161262835785063,0.0613375810752176,
-0.611607824009858));
#40184=CARTESIAN_POINT('Ctrl Pts',(-0.139769862186219,-0.101155249406303,
-0.603730188010472));
#40185=CARTESIAN_POINT('Ctrl Pts',(0.00786654276560517,-0.17235461740462,
-0.595852552011089));
#40186=CARTESIAN_POINT('Ctrl Pts',(0.148403332894812,-0.0880025528866245,
-0.587974916011704));
#40187=CARTESIAN_POINT('Ctrl Pts',(0.155004904078945,0.0757725396329093,
-0.580097280012322));
#40188=CARTESIAN_POINT('Ctrl Pts',(0.0217132878452772,0.171162294134837,
-0.572219644012935));
#40189=CARTESIAN_POINT('Ctrl Pts',(-0.131174748136735,0.112076685932905,
-0.564342008013554));
#40190=CARTESIAN_POINT('Ctrl Pts',(-0.165676505100818,-0.0481590453130367,
-0.556464372014167));
#40191=CARTESIAN_POINT('Ctrl Pts',(-0.0506538668265696,-0.164930845323967,
-0.548586736014785));
#40192=CARTESIAN_POINT('Ctrl Pts',(0.110084298956909,-0.132851214243416,
-0.5407091000154));
#40193=CARTESIAN_POINT('Ctrl Pts',(0.171470488172567,0.0191277200101626,
-0.532831464016017));
#40194=CARTESIAN_POINT('Ctrl Pts',(0.0781031650900689,0.153843731065615,
-0.524953828016632));
#40195=CARTESIAN_POINT('Ctrl Pts',(-0.0857529007036231,0.14971452171228,
-0.51707619201725));
#40196=CARTESIAN_POINT('Ctrl Pts',(-0.172216275088487,0.0104667369622776,
-0.509198556017864));
#40197=CARTESIAN_POINT('Ctrl Pts',(-0.103253058387983,-0.138227363143328,
-0.501320920018481));
#40198=CARTESIAN_POINT('Ctrl Pts',(0.0588968845776194,-0.162170142060081,
-0.493443284019097));
#40199=CARTESIAN_POINT('Ctrl Pts',(0.16789190945479,-0.0397530467755856,
-0.485565648019713));
#40200=CARTESIAN_POINT('Ctrl Pts',(0.125363118452966,0.118541497038427,
-0.477688012020329));
#40201=CARTESIAN_POINT('Ctrl Pts',(-0.0303069081228627,0.169851374173085,
-0.469810376020944));
#40202=CARTESIAN_POINT('Ctrl Pts',(-0.158624703246786,0.0678690025582943,
-0.461932740021561));
#40203=CARTESIAN_POINT('Ctrl Pts',(-0.143782411581849,-0.095365696705413,
-0.454055104022176));
#40204=CARTESIAN_POINT('Ctrl Pts',(0.000824677743651456,-0.172532077872582,
-0.446177468022794));
#40205=CARTESIAN_POINT('Ctrl Pts',(0.14468748868791,-0.0939868533657117,
-0.438299832023408));
#40206=CARTESIAN_POINT('Ctrl Pts',(0.157968662510953,0.0693822718920721,
-0.430422196024026));
#40207=CARTESIAN_POINT('Ctrl Pts',(0.0286818316530525,0.170133331600341,
-0.42254456002464));
#40208=CARTESIAN_POINT('Ctrl Pts',(-0.126490585905224,0.117337673684787,
-0.414666924025258));
#40209=CARTESIAN_POINT('Ctrl Pts',(-0.167504219330098,-0.0413561905283752,
-0.406789288025872));
#40210=CARTESIAN_POINT('Ctrl Pts',(-0.057343930371003,-0.1627257559147,
-0.39891165202649));
#40211=CARTESIAN_POINT('Ctrl Pts',(0.104569722854182,-0.137234001073365,
-0.391034016027105));
#40212=CARTESIAN_POINT('Ctrl Pts',(0.172108349410229,0.0121125576032212,
-0.383156380027722));
#40213=CARTESIAN_POINT('Ctrl Pts',(0.0843177886811427,0.150527434377681,
-0.375278744028337));
#40214=CARTESIAN_POINT('Ctrl Pts',(-0.079570263159802,0.153090075475469,
-0.367401108028953));
#40215=CARTESIAN_POINT('Ctrl Pts',(-0.171645504343801,0.0174876764313346,
-0.359523472029569));
#40216=CARTESIAN_POINT('Ctrl Pts',(-0.108809279685313,-0.133897493041387,
-0.351645836030186));
#40217=CARTESIAN_POINT('Ctrl Pts',(0.0522282062165519,-0.164439084355898,
-0.343768200030801));
#40218=CARTESIAN_POINT('Ctrl Pts',(0.166129310572857,-0.046573062568317,
-0.335890564031418));
#40219=CARTESIAN_POINT('Ctrl Pts',(0.130097358898192,0.11332552755721,-0.328012928032033));
#40220=CARTESIAN_POINT('Ctrl Pts',(-0.0233485189157071,0.170946905946985,
-0.32013529203265));
#40221=CARTESIAN_POINT('Ctrl Pts',(-0.155722168218232,0.0742873092379748,
-0.312257656033265));
#40222=CARTESIAN_POINT('Ctrl Pts',(-0.147555292238255,-0.0894171891802003,
-0.304380020033882));
#40223=CARTESIAN_POINT('Ctrl Pts',(-0.00621856307261924,-0.172421945997932,
-0.296502384034497));
#40224=CARTESIAN_POINT('Ctrl Pts',(0.140730469920608,-0.0998144920556959,
-0.288624748035114));
#40225=CARTESIAN_POINT('Ctrl Pts',(0.160669107462727,0.0628763540254339,
-0.280747112035729));
#40226=CARTESIAN_POINT('Ctrl Pts',(0.0356025667580126,0.168820778426797,
-0.272869476036346));
#40227=CARTESIAN_POINT('Ctrl Pts',(-0.121595580453677,0.122403075135335,
-0.264991840036961));
#40228=CARTESIAN_POINT('Ctrl Pts',(-0.169052725824908,-0.0344844005244726,
-0.257114204037578));
#40229=CARTESIAN_POINT('Ctrl Pts',(-0.0639384090875212,-0.16024942381074,
-0.249236568038193));
#40230=CARTESIAN_POINT('Ctrl Pts',(0.0988808426753398,-0.141388036766026,
-0.24135893203881));
#40231=CARTESIAN_POINT('Ctrl Pts',(0.172459328468264,0.00507720516674541,
-0.233481296039426));
#40232=CARTESIAN_POINT('Ctrl Pts',(0.0903918655211907,0.146960228074094,
-0.225603660040042));
#40233=CARTESIAN_POINT('Ctrl Pts',(-0.0732549923710354,0.156210448060755,
-0.217726024040658));
#40234=CARTESIAN_POINT('Ctrl Pts',(-0.170788622921086,0.0244794662113939,
-0.209848388041274));
#40235=CARTESIAN_POINT('Ctrl Pts',(-0.114184130119851,-0.129344433261344,
-0.20197075204189));
#40236=CARTESIAN_POINT('Ctrl Pts',(0.0454724702757093,-0.166433928181152,
-0.194093116042506));
#40237=CARTESIAN_POINT('Ctrl Pts',(0.164089795743936,-0.0533154470718918,
-0.186215480043122));
#40238=CARTESIAN_POINT('Ctrl Pts',(0.134614744114814,0.107920659073171,
-0.178337844043738));
#40239=CARTESIAN_POINT('Ctrl Pts',(-0.0163512109645475,0.171757491767992,
-0.170460208044354));
#40240=CARTESIAN_POINT('Ctrl Pts',(-0.152560064280512,0.0805817881985668,
-0.16258257204497));
#40241=CARTESIAN_POINT('Ctrl Pts',(-0.151082218159426,-0.0833196339824615,
-0.154704936045586));
#40242=CARTESIAN_POINT('Ctrl Pts',(-0.013251437039873,-0.172024410899238,
-0.146827300046202));
#40243=CARTESIAN_POINT('Ctrl Pts',(0.136538869315254,-0.105475749828517,
-0.138949664046818));
#40244=CARTESIAN_POINT('Ctrl Pts',(0.163101742715315,0.056265623441254,
-0.131072028047434));
#40245=CARTESIAN_POINT('Ctrl Pts',(0.0424639480067868,0.167226834501153,
-0.12319439204805));
#40246=CARTESIAN_POINT('Ctrl Pts',(-0.116497873889869,0.127264424836848,
-0.115316756048666));
#40247=CARTESIAN_POINT('Ctrl Pts',(-0.170319476035203,-0.0275550881297732,
-0.107439120049282));
#40248=CARTESIAN_POINT('Ctrl Pts',(-0.0704262489526473,-0.157506055458817,
-0.0995614840498983));
#40249=CARTESIAN_POINT('Ctrl Pts',(0.0930270234964012,-0.145306247631903,
-0.0916838480505141));
#40250=CARTESIAN_POINT('Ctrl Pts',(0.172523063615169,-0.00196689417004758,
-0.0838062120511303));
#40251=CARTESIAN_POINT('Ctrl Pts',(0.0963148466718817,0.143148597541948,
-0.0759285760517462));
#40252=CARTESIAN_POINT('Ctrl Pts',(-0.0668168090584207,0.159069413584198,
-0.0680509400523624));
#40253=CARTESIAN_POINT('Ctrl Pts',(-0.169648590460546,0.0314323985771063,
-0.0601733040529782));
#40254=CARTESIAN_POINT('Ctrl Pts',(-0.119365741142487,-0.124579471658591,
-0.0522956680535945));
#40255=CARTESIAN_POINT('Ctrl Pts',(0.0386354100237868,-0.168144321334793,
-0.0444180320542104));
#40256=CARTESIAN_POINT('Ctrl Pts',(0.161787268048238,-0.059982315041711,
-0.0365403960548265));
#40257=CARTESIAN_POINT('Ctrl Pts',(0.138887775639146,0.102361294846172,
-0.0286627600554425));
#40258=CARTESIAN_POINT('Ctrl Pts',(-0.00928859769797627,0.172233329787836,
-0.0207851240560585));
#40259=CARTESIAN_POINT('Ctrl Pts',(-0.149216909044174,0.0868357433033009,
-0.0129074880566745));
#40260=CARTESIAN_POINT('Ctrl Pts',(-0.154209994186705,-0.0772761570327524,
-0.00502985205729055));
#40261=CARTESIAN_POINT('Ctrl Pts',(-0.0651452477669514,-0.139665881708986,
0.000221905275632163));
#40262=CARTESIAN_POINT('Ctrl Pts',(-0.0171871968558845,-0.145337272453549,
0.00284778394209351));
#40263=CARTESIAN_POINT('Ctrl Pts',(-0.146417921947427,0.000120753153388515,
-0.0587155045842908));
#40264=CARTESIAN_POINT('Ctrl Pts',(-0.146069418978064,-0.0391769882200356,
-0.0565755590740587));
#40265=CARTESIAN_POINT('Ctrl Pts',(-0.129702676035881,-0.0787309748396744,
-0.0544356135638267));
#40266=CARTESIAN_POINT('Ctrl Pts',(-0.101412690834453,-0.10583830156534,
-0.0522956680535946));
#40267=CARTESIAN_POINT('Ctrl Pts',(-0.0666986907537308,-0.139101088217324,
-0.0496697893871332));
#40268=CARTESIAN_POINT('Ctrl Pts',(-0.0140316403649711,-0.153622704776059,
-0.0470439107206718));
#40269=CARTESIAN_POINT('Ctrl Pts',(0.0328271945001503,-0.142856512006579,
-0.0444180320542104));
#40270=CARTESIAN_POINT('Ctrl Pts',(0.0796860293652709,-0.132090319237099,
-0.0417921533877491));
#40271=CARTESIAN_POINT('Ctrl Pts',(0.120736648706754,-0.0960363171394056,
-0.0391662747212878));
#40272=CARTESIAN_POINT('Ctrl Pts',(0.137445376309314,-0.0509520477759113,
-0.0365403960548265));
#40273=CARTESIAN_POINT('Ctrl Pts',(0.154154103911874,-0.00586777841241708,
-0.0339145173883652));
#40274=CARTESIAN_POINT('Ctrl Pts',(0.14652093977551,0.0482467582168783,
-0.0312886387219038));
#40275=CARTESIAN_POINT('Ctrl Pts',(0.118008295484474,0.0869493656884694,
-0.0286627600554425));
#40276=CARTESIAN_POINT('Ctrl Pts',(0.0894956511934385,0.12565197316006,
-0.0260368813889812));
#40277=CARTESIAN_POINT('Ctrl Pts',(0.0401035267477311,0.148942651473948,
-0.0234110027225198));
#40278=CARTESIAN_POINT('Ctrl Pts',(-0.00791392069948822,0.146355059550136,
-0.0207851240560585));
#40279=CARTESIAN_POINT('Ctrl Pts',(-0.0514054509527252,0.144011362864443,
-0.0184067493707056));
#40280=CARTESIAN_POINT('Ctrl Pts',(-0.0937692336261515,0.120437837890111,
-0.0160283746853528));
#40281=CARTESIAN_POINT('Ctrl Pts',(-0.119316161853458,0.0851151957093249,
-0.0136499999999998));
#40282=CARTESIAN_POINT('',(-0.000884750838570857,0.117943724677159,-0.73765));
#40283=CARTESIAN_POINT('Ctrl Pts',(-0.000884750838570857,0.117943724677159,
-0.73765));
#40284=CARTESIAN_POINT('Ctrl Pts',(0.00278616629908432,0.118427354462138,
-0.73765));
#40285=CARTESIAN_POINT('Ctrl Pts',(0.00647167956003039,0.118727197682349,
-0.73765));
#40286=CARTESIAN_POINT('Ctrl Pts',(0.0101595898828385,0.118837906739275,
-0.73765));
#40287=CARTESIAN_POINT('Ctrl Pts',(0.0154982204910781,0.118998169519057,
-0.73765));
#40288=CARTESIAN_POINT('Ctrl Pts',(0.0208418519924889,0.118762501178767,
-0.73765));
#40289=CARTESIAN_POINT('Ctrl Pts',(0.026159529311872,0.118157056568905,
-0.73765));
#40290=CARTESIAN_POINT('Ctrl Pts',(0.0298727943515444,0.117734282457535,
-0.73765));
#40291=CARTESIAN_POINT('Ctrl Pts',(0.0335752445366655,0.117130286443933,
-0.73765));
#40292=CARTESIAN_POINT('Ctrl Pts',(0.0372395824352719,0.116356599132226,
-0.73765));
#40293=CARTESIAN_POINT('Ctrl Pts',(0.0440678843012388,0.114914873325166,
-0.73765));
#40294=CARTESIAN_POINT('Ctrl Pts',(0.0507761145954882,0.112884283325685,
-0.73765));
#40295=CARTESIAN_POINT('Ctrl Pts',(0.0572985626748901,0.110316011463869,
-0.73765));
#40296=CARTESIAN_POINT('Ctrl Pts',(0.0611801597768471,0.108787598129718,
-0.73765));
#40297=CARTESIAN_POINT('Ctrl Pts',(0.0649985389765126,0.107066533179972,
-0.73765));
#40298=CARTESIAN_POINT('Ctrl Pts',(0.0687175636740839,0.105173564435539,
-0.73765));
#40299=CARTESIAN_POINT('Ctrl Pts',(0.0771723185211559,0.100870127924939,
-0.73765));
#40300=CARTESIAN_POINT('Ctrl Pts',(0.0851385654920254,0.095673845814644,
-0.73765));
#40301=CARTESIAN_POINT('Ctrl Pts',(0.092460845720161,0.0896941979495885,
-0.73765));
#40302=CARTESIAN_POINT('Ctrl Pts',(0.0953295505232922,0.087351506326615,
-0.73765));
#40303=CARTESIAN_POINT('Ctrl Pts',(0.0980993075401888,0.0848880166213253,
-0.73765));
#40304=CARTESIAN_POINT('Ctrl Pts',(0.100759943103025,0.082308310166907,
-0.73765));
#40305=CARTESIAN_POINT('Ctrl Pts',(0.102972427973208,0.0801631229117881,
-0.73765));
#40306=CARTESIAN_POINT('Ctrl Pts',(0.105109190100999,0.0779373067134747,
-0.73765));
#40307=CARTESIAN_POINT('Ctrl Pts',(0.107154943682283,0.0756446505534301,
-0.73765));
#40308=CARTESIAN_POINT('Ctrl Pts',(0.110688967967185,0.0716841038773035,
-0.73765));
#40309=CARTESIAN_POINT('Ctrl Pts',(0.113959348635532,0.0675170854532638,
-0.73765));
#40310=CARTESIAN_POINT('Ctrl Pts',(0.116939708255812,0.0631610811162178,
-0.73765));
#40311=CARTESIAN_POINT('Ctrl Pts',(0.12057791194668,0.0578435915929273,
-0.73765));
#40312=CARTESIAN_POINT('Ctrl Pts',(0.123784383512494,0.0522446483168349,
-0.73765));
#40313=CARTESIAN_POINT('Ctrl Pts',(0.126564768603565,0.0464177189336189,
-0.73765));
#40314=CARTESIAN_POINT('Ctrl Pts',(0.127881821320869,0.0436575353884167,
-0.73765));
#40315=CARTESIAN_POINT('Ctrl Pts',(0.129103140600637,0.0408460784277879,
-0.73765));
#40316=CARTESIAN_POINT('Ctrl Pts',(0.130228617479411,0.0379885175969106,
-0.73765));
#40317=CARTESIAN_POINT('Ctrl Pts',(0.131421146659668,0.0349607124598609,
-0.73765));
#40318=CARTESIAN_POINT('Ctrl Pts',(0.132502923828134,0.0318888297538296,
-0.73765));
#40319=CARTESIAN_POINT('Ctrl Pts',(0.133473660931759,0.0287845863114225,
-0.73765));
#40320=CARTESIAN_POINT('Ctrl Pts',(0.13596121999,0.0208298178521682,-0.73765));
#40321=CARTESIAN_POINT('Ctrl Pts',(0.137724934662181,0.0126541835654583,
-0.73765));
#40322=CARTESIAN_POINT('Ctrl Pts',(0.138774959248534,0.00436662491368386,
-0.73765));
#40323=CARTESIAN_POINT('Ctrl Pts',(0.139475142462338,-0.00115973087531884,
-0.73765));
#40324=CARTESIAN_POINT('Ctrl Pts',(0.139857543532154,-0.00673626433291896,
-0.73765));
#40325=CARTESIAN_POINT('Ctrl Pts',(0.139919399280779,-0.0123331745591834,
-0.73765));
#40326=CARTESIAN_POINT('Ctrl Pts',(0.139954302158222,-0.0154913009423901,
-0.73765));
#40327=CARTESIAN_POINT('Ctrl Pts',(0.139886760375099,-0.0186552059838679,
-0.73765));
#40328=CARTESIAN_POINT('Ctrl Pts',(0.139717313713924,-0.0218061889195747,
-0.73765));
#40329=CARTESIAN_POINT('Ctrl Pts',(0.139162565153442,-0.0321221387031601,
-0.73765));
#40330=CARTESIAN_POINT('Ctrl Pts',(0.137520401557198,-0.0423353653549661,
-0.73765));
#40331=CARTESIAN_POINT('Ctrl Pts',(0.134789335766029,-0.0522596970838267,
-0.73765));
#40332=CARTESIAN_POINT('Ctrl Pts',(0.1331818334651,-0.0581011477515141,
-0.73765));
#40333=CARTESIAN_POINT('Ctrl Pts',(0.131196160006388,-0.0638428465505078,
-0.73765));
#40334=CARTESIAN_POINT('Ctrl Pts',(0.128823493644032,-0.0694465980833189,
-0.73765));
#40335=CARTESIAN_POINT('Ctrl Pts',(-0.00088475083857086,0.117943724677159,
-0.73765));
#40336=CARTESIAN_POINT('Ctrl Pts',(-0.0359625809725899,0.117451794425203,
-0.735271625314648));
#40337=CARTESIAN_POINT('Ctrl Pts',(-0.0971707523342012,0.0878186355611941,
-0.731126054823441));
#40338=CARTESIAN_POINT('Ctrl Pts',(-0.117482453641731,0.0261030598409213,
-0.726980484332236));
#40339=CARTESIAN_POINT('Ctrl Pts',(-0.117673801045155,-9.24777646016256E-5,
-0.725213288526384));
#40340=CARTESIAN_POINT('Origin',(-3.28582941601228E-18,0.,-0.73765));
#40341=CARTESIAN_POINT('',(-0.111717694016328,0.0372841450039317,-0.73765));
#40342=CARTESIAN_POINT('Ctrl Pts',(0.0262121662178384,-0.144200775921424,
-0.73765));
#40343=CARTESIAN_POINT('Ctrl Pts',(0.0216914116314411,-0.144617508648269,
-0.73765));
#40344=CARTESIAN_POINT('Ctrl Pts',(0.017160159126439,-0.144810578739906,
-0.73765));
#40345=CARTESIAN_POINT('Ctrl Pts',(0.012630831538952,-0.144770228896137,
-0.73765));
#40346=CARTESIAN_POINT('Ctrl Pts',(0.00502278391791575,-0.144702452051349,
-0.73765));
#40347=CARTESIAN_POINT('Ctrl Pts',(-0.00258026785134787,-0.143976762872906,
-0.73765));
#40348=CARTESIAN_POINT('Ctrl Pts',(-0.0101072259685224,-0.142628707009231,
-0.73765));
#40349=CARTESIAN_POINT('Ctrl Pts',(-0.0135423586684204,-0.142013484935917,
-0.73765));
#40350=CARTESIAN_POINT('Ctrl Pts',(-0.0169589000212732,-0.141268716329859,
-0.73765));
#40351=CARTESIAN_POINT('Ctrl Pts',(-0.0203418084420799,-0.140400116655759,
-0.73765));
#40352=CARTESIAN_POINT('Ctrl Pts',(-0.0268350469323433,-0.138732904856054,
-0.73765));
#40353=CARTESIAN_POINT('Ctrl Pts',(-0.0332137854254147,-0.136608416932435,
-0.73765));
#40354=CARTESIAN_POINT('Ctrl Pts',(-0.0394282027288326,-0.134050378168974,
-0.73765));
#40355=CARTESIAN_POINT('Ctrl Pts',(-0.0426874420061282,-0.13270877846563,
-0.73765));
#40356=CARTESIAN_POINT('Ctrl Pts',(-0.0459032314063151,-0.131246864018571,
-0.73765));
#40357=CARTESIAN_POINT('Ctrl Pts',(-0.0490617852831597,-0.129670241929581,
-0.73765));
#40358=CARTESIAN_POINT('Ctrl Pts',(-0.0579717447200327,-0.125222751271541,
-0.73765));
#40359=CARTESIAN_POINT('Ctrl Pts',(-0.0663802608480417,-0.119890965737638,
-0.73765));
#40360=CARTESIAN_POINT('Ctrl Pts',(-0.074123276457021,-0.113753043432987,
-0.73765));
#40361=CARTESIAN_POINT('Ctrl Pts',(-0.0793760400744385,-0.109589154762658,
-0.73765));
#40362=CARTESIAN_POINT('Ctrl Pts',(-0.0843220259407665,-0.105053336421179,
-0.73765));
#40363=CARTESIAN_POINT('Ctrl Pts',(-0.0888980477470807,-0.100162202168974,
-0.73765));
#40364=CARTESIAN_POINT('Ctrl Pts',(-0.0907777300028143,-0.0981530818777209,
-0.73765));
#40365=CARTESIAN_POINT('Ctrl Pts',(-0.092593341574421,-0.0960852887450699,
-0.73765));
#40366=CARTESIAN_POINT('Ctrl Pts',(-0.0943350874707246,-0.0939670993988704,
-0.73765));
#40367=CARTESIAN_POINT('Ctrl Pts',(-0.0976089573306515,-0.0899856482165493,
-0.73765));
#40368=CARTESIAN_POINT('Ctrl Pts',(-0.100628388290881,-0.0858197177372537,
-0.73765));
#40369=CARTESIAN_POINT('Ctrl Pts',(-0.10336682064894,-0.081478830271231,
-0.73765));
#40370=CARTESIAN_POINT('Ctrl Pts',(-0.106575782904835,-0.0763920717852811,
-0.73765));
#40371=CARTESIAN_POINT('Ctrl Pts',(-0.109399057782675,-0.0710649351750326,
-0.73765));
#40372=CARTESIAN_POINT('Ctrl Pts',(-0.111830948744127,-0.0655430594973256,
-0.73765));
#40373=CARTESIAN_POINT('Ctrl Pts',(-0.113091811307504,-0.0626801324862042,
-0.73765));
#40374=CARTESIAN_POINT('Ctrl Pts',(-0.114247330990164,-0.0597648360251877,
-0.73765));
#40375=CARTESIAN_POINT('Ctrl Pts',(-0.115295848804168,-0.0568035605001958,
-0.73765));
#40376=CARTESIAN_POINT('Ctrl Pts',(-0.116314386310609,-0.0539269568327871,
-0.73765));
#40377=CARTESIAN_POINT('Ctrl Pts',(-0.117229972470728,-0.0510120371908431,
-0.73765));
#40378=CARTESIAN_POINT('Ctrl Pts',(-0.118040228185711,-0.0480723152749109,
-0.73765));
#40379=CARTESIAN_POINT('Ctrl Pts',(-0.119975551423544,-0.0410506898405367,
-0.73765));
#40380=CARTESIAN_POINT('Ctrl Pts',(-0.121315904182743,-0.0338746385959458,
-0.73765));
#40381=CARTESIAN_POINT('Ctrl Pts',(-0.122051121145503,-0.0266271899647891,
-0.73765));
#40382=CARTESIAN_POINT('Ctrl Pts',(-0.122625570639283,-0.0209645170284367,
-0.73765));
#40383=CARTESIAN_POINT('Ctrl Pts',(-0.122830202791461,-0.0152581010368553,
-0.73765));
#40384=CARTESIAN_POINT('Ctrl Pts',(-0.122652104845954,-0.00954986495031056,
-0.73765));
#40385=CARTESIAN_POINT('Ctrl Pts',(-0.122569605793161,-0.00690567908438269,
-0.73765));
#40386=CARTESIAN_POINT('Ctrl Pts',(-0.122404760993965,-0.00426311687457716,
-0.73765));
#40387=CARTESIAN_POINT('Ctrl Pts',(-0.122157517869817,-0.00163526686520094,
-0.73765));
#40388=CARTESIAN_POINT('Ctrl Pts',(-0.121338098277213,0.00707402198368037,
-0.73765));
#40389=CARTESIAN_POINT('Ctrl Pts',(-0.119616360728985,0.0156516535710813,
-0.73765));
#40390=CARTESIAN_POINT('Ctrl Pts',(-0.116954245640549,0.0239432946408254,
-0.73765));
#40391=CARTESIAN_POINT('Ctrl Pts',(-0.115495686406583,0.028486242351667,
-0.73765));
#40392=CARTESIAN_POINT('Ctrl Pts',(-0.113754063897855,0.0329430069155385,
-0.73765));
#40393=CARTESIAN_POINT('Ctrl Pts',(-0.111717694016328,0.0372841450039292,
-0.73765));
#40394=CARTESIAN_POINT('Origin',(0.,0.,-0.73765));
#40395=CARTESIAN_POINT('Origin',(0.,0.,-0.860086711473615));
#40396=CARTESIAN_POINT('Ctrl Pts',(-0.111717694016328,0.037284145003932,
-0.73765));
#40397=CARTESIAN_POINT('Ctrl Pts',(-0.115720921699071,0.0252889292013099,
-0.736795570491205));
#40398=CARTESIAN_POINT('Ctrl Pts',(-0.117632122859214,0.0126318657558966,
-0.735941140982411));
#40399=CARTESIAN_POINT('Ctrl Pts',(-0.11756447877375,-3.10001368070065E-5,
-0.735086711473616));
#40400=CARTESIAN_POINT('Ctrl Pts',(-0.138823048348881,0.0463301602320166,
-0.754147783942094));
#40401=CARTESIAN_POINT('Ctrl Pts',(-0.154110965519853,0.000521657650733254,
-0.751521905275632));
#40402=CARTESIAN_POINT('Ctrl Pts',(-0.135580905218918,-0.106630820062224,
-0.746270147942711));
#40403=CARTESIAN_POINT('Ctrl Pts',(0.0150378134171585,-0.171988340881595,
-0.738392511943325));
#40404=CARTESIAN_POINT('Ctrl Pts',(0.151886514761348,-0.081737977277168,
-0.730514875943943));
#40405=CARTESIAN_POINT('Ctrl Pts',(0.151754795995761,0.0820861101213215,
-0.722637239944558));
#40406=CARTESIAN_POINT('Ctrl Pts',(0.0146120564079159,0.171928721992484,
-0.714759603945174));
#40407=CARTESIAN_POINT('Ctrl Pts',(-0.13569138198474,0.106550741701972,
-0.70688196794579));
#40408=CARTESIAN_POINT('Ctrl Pts',(-0.16354633841588,-0.05496199688411,
-0.699004331946406));
#40409=CARTESIAN_POINT('Ctrl Pts',(-0.0437919749452907,-0.16688590131284,
-0.691126695947022));
#40410=CARTESIAN_POINT('Ctrl Pts',(0.115481099091748,-0.128186123155717,
-0.683249059947638));
#40411=CARTESIAN_POINT('Ctrl Pts',(0.170533594917282,0.0261985716909196,
-0.675371423948254));
#40412=CARTESIAN_POINT('Ctrl Pts',(0.0716770510023252,0.156941001890843,
-0.667493787948871));
#40413=CARTESIAN_POINT('Ctrl Pts',(-0.0918680462662227,0.14604176284845,
-0.659616151949486));
#40414=CARTESIAN_POINT('Ctrl Pts',(-0.17250178293021,0.00333924143125606,
-0.651738515950102));
#40415=CARTESIAN_POINT('Ctrl Pts',(-0.0974510977380058,-0.14237728741126,
-0.643860879950718));
#40416=CARTESIAN_POINT('Ctrl Pts',(0.0655499140182738,-0.159596988908127,
-0.635983243951334));
#40417=CARTESIAN_POINT('Ctrl Pts',(0.16939163808025,-0.0327791950909268,
-0.628105607951951));
#40418=CARTESIAN_POINT('Ctrl Pts',(0.12035600598554,0.123622135200244,-0.620227971952565));
#40419=CARTESIAN_POINT('Ctrl Pts',(-0.0373018898023092,0.168453457330507,
-0.612350335953183));
#40420=CARTESIAN_POINT('Ctrl Pts',(-0.161294532557813,0.0612541747614786,
-0.604472699953798));
#40421=CARTESIAN_POINT('Ctrl Pts',(-0.139717542474164,-0.10122750617809,
-0.596595063954415));
#40422=CARTESIAN_POINT('Ctrl Pts',(0.00795566602636565,-0.172350534702269,
-0.58871742795503));
#40423=CARTESIAN_POINT('Ctrl Pts',(0.148448822061392,-0.0879258035956179,
-0.580839791955647));
#40424=CARTESIAN_POINT('Ctrl Pts',(0.154965706478682,0.0758526824482954,
-0.572962155956262));
#40425=CARTESIAN_POINT('Ctrl Pts',(0.0216247787522968,0.171173504196391,
-0.565084519956878));
#40426=CARTESIAN_POINT('Ctrl Pts',(-0.131232688082165,0.112008844349949,
-0.557206883957495));
#40427=CARTESIAN_POINT('Ctrl Pts',(-0.165651584869631,-0.0482447100545612,
-0.549329247958111));
#40428=CARTESIAN_POINT('Ctrl Pts',(-0.0505685770021586,-0.164957020573233,
-0.541451611958726));
#40429=CARTESIAN_POINT('Ctrl Pts',(0.110152983545764,-0.132794276374095,
-0.533573975959343));
#40430=CARTESIAN_POINT('Ctrl Pts',(0.171460579160472,0.0192163839752785,
-0.525696339959958));
#40431=CARTESIAN_POINT('Ctrl Pts',(0.0780236054224529,0.153884101245222,
-0.517818703960575));
#40432=CARTESIAN_POINT('Ctrl Pts',(-0.0858303077688239,0.149670163653888,
-0.50994106796119));
#40433=CARTESIAN_POINT('Ctrl Pts',(-0.172221669049576,0.010377684194152,
-0.502063431961807));
#40434=CARTESIAN_POINT('Ctrl Pts',(-0.103181571148412,-0.138280739782684,
-0.494185795962423));
#40435=CARTESIAN_POINT('Ctrl Pts',(0.0589807352003881,-0.162139669713528,
-0.486308159963038));
#40436=CARTESIAN_POINT('Ctrl Pts',(0.167912447591442,-0.0396662269869119,
-0.478430523963655));
#40437=CARTESIAN_POINT('Ctrl Pts',(0.125301808267477,0.118606308704212,
-0.470552887964271));
#40438=CARTESIAN_POINT('Ctrl Pts',(-0.0303947336884643,0.169835684658897,
-0.462675251964886));
#40439=CARTESIAN_POINT('Ctrl Pts',(-0.158659780904255,0.0677869717788998,
-0.454797615965503));
#40440=CARTESIAN_POINT('Ctrl Pts',(-0.14373308345953,-0.0954400353036286,
-0.446919979966119));
#40441=CARTESIAN_POINT('Ctrl Pts',(0.000913892613523542,-0.172531633099076,
-0.439042343966734));
#40442=CARTESIAN_POINT('Ctrl Pts',(0.144736073158576,-0.0939120266322549,
-0.431164707967351));
#40443=CARTESIAN_POINT('Ctrl Pts',(0.157932768701871,0.0694639488490502,
-0.423287071967967));
#40444=CARTESIAN_POINT('Ctrl Pts',(0.0285938540193059,0.170148144661836,
-0.415409435968583));
#40445=CARTESIAN_POINT('Ctrl Pts',(-0.126551246832543,0.117272253942145,
-0.407531799969199));
#40446=CARTESIAN_POINT('Ctrl Pts',(-0.167482816569958,-0.0414428012245345,
-0.399654163969815));
#40447=CARTESIAN_POINT('Ctrl Pts',(-0.0572597800887704,-0.162755390705586,
-0.391776527970431));
#40448=CARTESIAN_POINT('Ctrl Pts',(0.104640674343329,-0.137179914318808,
-0.383898891971047));
#40449=CARTESIAN_POINT('Ctrl Pts',(0.172102067809386,0.0122015521666594,
-0.376021255971662));
#40450=CARTESIAN_POINT('Ctrl Pts',(0.0842399431862384,0.150571018431575,
-0.368143619972279));
#40451=CARTESIAN_POINT('Ctrl Pts',(-0.0796494163555106,0.153048914056156,
-0.360265983972895));
#40452=CARTESIAN_POINT('Ctrl Pts',(-0.17165452883643,0.0173989180550344,
-0.352388347973511));
#40453=CARTESIAN_POINT('Ctrl Pts',(-0.108740030796753,-0.133953743217066,
-0.344510711974127));
#40454=CARTESIAN_POINT('Ctrl Pts',(0.0523132308002934,-0.164412060089207,
-0.336633075974743));
#40455=CARTESIAN_POINT('Ctrl Pts',(0.166153375472371,-0.0464871534800791,
-0.328755439975359));
#40456=CARTESIAN_POINT('Ctrl Pts',(0.130038745345635,0.113392787815077,
-0.320877803975975));
#40457=CARTESIAN_POINT('Ctrl Pts',(-0.023436911711692,0.170934814443863,
-0.313000167976591));
#40458=CARTESIAN_POINT('Ctrl Pts',(-0.155760565039272,0.0742067786539452,
-0.305122531977207));
#40459=CARTESIAN_POINT('Ctrl Pts',(-0.147509039640546,-0.0894934793371125,
-0.297244895977823));
#40460=CARTESIAN_POINT('Ctrl Pts',(-0.00612940440244159,-0.172425143239602,
-0.289367259978439));
#40461=CARTESIAN_POINT('Ctrl Pts',(0.140782068237328,-0.0997417108456163,
-0.281489623979055));
#40462=CARTESIAN_POINT('Ctrl Pts',(0.160636577524524,0.0629594280525857,
-0.273611987979671));
#40463=CARTESIAN_POINT('Ctrl Pts',(0.0355152670997055,0.168839170284302,
-0.265734351980287));
#40464=CARTESIAN_POINT('Ctrl Pts',(-0.121658861180512,0.122340186022964,
-0.257856715980903));
#40465=CARTESIAN_POINT('Ctrl Pts',(-0.169034876246628,-0.0345718126723981,
-0.249979079981519));
#40466=CARTESIAN_POINT('Ctrl Pts',(-0.0638555385981163,-0.160282468815134,
-0.242101443982135));
#40467=CARTESIAN_POINT('Ctrl Pts',(0.0989539427921171,-0.141336891247995,
-0.234223807982751));
#40468=CARTESIAN_POINT('Ctrl Pts',(0.172456684746421,0.00516638197338353,
-0.226346171983367));
#40469=CARTESIAN_POINT('Ctrl Pts',(0.0903158639700122,0.14700695335058,
-0.218468535983983));
#40470=CARTESIAN_POINT('Ctrl Pts',(-0.0733357597872231,0.15617255191074,
-0.210590899984599));
#40471=CARTESIAN_POINT('Ctrl Pts',(-0.170801262847335,0.0243911501310009,
-0.202713263985215));
#40472=CARTESIAN_POINT('Ctrl Pts',(-0.114117235117242,-0.129403463123037,
-0.194835627985831));
#40473=CARTESIAN_POINT('Ctrl Pts',(0.04555852729765,-0.166410397210689,
-0.186957991986448));
#40474=CARTESIAN_POINT('Ctrl Pts',(0.164117346908928,-0.0532305915583867,
-0.179080355987063));
#40475=CARTESIAN_POINT('Ctrl Pts',(0.134558925626773,0.10799025519103,-0.17120271998768));
#40476=CARTESIAN_POINT('Ctrl Pts',(-0.0164400250396412,0.171749019605496,
-0.163325083988295));
#40477=CARTESIAN_POINT('Ctrl Pts',(-0.152601713625263,0.0805028898118418,
-0.155447447988912));
#40478=CARTESIAN_POINT('Ctrl Pts',(-0.151039123194672,-0.0833977442910985,
-0.147569811989528));
#40479=CARTESIAN_POINT('Ctrl Pts',(-0.0131624736632622,-0.172031252885583,
-0.139692175990144));
#40480=CARTESIAN_POINT('Ctrl Pts',(0.13659337737755,-0.10540512014574,-0.13181453999076));
#40481=CARTESIAN_POINT('Ctrl Pts',(0.163072665249414,0.0563499269687501,
-0.123936903991376));
#40482=CARTESIAN_POINT('Ctrl Pts',(0.042377406518749,0.167248829784194,
-0.116059267991992));
#40483=CARTESIAN_POINT('Ctrl Pts',(-0.116563544816227,0.127204066132066,
-0.108181631992608));
#40484=CARTESIAN_POINT('Ctrl Pts',(-0.170305445231403,-0.0276429564161484,
-0.100303995993224));
#40485=CARTESIAN_POINT('Ctrl Pts',(-0.0703443482700645,-0.157542834875204,
-0.0924263599938398));
#40486=CARTESIAN_POINT('Ctrl Pts',(0.0931012989163088,-0.145257407925471,
-0.0845487239944556));
#40487=CARTESIAN_POINT('Ctrl Pts',(0.172525680076593,-0.00187905314371138,
-0.0766710879950718));
#40488=CARTESIAN_POINT('Ctrl Pts',(0.096237741546027,0.143200988169951,
-0.0687934519956877));
#40489=CARTESIAN_POINT('Ctrl Pts',(-0.0668932145228675,0.159029901442989,
-0.0609158159963038));
#40490=CARTESIAN_POINT('Ctrl Pts',(-0.169675926294121,0.0313540695073055,
-0.0530381799969198));
#40491=CARTESIAN_POINT('Ctrl Pts',(-0.119280200416385,-0.124659060525867,
-0.0451605439975358));
#40492=CARTESIAN_POINT('Ctrl Pts',(0.03868209760446,-0.168090171100606,
-0.0372829079981519));
#40493=CARTESIAN_POINT('Ctrl Pts',(0.161895992042455,-0.0599650981168399,
-0.0294052719987679));
#40494=CARTESIAN_POINT('Ctrl Pts',(0.1386766030792,0.102572478792013,-0.0215276359993839));
#40495=CARTESIAN_POINT('Ctrl Pts',(0.040233477224662,0.148767365811789,
-0.0162758786664613));
#40496=CARTESIAN_POINT('Ctrl Pts',(-0.00798678478682508,0.146131905375825,
-0.0136499999999999));
#40497=CARTESIAN_POINT('Ctrl Pts',(-0.12978793023803,0.0433148218226551,
-0.748648522628063));
#40498=CARTESIAN_POINT('Ctrl Pts',(-0.144080853141469,0.000487706238889336,
-0.746022643961601));
#40499=CARTESIAN_POINT('Ctrl Pts',(-0.126756797790082,-0.0996908913905975,
-0.740770886628678));
#40500=CARTESIAN_POINT('Ctrl Pts',(0.0140590968281712,-0.16079470270669,
-0.732893250629295));
#40501=CARTESIAN_POINT('Ctrl Pts',(0.14200117787647,-0.0764181670034058,
-0.72501561462991));
#40502=CARTESIAN_POINT('Ctrl Pts',(0.141878031855961,0.0767436420727705,
-0.717137978630528));
#40503=CARTESIAN_POINT('Ctrl Pts',(0.0136610496618582,0.160738964035679,
-0.709260342631142));
#40504=CARTESIAN_POINT('Ctrl Pts',(-0.12686008431884,0.0996160248265959,
-0.701382706631759));
#40505=CARTESIAN_POINT('Ctrl Pts',(-0.152902137025984,-0.051384866577851,
-0.693505070632375));
#40506=CARTESIAN_POINT('Ctrl Pts',(-0.0409418310344329,-0.156024348801704,
-0.68562743463299));
#40507=CARTESIAN_POINT('Ctrl Pts',(0.107965161484308,-0.119843295529764,
-0.677749798633607));
#40508=CARTESIAN_POINT('Ctrl Pts',(0.159434636997316,0.0244934716201587,
-0.669872162634223));
#40509=CARTESIAN_POINT('Ctrl Pts',(0.0670120430706731,0.146726700264534,
-0.661994526634839));
#40510=CARTESIAN_POINT('Ctrl Pts',(-0.0858889335864435,0.136536824063813,
-0.654116890635455));
#40511=CARTESIAN_POINT('Ctrl Pts',(-0.161274728045275,0.00312191123219325,
-0.64623925463607));
#40512=CARTESIAN_POINT('Ctrl Pts',(-0.0911086193918861,-0.133110846259281,
-0.638361618636687));
#40513=CARTESIAN_POINT('Ctrl Pts',(0.0612836828530949,-0.149209825810416,
-0.630483982637303));
#40514=CARTESIAN_POINT('Ctrl Pts',(0.158367002940418,-0.0306458036782776,
-0.62260634663792));
#40515=CARTESIAN_POINT('Ctrl Pts',(0.112522791383474,0.115576348812938,
-0.614728710638535));
#40516=CARTESIAN_POINT('Ctrl Pts',(-0.0348741446682685,0.157489882468374,
-0.606851074639151));
#40517=CARTESIAN_POINT('Ctrl Pts',(-0.150796887032612,0.0572675262161885,
-0.598973438639767));
#40518=CARTESIAN_POINT('Ctrl Pts',(-0.130624207372924,-0.0946392451849487,
-0.591095802640384));
#40519=CARTESIAN_POINT('Ctrl Pts',(0.0074378818179544,-0.161133323612149,
-0.583218166640998));
#40520=CARTESIAN_POINT('Ctrl Pts',(0.138787222948753,-0.0822032666687414,
-0.575340530641615));
#40521=CARTESIAN_POINT('Ctrl Pts',(0.144879964393206,0.0709159089578964,
-0.567462894642231));
#40522=CARTESIAN_POINT('Ctrl Pts',(0.0202173580647961,0.160032898610667,
-0.559585258642847));
#40523=CARTESIAN_POINT('Ctrl Pts',(-0.122691578727996,0.104718893940429,
-0.551707622643464));
#40524=CARTESIAN_POINT('Ctrl Pts',(-0.154870366243849,-0.0451047656523092,
-0.543829986644079));
#40525=CARTESIAN_POINT('Ctrl Pts',(-0.0472773867326288,-0.154221006764145,
-0.535952350644695));
#40526=CARTESIAN_POINT('Ctrl Pts',(0.10298381943047,-0.124151533070622,
-0.528074714645311));
#40527=CARTESIAN_POINT('Ctrl Pts',(0.160301289672918,0.0179657105392391,
-0.520197078645928));
#40528=CARTESIAN_POINT('Ctrl Pts',(0.0729455402249881,0.143868754034011,
-0.512319442646543));
#40529=CARTESIAN_POINT('Ctrl Pts',(-0.0802441534709221,0.13992907510723,
-0.50444180664716));
#40530=CARTESIAN_POINT('Ctrl Pts',(-0.16101284501338,0.00970226607355439,
-0.496564170647775));
#40531=CARTESIAN_POINT('Ctrl Pts',(-0.0964661323702182,-0.129280917121734,
-0.488686534648391));
#40532=CARTESIAN_POINT('Ctrl Pts',(0.0551420505213066,-0.151587019532309,
-0.480808898649007));
#40533=CARTESIAN_POINT('Ctrl Pts',(0.156984083646731,-0.0370846020326892,
-0.472931262649624));
#40534=CARTESIAN_POINT('Ctrl Pts',(0.117146702536368,0.110886970881133,
-0.465053626650239));
#40535=CARTESIAN_POINT('Ctrl Pts',(-0.0284165318546242,0.158782149323222,
-0.457175990650856));
#40536=CARTESIAN_POINT('Ctrl Pts',(-0.14833361477434,0.0633751446098248,
-0.449298354651471));
#40537=CARTESIAN_POINT('Ctrl Pts',(-0.134378402079605,-0.0892284443486102,
-0.441420718652087));
#40538=CARTESIAN_POINT('Ctrl Pts',(0.000854413097680245,-0.161302635454603,
-0.433543082652704));
#40539=CARTESIAN_POINT('Ctrl Pts',(0.135316113494514,-0.0877998841404727,
-0.42566544665332));
#40540=CARTESIAN_POINT('Ctrl Pts',(0.147653919218541,0.0649429778016496,
-0.417787810653936));
#40541=CARTESIAN_POINT('Ctrl Pts',(0.0267328601038017,0.15907427327199,
-0.409910174654551));
#40542=CARTESIAN_POINT('Ctrl Pts',(-0.118314823012387,0.109639741343586,
-0.402032538655168));
#40543=CARTESIAN_POINT('Ctrl Pts',(-0.156582414603242,-0.0387455502394743,
-0.394154902655784));
#40544=CARTESIAN_POINT('Ctrl Pts',(-0.0535331015418237,-0.152162667121912,
-0.386277266656399));
#40545=CARTESIAN_POINT('Ctrl Pts',(0.0978302717254945,-0.128251737455899,
-0.378399630657016));
#40546=CARTESIAN_POINT('Ctrl Pts',(0.16090102786484,0.0114074299638081,
-0.370521994657631));
#40547=CARTESIAN_POINT('Ctrl Pts',(0.0787572957052066,0.140771298919715,
-0.362644358658248));
#40548=CARTESIAN_POINT('Ctrl Pts',(-0.0744655373614135,0.143087923920284,
-0.354766722658863));
#40549=CARTESIAN_POINT('Ctrl Pts',(-0.160482616385682,0.0162665320319777,
-0.34688908665948));
#40550=CARTESIAN_POINT('Ctrl Pts',(-0.101662826879164,-0.125235537517425,
-0.339011450660095));
#40551=CARTESIAN_POINT('Ctrl Pts',(0.0489084920003435,-0.153711514326653,
-0.331133814660712));
#40552=CARTESIAN_POINT('Ctrl Pts',(0.155339498455806,-0.0434615973687168,
-0.323256178661328));
#40553=CARTESIAN_POINT('Ctrl Pts',(0.121575342206467,0.106012765239481,
-0.315378542661944));
#40554=CARTESIAN_POINT('Ctrl Pts',(-0.0219115507000505,0.15980974367121,
-0.30750090666256));
#40555=CARTESIAN_POINT('Ctrl Pts',(-0.145623090614954,0.0693771266780044,
-0.299623270663176));
#40556=CARTESIAN_POINT('Ctrl Pts',(-0.137908605048293,-0.0836689122671714,
-0.291745634663792));
#40557=CARTESIAN_POINT('Ctrl Pts',(-0.00573048006398319,-0.161203076349563,
-0.283867998664408));
#40558=CARTESIAN_POINT('Ctrl Pts',(0.131619449857004,-0.0932501509152808,
-0.275990362665024));
#40559=CARTESIAN_POINT('Ctrl Pts',(0.150181754149593,0.0588617953077906,
-0.26811272666564));
#40560=CARTESIAN_POINT('Ctrl Pts',(0.0332038019878175,0.157850491794668,
-0.260235090666256));
#40561=CARTESIAN_POINT('Ctrl Pts',(-0.113740851937299,0.11437783363575,
-0.252357454666872));
#40562=CARTESIAN_POINT('Ctrl Pts',(-0.158033460488178,-0.0323217510686777,
-0.244479818667488));
#40563=CARTESIAN_POINT('Ctrl Pts',(-0.0596995836603153,-0.149850692146435,
-0.236602182668104));
#40564=CARTESIAN_POINT('Ctrl Pts',(0.0925136537241649,-0.132138162931375,
-0.22872454666872));
#40565=CARTESIAN_POINT('Ctrl Pts',(0.161232565018306,0.00483013470111595,
-0.220846910669336));
#40566=CARTESIAN_POINT('Ctrl Pts',(0.0844377730624996,0.13743919639353,
-0.212969274669952));
#40567=CARTESIAN_POINT('Ctrl Pts',(-0.0685627969449054,0.146008263855052,
-0.205091638670568));
#40568=CARTESIAN_POINT('Ctrl Pts',(-0.159684884107186,0.0228036837490541,
-0.197214002671184));
#40569=CARTESIAN_POINT('Ctrl Pts',(-0.106690062828264,-0.120981406503653,
-0.1893363666718));
#40570=CARTESIAN_POINT('Ctrl Pts',(0.042593409617363,-0.155579792267527,
-0.181458730672416));
#40571=CARTESIAN_POINT('Ctrl Pts',(0.153435982171603,-0.0497661475228981,
-0.173581094673032));
#40572=CARTESIAN_POINT('Ctrl Pts',(0.125801332414644,0.10096184944662,-0.165703458673648));
#40573=CARTESIAN_POINT('Ctrl Pts',(-0.0153700473252411,0.160570957345555,
-0.157825822674264));
#40574=CARTESIAN_POINT('Ctrl Pts',(-0.142669828949619,0.0752634636044082,
-0.14994818667488));
#40575=CARTESIAN_POINT('Ctrl Pts',(-0.141208937691226,-0.0779699102332057,
-0.142070550675496));
#40576=CARTESIAN_POINT('Ctrl Pts',(-0.0123058111306849,-0.160834821838537,
-0.134192914676112));
#40577=CARTESIAN_POINT('Ctrl Pts',(0.12770337451099,-0.0985449645639955,
-0.126315278676728));
#40578=CARTESIAN_POINT('Ctrl Pts',(0.152459292263417,0.0526824650324521,
-0.118437642677344));
#40579=CARTESIAN_POINT('Ctrl Pts',(0.039619327959875,0.156363656544054,
-0.110560006677961));
#40580=CARTESIAN_POINT('Ctrl Pts',(-0.108977157632254,0.118925154414212,
-0.102682370678576));
#40581=CARTESIAN_POINT('Ctrl Pts',(-0.159221336137934,-0.025843850438262,
-0.0948047346791926));
#40582=CARTESIAN_POINT('Ctrl Pts',(-0.0657660775678267,-0.147289363729415,
-0.0869270986798085));
#40583=CARTESIAN_POINT('Ctrl Pts',(0.0870419215867718,-0.135803517864042,
-0.0790494626804245));
#40584=CARTESIAN_POINT('Ctrl Pts',(0.16129706987687,-0.00175675740613725,
-0.0711718266810406));
#40585=CARTESIAN_POINT('Ctrl Pts',(0.089974232914486,0.133880937522061,
-0.0632941906816565));
#40586=CARTESIAN_POINT('Ctrl Pts',(-0.0625395563860025,0.14867964649769,
-0.0554165546822727));
#40587=CARTESIAN_POINT('Ctrl Pts',(-0.158632788624483,0.0293134305455207,
-0.0475389186828885));
#40588=CARTESIAN_POINT('Ctrl Pts',(-0.111517003224952,-0.116545787198168,
-0.0396612826835047));
#40589=CARTESIAN_POINT('Ctrl Pts',(0.0361645234351237,-0.157150240251728,
-0.0317836466841206));
#40590=CARTESIAN_POINT('Ctrl Pts',(0.151359201306518,-0.0560623474536147,
-0.0239060106847367));
#40591=CARTESIAN_POINT('Ctrl Pts',(0.129651016168851,0.0958966820001181,
-0.0160283746853527));
#40592=CARTESIAN_POINT('Ctrl Pts',(0.0376149335241836,0.139085034692163,
-0.0107766173524301));
#40593=CARTESIAN_POINT('Ctrl Pts',(-0.00746697525423609,0.136621099781669,
-0.00815073868596875));
#40594=CARTESIAN_POINT('Ctrl Pts',(-0.120752812127179,0.0402994834132936,
-0.743149261314032));
#40595=CARTESIAN_POINT('Ctrl Pts',(-0.134050740763084,0.000453754827045585,
-0.74052338264757));
#40596=CARTESIAN_POINT('Ctrl Pts',(-0.117932690361245,-0.0927509627189708,
-0.735271625314648));
#40597=CARTESIAN_POINT('Ctrl Pts',(0.0130803802391836,-0.149601064531786,
-0.727393989315262));
#40598=CARTESIAN_POINT('Ctrl Pts',(0.132115840991593,-0.0710983567296433,
-0.719516353315881));
#40599=CARTESIAN_POINT('Ctrl Pts',(0.132001267716162,0.0714011740242192,
-0.711638717316495));
#40600=CARTESIAN_POINT('Ctrl Pts',(0.0127100429158007,0.149549206078874,
-0.703761081317112));
#40601=CARTESIAN_POINT('Ctrl Pts',(-0.118028786652939,0.092681307951219,
-0.695883445317726));
#40602=CARTESIAN_POINT('Ctrl Pts',(-0.142257935636087,-0.0478077362715918,
-0.688005809318345));
#40603=CARTESIAN_POINT('Ctrl Pts',(-0.0380916871235754,-0.145162796290568,
-0.680128173318959));
#40604=CARTESIAN_POINT('Ctrl Pts',(0.100449223876869,-0.11150046790381,
-0.672250537319576));
#40605=CARTESIAN_POINT('Ctrl Pts',(0.148335679077349,0.0227883715493975,
-0.664372901320192));
#40606=CARTESIAN_POINT('Ctrl Pts',(0.0623470351390212,0.136512398638226,
-0.656495265320809));
#40607=CARTESIAN_POINT('Ctrl Pts',(-0.0799098209066646,0.127031885279177,
-0.648617629321423));
#40608=CARTESIAN_POINT('Ctrl Pts',(-0.15004767316034,0.00290458103313051,
-0.64073999332204));
#40609=CARTESIAN_POINT('Ctrl Pts',(-0.0847661410457665,-0.123844405107302,
-0.632862357322656));
#40610=CARTESIAN_POINT('Ctrl Pts',(0.0570174516879159,-0.138822662712705,
-0.624984721323272));
#40611=CARTESIAN_POINT('Ctrl Pts',(0.147342367800587,-0.0285124122656285,
-0.617107085323888));
#40612=CARTESIAN_POINT('Ctrl Pts',(0.104689576781408,0.107530562425632,
-0.609229449324504));
#40613=CARTESIAN_POINT('Ctrl Pts',(-0.0324463995342276,0.146526307606242,
-0.60135181332512));
#40614=CARTESIAN_POINT('Ctrl Pts',(-0.140299241507412,0.0532808776708985,
-0.593474177325736));
#40615=CARTESIAN_POINT('Ctrl Pts',(-0.121530872271684,-0.0880509841918077,
-0.585596541326352));
#40616=CARTESIAN_POINT('Ctrl Pts',(0.00692009760954291,-0.149916112522029,
-0.577718905326969));
#40617=CARTESIAN_POINT('Ctrl Pts',(0.129125623836115,-0.076480729741865,
-0.569841269327583));
#40618=CARTESIAN_POINT('Ctrl Pts',(0.134794222307729,0.0659791354674974,
-0.561963633328201));
#40619=CARTESIAN_POINT('Ctrl Pts',(0.0188099373772952,0.148892293024944,
-0.554085997328816));
#40620=CARTESIAN_POINT('Ctrl Pts',(-0.114150469373828,0.097428943530908,
-0.546208361329432));
#40621=CARTESIAN_POINT('Ctrl Pts',(-0.144089147618066,-0.0419648212500574,
-0.538330725330049));
#40622=CARTESIAN_POINT('Ctrl Pts',(-0.043986196463099,-0.143484992955057,
-0.530453089330663));
#40623=CARTESIAN_POINT('Ctrl Pts',(0.0958146553151759,-0.115508789767149,
-0.52257545333128));
#40624=CARTESIAN_POINT('Ctrl Pts',(0.149142000185364,0.0167150371031994,
-0.514697817331896));
#40625=CARTESIAN_POINT('Ctrl Pts',(0.0678674750275233,0.1338534068228,-0.506820181332512));
#40626=CARTESIAN_POINT('Ctrl Pts',(-0.0746579991730203,0.130187986560573,
-0.498942545333128));
#40627=CARTESIAN_POINT('Ctrl Pts',(-0.149804020977185,0.00902684795295702,
-0.491064909333744));
#40628=CARTESIAN_POINT('Ctrl Pts',(-0.089750693592024,-0.120281094460784,
-0.48318727333436));
#40629=CARTESIAN_POINT('Ctrl Pts',(0.0513033658422252,-0.14103436935109,
-0.475309637334976));
#40630=CARTESIAN_POINT('Ctrl Pts',(0.14605571970202,-0.0345029770784666,
-0.467432001335592));
#40631=CARTESIAN_POINT('Ctrl Pts',(0.108991596805259,0.103167633058055,
-0.459554365336209));
#40632=CARTESIAN_POINT('Ctrl Pts',(-0.0264383300207842,0.147728613987548,
-0.451676729336824));
#40633=CARTESIAN_POINT('Ctrl Pts',(-0.138007448644426,0.0589633174407497,
-0.443799093337441));
#40634=CARTESIAN_POINT('Ctrl Pts',(-0.125023720699679,-0.0830168533935917,
-0.435921457338056));
#40635=CARTESIAN_POINT('Ctrl Pts',(0.000794933581836814,-0.150073637810129,
-0.428043821338672));
#40636=CARTESIAN_POINT('Ctrl Pts',(0.125896153830453,-0.0816877416486904,
-0.420166185339288));
#40637=CARTESIAN_POINT('Ctrl Pts',(0.137375069735211,0.0604220067542489,
-0.412288549339905));
#40638=CARTESIAN_POINT('Ctrl Pts',(0.0248718661882977,0.148000401882144,
-0.40441091334052));
#40639=CARTESIAN_POINT('Ctrl Pts',(-0.110078399192231,0.102007228745028,
-0.396533277341137));
#40640=CARTESIAN_POINT('Ctrl Pts',(-0.145682012636526,-0.0360482992544141,
-0.388655641341752));
#40641=CARTESIAN_POINT('Ctrl Pts',(-0.0498064229948769,-0.141569943538238,
-0.380778005342368));
#40642=CARTESIAN_POINT('Ctrl Pts',(0.0910198691076597,-0.11932356059299,
-0.372900369342984));
#40643=CARTESIAN_POINT('Ctrl Pts',(0.149699987920293,0.0106133077609567,
-0.365022733343601));
#40644=CARTESIAN_POINT('Ctrl Pts',(0.0732746482241745,0.130971579407855,
-0.357145097344216));
#40645=CARTESIAN_POINT('Ctrl Pts',(-0.0692816583673163,0.133126933784411,
-0.349267461344833));
#40646=CARTESIAN_POINT('Ctrl Pts',(-0.149310703934934,0.0151341460089211,
-0.341389825345448));
#40647=CARTESIAN_POINT('Ctrl Pts',(-0.0945856229615745,-0.116517331817784,
-0.333512189346065));
#40648=CARTESIAN_POINT('Ctrl Pts',(0.0455037532003936,-0.1430109685641,
-0.32563455334668));
#40649=CARTESIAN_POINT('Ctrl Pts',(0.144525621439241,-0.0404360412573544,
-0.317756917347297));
#40650=CARTESIAN_POINT('Ctrl Pts',(0.113111939067299,0.0986327426638849,
-0.309879281347913));
#40651=CARTESIAN_POINT('Ctrl Pts',(-0.020386189688409,0.148684672898556,
-0.302001645348529));
#40652=CARTESIAN_POINT('Ctrl Pts',(-0.135485616190635,0.0645474747020636,
-0.294124009349145));
#40653=CARTESIAN_POINT('Ctrl Pts',(-0.12830817045604,-0.0778443451972303,
-0.286246373349761));
#40654=CARTESIAN_POINT('Ctrl Pts',(-0.00533155572552474,-0.149981009459524,
-0.278368737350377));
#40655=CARTESIAN_POINT('Ctrl Pts',(0.122456831476679,-0.0867585909849453,
-0.270491101350993));
#40656=CARTESIAN_POINT('Ctrl Pts',(0.139726930774663,0.0547641625629956,
-0.262613465351609));
#40657=CARTESIAN_POINT('Ctrl Pts',(0.0308923368759293,0.146861813305034,
-0.254735829352225));
#40658=CARTESIAN_POINT('Ctrl Pts',(-0.105822842694085,0.106415481248536,
-0.246858193352841));
#40659=CARTESIAN_POINT('Ctrl Pts',(-0.147032044729728,-0.0300716894649577,
-0.238980557353457));
#40660=CARTESIAN_POINT('Ctrl Pts',(-0.0555436287225143,-0.139418915477736,
-0.231102921354073));
#40661=CARTESIAN_POINT('Ctrl Pts',(0.0860733646562128,-0.122939434614756,
-0.223225285354689));
#40662=CARTESIAN_POINT('Ctrl Pts',(0.15000844529019,0.0044938874288485,
-0.215347649355305));
#40663=CARTESIAN_POINT('Ctrl Pts',(0.0785596821549869,0.127871439436481,
-0.207470013355921));
#40664=CARTESIAN_POINT('Ctrl Pts',(-0.0637898341025878,0.135843975799365,
-0.199592377356537));
#40665=CARTESIAN_POINT('Ctrl Pts',(-0.148568505367037,0.0212162173671073,
-0.191714741357153));
#40666=CARTESIAN_POINT('Ctrl Pts',(-0.0992628905392872,-0.112559349884269,
-0.183837105357769));
#40667=CARTESIAN_POINT('Ctrl Pts',(0.039628291937076,-0.144749187324364,
-0.175959469358385));
#40668=CARTESIAN_POINT('Ctrl Pts',(0.142754617434278,-0.0463017034874096,
-0.168081833359001));
#40669=CARTESIAN_POINT('Ctrl Pts',(0.117043739202515,0.0939334437022093,
-0.160204197359617));
#40670=CARTESIAN_POINT('Ctrl Pts',(-0.0143000696108409,0.149392895085614,
-0.152326561360233));
#40671=CARTESIAN_POINT('Ctrl Pts',(-0.132737944273974,0.0700240373969747,
-0.144448925360849));
#40672=CARTESIAN_POINT('Ctrl Pts',(-0.13137875218778,-0.0725420761753132,
-0.136571289361465));
#40673=CARTESIAN_POINT('Ctrl Pts',(-0.0114491485981074,-0.149638390791491,
-0.128693653362081));
#40674=CARTESIAN_POINT('Ctrl Pts',(0.11881337164443,-0.0916848089822516,
-0.120816017362697));
#40675=CARTESIAN_POINT('Ctrl Pts',(0.14184591927742,0.0490150030961542,
-0.112938381363313));
#40676=CARTESIAN_POINT('Ctrl Pts',(0.0368612494010009,0.145478483303915,
-0.105060745363929));
#40677=CARTESIAN_POINT('Ctrl Pts',(-0.101390770448281,0.110646242696357,
-0.0971831093645454));
#40678=CARTESIAN_POINT('Ctrl Pts',(-0.148137227044466,-0.0240447444603757,
-0.0893054733651613));
#40679=CARTESIAN_POINT('Ctrl Pts',(-0.061187806865589,-0.137035892583625,
-0.0814278373657773));
#40680=CARTESIAN_POINT('Ctrl Pts',(0.0809825442572348,-0.126349627802613,
-0.0735502013663932));
#40681=CARTESIAN_POINT('Ctrl Pts',(0.150068459677146,-0.00163446166856293,
-0.0656725653670095));
#40682=CARTESIAN_POINT('Ctrl Pts',(0.0837107242829451,0.124560886874171,
-0.0577949293676252));
#40683=CARTESIAN_POINT('Ctrl Pts',(-0.0581858982491374,0.138329391552391,
-0.0499172933682416));
#40684=CARTESIAN_POINT('Ctrl Pts',(-0.147589650954845,0.0272727915837357,
-0.0420396573688573));
#40685=CARTESIAN_POINT('Ctrl Pts',(-0.103753806033519,-0.108432513870469,
-0.0341620213694735));
#40686=CARTESIAN_POINT('Ctrl Pts',(0.0336469492657874,-0.14621030940285,
-0.0262843853700894));
#40687=CARTESIAN_POINT('Ctrl Pts',(0.140822410570581,-0.0521595967903893,
-0.0184067493707056));
#40688=CARTESIAN_POINT('Ctrl Pts',(0.120625429258503,0.0892208852082231,
-0.0105291133713215));
#40689=CARTESIAN_POINT('Ctrl Pts',(0.0349963898237052,0.129402703572537,
-0.00527735603839891));
#40690=CARTESIAN_POINT('Ctrl Pts',(-0.00694716572164709,0.127110294187512,
-0.00265147737193757));
#40691=CARTESIAN_POINT('Ctrl Pts',(-0.111717694016328,0.037284145003932,
-0.73765));
#40692=CARTESIAN_POINT('Ctrl Pts',(-0.124020628384699,0.000419803415201668,
-0.735024121333539));
#40693=CARTESIAN_POINT('Ctrl Pts',(-0.109108582932408,-0.0858110340473438,
-0.729772364000617));
#40694=CARTESIAN_POINT('Ctrl Pts',(0.0121016636501963,-0.138407426356883,
-0.721894728001232));
#40695=CARTESIAN_POINT('Ctrl Pts',(0.122230504106716,-0.0657785464558806,
-0.714017092001848));
#40696=CARTESIAN_POINT('Ctrl Pts',(0.122124503576362,0.0660587059756678,
-0.706139456002464));
#40697=CARTESIAN_POINT('Ctrl Pts',(0.0117590361697431,0.138359448122069,
-0.69826182000308));
#40698=CARTESIAN_POINT('Ctrl Pts',(-0.109197488987038,0.0857465910758423,
-0.690384184003696));
#40699=CARTESIAN_POINT('Ctrl Pts',(-0.131613734246191,-0.0442306059653326,
-0.682506548004313));
#40700=CARTESIAN_POINT('Ctrl Pts',(-0.0352415432127178,-0.134301243779432,
-0.674628912004927));
#40701=CARTESIAN_POINT('Ctrl Pts',(0.0929332862694289,-0.103157640277856,
-0.666751276005546));
#40702=CARTESIAN_POINT('Ctrl Pts',(0.137236721157382,0.0210832714786364,
-0.65887364000616));
#40703=CARTESIAN_POINT('Ctrl Pts',(0.0576820272073694,0.126298097011918,
-0.650996004006777));
#40704=CARTESIAN_POINT('Ctrl Pts',(-0.0739307082268856,0.11752694649454,
-0.643118368007392));
#40705=CARTESIAN_POINT('Ctrl Pts',(-0.138820618275404,0.0026872508340677,
-0.635240732008009));
#40706=CARTESIAN_POINT('Ctrl Pts',(-0.0784236626996469,-0.114577963955322,
-0.627363096008624));
#40707=CARTESIAN_POINT('Ctrl Pts',(0.0527512205227371,-0.128435499614995,
-0.619485460009241));
#40708=CARTESIAN_POINT('Ctrl Pts',(0.136317732660755,-0.0263790208529794,
-0.611607824009857));
#40709=CARTESIAN_POINT('Ctrl Pts',(0.0968563621793423,0.099484776038326,
-0.603730188010473));
#40710=CARTESIAN_POINT('Ctrl Pts',(-0.030018654400187,0.135562732744109,
-0.595852552011088));
#40711=CARTESIAN_POINT('Ctrl Pts',(-0.129801595982211,0.0492942291256084,
-0.587974916011705));
#40712=CARTESIAN_POINT('Ctrl Pts',(-0.112437537170444,-0.0814627231986667,
-0.580097280012321));
#40713=CARTESIAN_POINT('Ctrl Pts',(0.00640231340113165,-0.138698901431908,
-0.572219644012936));
#40714=CARTESIAN_POINT('Ctrl Pts',(0.119464024723476,-0.0707581928149885,
-0.564342008013553));
#40715=CARTESIAN_POINT('Ctrl Pts',(0.124708480222252,0.0610423619770983,
-0.556464372014168));
#40716=CARTESIAN_POINT('Ctrl Pts',(0.0174025166897942,0.137751687439221,
-0.548586736014785));
#40717=CARTESIAN_POINT('Ctrl Pts',(-0.10560936001966,0.0901389931213871,
-0.540709100015401));
#40718=CARTESIAN_POINT('Ctrl Pts',(-0.133307928992284,-0.0388248768478054,
-0.532831464016017));
#40719=CARTESIAN_POINT('Ctrl Pts',(-0.0406950061935692,-0.13274897914597,
-0.524953828016632));
#40720=CARTESIAN_POINT('Ctrl Pts',(0.0886454911998817,-0.106866046463675,
-0.51707619201725));
#40721=CARTESIAN_POINT('Ctrl Pts',(0.137982710697811,0.0154643636671598,
-0.509198556017864));
#40722=CARTESIAN_POINT('Ctrl Pts',(0.0627894098300584,0.12383805961159,
-0.501320920018481));
#40723=CARTESIAN_POINT('Ctrl Pts',(-0.0690718448751183,0.120446898013915,
-0.493443284019097));
#40724=CARTESIAN_POINT('Ctrl Pts',(-0.13859519694099,0.00835142983235973,
-0.485565648019713));
#40725=CARTESIAN_POINT('Ctrl Pts',(-0.0830352548138296,-0.111281271799835,
-0.477688012020329));
#40726=CARTESIAN_POINT('Ctrl Pts',(0.0474646811631436,-0.130481719169871,
-0.469810376020945));
#40727=CARTESIAN_POINT('Ctrl Pts',(0.135127355757309,-0.0319213521242443,
-0.461932740021561));
#40728=CARTESIAN_POINT('Ctrl Pts',(0.10083649107415,0.0954482952349766,
-0.454055104022177));
#40729=CARTESIAN_POINT('Ctrl Pts',(-0.024460128186944,0.136675078651873,
-0.446177468022793));
#40730=CARTESIAN_POINT('Ctrl Pts',(-0.127681282514511,0.0545514902716746,
-0.438299832023409));
#40731=CARTESIAN_POINT('Ctrl Pts',(-0.115669039319754,-0.0768052624385732,
-0.430422196024025));
#40732=CARTESIAN_POINT('Ctrl Pts',(0.000735454065993374,-0.138844640165656,
-0.42254456002464));
#40733=CARTESIAN_POINT('Ctrl Pts',(0.116476194166392,-0.0755755991569081,
-0.414666924025258));
#40734=CARTESIAN_POINT('Ctrl Pts',(0.127096220251881,0.0559010357068483,
-0.406789288025873));
#40735=CARTESIAN_POINT('Ctrl Pts',(0.0230108722727937,0.136926530492298,
-0.39891165202649));
#40736=CARTESIAN_POINT('Ctrl Pts',(-0.101841975372074,0.0943747161464696,
-0.391034016027105));
#40737=CARTESIAN_POINT('Ctrl Pts',(-0.13478161066981,-0.0333510482693538,
-0.383156380027722));
#40738=CARTESIAN_POINT('Ctrl Pts',(-0.0460797444479301,-0.130977219954565,
-0.375278744028337));
#40739=CARTESIAN_POINT('Ctrl Pts',(0.0842094664898252,-0.110395383730082,
-0.367401108028953));
#40740=CARTESIAN_POINT('Ctrl Pts',(0.138498947975746,0.0098191855581053,
-0.359523472029569));
#40741=CARTESIAN_POINT('Ctrl Pts',(0.0677920007431425,0.121171859895995,
-0.351645836030185));
#40742=CARTESIAN_POINT('Ctrl Pts',(-0.0640977793732191,0.123165943648539,
-0.343768200030801));
#40743=CARTESIAN_POINT('Ctrl Pts',(-0.138138791484186,0.0140017599858645,
-0.335890564031418));
#40744=CARTESIAN_POINT('Ctrl Pts',(-0.0875084190439853,-0.107799126118143,
-0.328012928032034));
#40745=CARTESIAN_POINT('Ctrl Pts',(0.0420990144004436,-0.132310422801546,
-0.320135292032649));
#40746=CARTESIAN_POINT('Ctrl Pts',(0.133711744422676,-0.0374104851459921,
-0.312257656033266));
#40747=CARTESIAN_POINT('Ctrl Pts',(0.104648535928131,0.0912527200882886,
-0.304380020033881));
#40748=CARTESIAN_POINT('Ctrl Pts',(-0.0188608286767674,0.137559602125903,
-0.296502384034497));
#40749=CARTESIAN_POINT('Ctrl Pts',(-0.125348141766317,0.0597178227261228,
-0.288624748035114));
#40750=CARTESIAN_POINT('Ctrl Pts',(-0.118707735863786,-0.0720197781272891,
-0.280747112035729));
#40751=CARTESIAN_POINT('Ctrl Pts',(-0.00493263138706642,-0.138758942569485,
-0.272869476036346));
#40752=CARTESIAN_POINT('Ctrl Pts',(0.113294213096355,-0.0802670310546098,
-0.264991840036961));
#40753=CARTESIAN_POINT('Ctrl Pts',(0.129272107399731,0.0506665298182005,
-0.257114204037578));
#40754=CARTESIAN_POINT('Ctrl Pts',(0.0285808717640413,0.1358731348154,-0.249236568038194));
#40755=CARTESIAN_POINT('Ctrl Pts',(-0.0979048334508719,0.0984531288613211,
-0.24135893203881));
#40756=CARTESIAN_POINT('Ctrl Pts',(-0.136030628971278,-0.0278216278612372,
-0.233481296039426));
#40757=CARTESIAN_POINT('Ctrl Pts',(-0.0513876737847133,-0.128987138809037,
-0.225603660040042));
#40758=CARTESIAN_POINT('Ctrl Pts',(0.0796330755882605,-0.113740706298137,
-0.217726024040658));
#40759=CARTESIAN_POINT('Ctrl Pts',(0.138784325562075,0.004157640156581,
-0.209848388041274));
#40760=CARTESIAN_POINT('Ctrl Pts',(0.0726815912474743,0.118303682479431,
-0.20197075204189));
#40761=CARTESIAN_POINT('Ctrl Pts',(-0.0590168712602702,0.125679687743678,
-0.194093116042506));
#40762=CARTESIAN_POINT('Ctrl Pts',(-0.137452126626887,0.0196287509851605,
-0.186215480043122));
#40763=CARTESIAN_POINT('Ctrl Pts',(-0.0918357182503099,-0.104137293264885,
-0.178337844043738));
#40764=CARTESIAN_POINT('Ctrl Pts',(0.0366631742567891,-0.133918582381201,
-0.170460208044354));
#40765=CARTESIAN_POINT('Ctrl Pts',(0.132073252696953,-0.042837259451921,
-0.16258257204497));
#40766=CARTESIAN_POINT('Ctrl Pts',(0.108286145990386,0.0869050379577989,
-0.154704936045586));
#40767=CARTESIAN_POINT('Ctrl Pts',(-0.0132300918964409,0.138214832825673,
-0.146827300046202));
#40768=CARTESIAN_POINT('Ctrl Pts',(-0.12280605959833,0.0647846111895411,
-0.138949664046818));
#40769=CARTESIAN_POINT('Ctrl Pts',(-0.121548566684335,-0.0671142421174204,
-0.131072028047434));
#40770=CARTESIAN_POINT('Ctrl Pts',(-0.01059248606553,-0.138441959744445,
-0.12319439204805));
#40771=CARTESIAN_POINT('Ctrl Pts',(0.10992336877787,-0.0848246534005071,
-0.115316756048666));
#40772=CARTESIAN_POINT('Ctrl Pts',(0.131232546291422,0.045347541159856,
-0.107439120049282));
#40773=CARTESIAN_POINT('Ctrl Pts',(0.034103170842127,0.134593310063775,
-0.099561484049898));
#40774=CARTESIAN_POINT('Ctrl Pts',(-0.0938043832643078,0.102367330978503,
-0.0916838480505142));
#40775=CARTESIAN_POINT('Ctrl Pts',(-0.137053117950997,-0.022245638482489,
-0.0838062120511301));
#40776=CARTESIAN_POINT('Ctrl Pts',(-0.0566095361633514,-0.126782421437836,
-0.0759285760517461));
#40777=CARTESIAN_POINT('Ctrl Pts',(0.0749231669276979,-0.116895737741183,
-0.0680509400523622));
#40778=CARTESIAN_POINT('Ctrl Pts',(0.138839849477423,-0.00151216593098895,
-0.0601733040529782));
#40779=CARTESIAN_POINT('Ctrl Pts',(0.0774472156514042,0.115240836226281,
-0.0522956680535942));
#40780=CARTESIAN_POINT('Ctrl Pts',(-0.0538322401122725,0.127979136607092,
-0.0444180320542103));
#40781=CARTESIAN_POINT('Ctrl Pts',(-0.136546513285208,0.0252321526219511,
-0.0365403960548262));
#40782=CARTESIAN_POINT('Ctrl Pts',(-0.0959906088420872,-0.10031924054277,
-0.0286627600554423));
#40783=CARTESIAN_POINT('Ctrl Pts',(0.0311293750964514,-0.135270378553972,
-0.0207851240560583));
#40784=CARTESIAN_POINT('Ctrl Pts',(0.130285619834645,-0.0482568461271642,
-0.0129074880566744));
#40785=CARTESIAN_POINT('Ctrl Pts',(0.111599842348155,0.0825450884163283,
-0.0050298520572903));
#40786=CARTESIAN_POINT('Ctrl Pts',(0.0323778461232267,0.119720372452911,
0.000221905275632274));
#40787=CARTESIAN_POINT('Ctrl Pts',(-0.00642735618905809,0.117599488593356,
0.00284778394209362));
#40788=CARTESIAN_POINT('Ctrl Pts',(-0.00798678478682509,0.146131905375825,
-0.0136499999999999));
#40789=CARTESIAN_POINT('Ctrl Pts',(0.0402334772246618,0.148767365811789,
-0.0162758786664613));
#40790=CARTESIAN_POINT('Ctrl Pts',(0.0894550401519313,0.125669922301901,
-0.0189017573329226));
#40791=CARTESIAN_POINT('Ctrl Pts',(0.117935719776108,0.087031604395481,
-0.0215276359993839));
#40792=CARTESIAN_POINT('Ctrl Pts',(0.146416399400285,0.0483932864890619,
-0.0241535146658452));
#40793=CARTESIAN_POINT('Ctrl Pts',(0.154156195721369,-0.00578590581389135,
-0.0267793933323067));
#40794=CARTESIAN_POINT('Ctrl Pts',(0.137490444808912,-0.0508963474626602,
-0.029405271998768));
#40795=CARTESIAN_POINT('Ctrl Pts',(0.120824693896455,-0.0960067891114296,
-0.0320311506652293));
#40796=CARTESIAN_POINT('Ctrl Pts',(0.0797533957504597,-0.132048480106016,
-0.0346570293316905));
#40797=CARTESIAN_POINT('Ctrl Pts',(0.0328906970073198,-0.142830807174188,
-0.0372829079981518));
#40798=CARTESIAN_POINT('Ctrl Pts',(-0.0139720017358201,-0.15361313424236,
-0.0399087866646132));
#40799=CARTESIAN_POINT('Ctrl Pts',(-0.0666261010761026,-0.139136097384114,
-0.0425346653310745));
#40800=CARTESIAN_POINT('Ctrl Pts',(-0.101352438392533,-0.105895390616129,
-0.0451605439975358));
#40801=CARTESIAN_POINT('Ctrl Pts',(-0.129670617078281,-0.0787886944702327,
-0.0473018611369268));
#40802=CARTESIAN_POINT('Ctrl Pts',(-0.146067080217357,-0.0392044155129423,
-0.0494431782763179));
#40803=CARTESIAN_POINT('Ctrl Pts',(-0.146419470807316,0.000121292426834327,
-0.0515844954157089));
#40804=CARTESIAN_POINT('Origin',(0.277715786349443,-0.0489687861020744,
0.04));
#40805=CARTESIAN_POINT('',(0.271097754137541,-0.0461628389679574,0.04));
#40806=CARTESIAN_POINT('',(0.27053717987482,-0.0493420135926708,0.04));
#40807=CARTESIAN_POINT('Origin',(0.,0.,0.04));
#40808=CARTESIAN_POINT('',(0.264913285560284,-0.0467113597924043,0.04));
#40809=CARTESIAN_POINT('',(0.29173382438227,-0.044332558140659,0.04));
#40810=CARTESIAN_POINT('',(0.264913285560284,-0.0467113597924043,0.04));
#40811=CARTESIAN_POINT('Origin',(0.264913285560284,-0.0467113597924043,
0.04));
#40812=CARTESIAN_POINT('',(0.27053717987482,-0.0493420135926708,0.285));
#40813=CARTESIAN_POINT('',(0.27053717987482,-0.0493420135926708,0.1425));
#40814=CARTESIAN_POINT('',(0.264913285560284,-0.0467113597924043,0.291));
#40815=CARTESIAN_POINT('',(0.264913285560284,-0.0467113597924043,0.04));
#40816=CARTESIAN_POINT('Ctrl Pts',(0.27053717987482,-0.0493420135926707,
0.285));
#40817=CARTESIAN_POINT('Ctrl Pts',(0.267694218594527,-0.048012179410566,
0.288035430631103));
#40818=CARTESIAN_POINT('Ctrl Pts',(0.264913285560284,-0.0467113597924043,
0.291));
#40819=CARTESIAN_POINT('Origin',(0.29173382438227,-0.044332558140659,0.04));
#40820=CARTESIAN_POINT('',(0.271097754137541,-0.0461628389679574,0.285));
#40821=CARTESIAN_POINT('',(0.271097754137541,-0.0461628389679574,0.1425));
#40822=CARTESIAN_POINT('Ctrl Pts',(0.264913285560284,-0.0467113597924043,
0.291));
#40823=CARTESIAN_POINT('Ctrl Pts',(0.267971414323715,-0.0464401243111941,
0.288035430631094));
#40824=CARTESIAN_POINT('Ctrl Pts',(0.271097754137541,-0.0461628389679575,
0.285));
#40825=CARTESIAN_POINT('Origin',(0.264993319061626,-0.0964496804178388,
0.04));
#40826=CARTESIAN_POINT('',(0.25896307723613,-0.0925371526922802,0.04));
#40827=CARTESIAN_POINT('',(0.257858961475997,-0.0955706858117092,0.04));
#40828=CARTESIAN_POINT('Origin',(0.,0.,0.04));
#40829=CARTESIAN_POINT('',(0.252777314991409,-0.0920034185546051,0.04));
#40830=CARTESIAN_POINT('',(0.279603464135123,-0.0943180939355711,0.04));
#40831=CARTESIAN_POINT('',(0.252777314991409,-0.0920034185546051,0.04));
#40832=CARTESIAN_POINT('Origin',(0.252777314991409,-0.0920034185546051,
0.04));
#40833=CARTESIAN_POINT('',(0.257858961475997,-0.0955706858117092,0.285));
#40834=CARTESIAN_POINT('',(0.257858961475997,-0.0955706858117092,0.1425));
#40835=CARTESIAN_POINT('',(0.252777314991409,-0.0920034185546051,0.291));
#40836=CARTESIAN_POINT('',(0.252777314991409,-0.0920034185546051,0.04));
#40837=CARTESIAN_POINT('Ctrl Pts',(0.257858961475997,-0.0955706858117092,
0.285));
#40838=CARTESIAN_POINT('Ctrl Pts',(0.255290114447966,-0.0937673797534469,
0.28803543063111));
#40839=CARTESIAN_POINT('Ctrl Pts',(0.252777314991409,-0.0920034185546051,
0.291));
#40840=CARTESIAN_POINT('Origin',(0.279603464135123,-0.0943180939355711,
0.04));
#40841=CARTESIAN_POINT('',(0.25896307723613,-0.0925371526922802,0.285));
#40842=CARTESIAN_POINT('',(0.25896307723613,-0.0925371526922802,0.1425));
#40843=CARTESIAN_POINT('Ctrl Pts',(0.252777314991409,-0.0920034185546051,
0.291));
#40844=CARTESIAN_POINT('Ctrl Pts',(0.255836083454352,-0.0922673422366557,
0.288035430631118));
#40845=CARTESIAN_POINT('Ctrl Pts',(0.25896307723613,-0.0925371526922802,
0.285));
#40846=CARTESIAN_POINT('Origin',(0.244219163867212,-0.141,0.04));
#40847=CARTESIAN_POINT('',(0.238959938274539,-0.136099771858106,0.04));
#40848=CARTESIAN_POINT('',(0.237345829015656,-0.138895491103459,0.04));
#40849=CARTESIAN_POINT('Origin',(0.,0.,0.04));
#40850=CARTESIAN_POINT('',(0.232960833618014,-0.1345,0.04));
#40851=CARTESIAN_POINT('',(0.258977494116409,-0.141437822173509,0.04));
#40852=CARTESIAN_POINT('',(0.232960833618014,-0.1345,0.04));
#40853=CARTESIAN_POINT('Origin',(0.232960833618014,-0.1345,0.04));
#40854=CARTESIAN_POINT('',(0.237345829015656,-0.138895491103459,0.285));
#40855=CARTESIAN_POINT('',(0.237345829015656,-0.138895491103459,0.1425));
#40856=CARTESIAN_POINT('',(0.232960833618014,-0.1345,0.291));
#40857=CARTESIAN_POINT('',(0.232960833618014,-0.1345,0.04));
#40858=CARTESIAN_POINT('Ctrl Pts',(0.237345829015656,-0.138895491103459,
0.285));
#40859=CARTESIAN_POINT('Ctrl Pts',(0.235129149356958,-0.136673505711122,
0.288035430631088));
#40860=CARTESIAN_POINT('Ctrl Pts',(0.232960833618014,-0.1345,0.291));
#40861=CARTESIAN_POINT('Origin',(0.258977494116409,-0.141437822173509,0.04));
#40862=CARTESIAN_POINT('',(0.238959938274539,-0.136099771858106,0.285));
#40863=CARTESIAN_POINT('',(0.238959938274539,-0.136099771858106,0.1425));
#40864=CARTESIAN_POINT('Ctrl Pts',(0.232960833618014,-0.1345,0.291));
#40865=CARTESIAN_POINT('Ctrl Pts',(0.235927302648582,-0.135291063657789,
0.288035430631094));
#40866=CARTESIAN_POINT('Ctrl Pts',(0.238959938274539,-0.136099771858106,
0.285));
#40867=CARTESIAN_POINT('Origin',(0.216024532959552,-0.181266105931604,0.04));
#40868=CARTESIAN_POINT('',(0.211696122508039,-0.175527068325832,0.04));
#40869=CARTESIAN_POINT('',(0.209621063643459,-0.17800002718254,0.04));
#40870=CARTESIAN_POINT('Origin',(0.,0.,0.04));
#40871=CARTESIAN_POINT('',(0.206065955199005,-0.172909867005679,0.04));
#40872=CARTESIAN_POINT('',(0.230482623987904,-0.184260033755696,0.04));
#40873=CARTESIAN_POINT('',(0.206065955199005,-0.172909867005679,0.04));
#40874=CARTESIAN_POINT('Origin',(0.206065955199005,-0.172909867005679,0.04));
#40875=CARTESIAN_POINT('',(0.209621063643459,-0.17800002718254,0.285));
#40876=CARTESIAN_POINT('',(0.209621063643459,-0.17800002718254,0.1425));
#40877=CARTESIAN_POINT('',(0.206065955199005,-0.172909867005679,0.291));
#40878=CARTESIAN_POINT('',(0.206065955199005,-0.172909867005679,0.04));
#40879=CARTESIAN_POINT('Ctrl Pts',(0.209621063643459,-0.17800002718254,
0.285));
#40880=CARTESIAN_POINT('Ctrl Pts',(0.207823904043776,-0.175426876357833,
0.288035430631146));
#40881=CARTESIAN_POINT('Ctrl Pts',(0.206065955199005,-0.172909867005679,
0.291));
#40882=CARTESIAN_POINT('Origin',(0.230482623987904,-0.184260033755696,0.04));
#40883=CARTESIAN_POINT('',(0.211696122508039,-0.175527068325832,0.285));
#40884=CARTESIAN_POINT('',(0.211696122508039,-0.175527068325832,0.1425));
#40885=CARTESIAN_POINT('Ctrl Pts',(0.206065955199005,-0.172909867005679,
0.291));
#40886=CARTESIAN_POINT('Ctrl Pts',(0.208849990136834,-0.174204034570282,
0.288035430631042));
#40887=CARTESIAN_POINT('Ctrl Pts',(0.211696122508039,-0.175527068325832,
0.285));
#40888=CARTESIAN_POINT('Origin',(0.181266105931604,-0.216024532959552,0.04));
#40889=CARTESIAN_POINT('',(0.17800002718254,-0.209621063643459,0.04));
#40890=CARTESIAN_POINT('',(0.175527068325832,-0.211696122508039,0.04));
#40891=CARTESIAN_POINT('Origin',(0.,0.,0.04));
#40892=CARTESIAN_POINT('',(0.172909867005679,-0.206065955199005,0.04));
#40893=CARTESIAN_POINT('',(0.194984655959362,-0.221483597452293,0.04));
#40894=CARTESIAN_POINT('',(0.172909867005679,-0.206065955199005,0.04));
#40895=CARTESIAN_POINT('Origin',(0.172909867005679,-0.206065955199005,0.04));
#40896=CARTESIAN_POINT('',(0.175527068325832,-0.211696122508039,0.285));
#40897=CARTESIAN_POINT('',(0.175527068325832,-0.211696122508039,0.1425));
#40898=CARTESIAN_POINT('',(0.172909867005679,-0.206065955199005,0.291));
#40899=CARTESIAN_POINT('',(0.172909867005679,-0.206065955199005,0.04));
#40900=CARTESIAN_POINT('Ctrl Pts',(0.175527068325832,-0.211696122508039,
0.285));
#40901=CARTESIAN_POINT('Ctrl Pts',(0.174204034570244,-0.208849990136752,
0.288035430631129));
#40902=CARTESIAN_POINT('Ctrl Pts',(0.172909867005679,-0.206065955199005,
0.291));
#40903=CARTESIAN_POINT('Origin',(0.194984655959362,-0.221483597452293,0.04));
#40904=CARTESIAN_POINT('',(0.17800002718254,-0.209621063643459,0.285));
#40905=CARTESIAN_POINT('',(0.17800002718254,-0.209621063643459,0.1425));
#40906=CARTESIAN_POINT('Ctrl Pts',(0.172909867005679,-0.206065955199005,
0.291));
#40907=CARTESIAN_POINT('Ctrl Pts',(0.175426876357872,-0.207823904043804,
0.2880354306311));
#40908=CARTESIAN_POINT('Ctrl Pts',(0.17800002718254,-0.209621063643459,
0.285));
#40909=CARTESIAN_POINT('Origin',(0.141,-0.244219163867212,0.04));
#40910=CARTESIAN_POINT('',(0.138895491103459,-0.237345829015656,0.04));
#40911=CARTESIAN_POINT('',(0.136099771858106,-0.238959938274539,0.04));
#40912=CARTESIAN_POINT('Origin',(0.,0.,0.04));
#40913=CARTESIAN_POINT('',(0.1345,-0.232960833618014,0.04));
#40914=CARTESIAN_POINT('',(0.153562177826491,-0.251977494116409,0.04));
#40915=CARTESIAN_POINT('',(0.1345,-0.232960833618014,0.04));
#40916=CARTESIAN_POINT('Origin',(0.1345,-0.232960833618014,0.04));
#40917=CARTESIAN_POINT('',(0.136099771858106,-0.238959938274539,0.285));
#40918=CARTESIAN_POINT('',(0.136099771858106,-0.238959938274539,0.1425));
#40919=CARTESIAN_POINT('',(0.1345,-0.232960833618014,0.291));
#40920=CARTESIAN_POINT('',(0.1345,-0.232960833618014,0.04));
#40921=CARTESIAN_POINT('Ctrl Pts',(0.136099771858106,-0.238959938274539,
0.285));
#40922=CARTESIAN_POINT('Ctrl Pts',(0.135291063657772,-0.23592730264852,
0.288035430631155));
#40923=CARTESIAN_POINT('Ctrl Pts',(0.1345,-0.232960833618014,0.291));
#40924=CARTESIAN_POINT('Origin',(0.153562177826491,-0.251977494116409,0.04));
#40925=CARTESIAN_POINT('',(0.138895491103459,-0.237345829015656,0.285));
#40926=CARTESIAN_POINT('',(0.138895491103459,-0.237345829015656,0.1425));
#40927=CARTESIAN_POINT('Ctrl Pts',(0.1345,-0.232960833618014,0.291));
#40928=CARTESIAN_POINT('Ctrl Pts',(0.136673505711114,-0.23512914935695,
0.288035430631099));
#40929=CARTESIAN_POINT('Ctrl Pts',(0.138895491103459,-0.237345829015656,
0.285));
#40930=CARTESIAN_POINT('Origin',(0.0964496804178385,-0.264993319061626,
0.04));
#40931=CARTESIAN_POINT('',(0.0955706858117088,-0.257858961475997,0.04));
#40932=CARTESIAN_POINT('',(0.0925371526922799,-0.25896307723613,0.04));
#40933=CARTESIAN_POINT('Origin',(0.,0.,0.04));
#40934=CARTESIAN_POINT('',(0.0920034185546048,-0.252777314991409,0.04));
#40935=CARTESIAN_POINT('',(0.107473790626574,-0.274815182128563,0.04));
#40936=CARTESIAN_POINT('',(0.0920034185546048,-0.252777314991409,0.04));
#40937=CARTESIAN_POINT('Origin',(0.0920034185546048,-0.252777314991409,
0.04));
#40938=CARTESIAN_POINT('',(0.0925371526922799,-0.25896307723613,0.285));
#40939=CARTESIAN_POINT('',(0.0925371526922799,-0.25896307723613,0.1425));
#40940=CARTESIAN_POINT('',(0.0920034185546048,-0.252777314991409,0.291));
#40941=CARTESIAN_POINT('',(0.0920034185546048,-0.252777314991409,0.04));
#40942=CARTESIAN_POINT('Ctrl Pts',(0.0925371526922799,-0.25896307723613,
0.285));
#40943=CARTESIAN_POINT('Ctrl Pts',(0.0922673422366487,-0.255836083454274,
0.288035430631194));
#40944=CARTESIAN_POINT('Ctrl Pts',(0.0920034185546048,-0.252777314991409,
0.291));
#40945=CARTESIAN_POINT('Origin',(0.107473790626574,-0.274815182128563,0.04));
#40946=CARTESIAN_POINT('',(0.0955706858117089,-0.257858961475997,0.285));
#40947=CARTESIAN_POINT('',(0.0955706858117089,-0.257858961475997,0.1425));
#40948=CARTESIAN_POINT('Ctrl Pts',(0.0920034185546048,-0.252777314991409,
0.291));
#40949=CARTESIAN_POINT('Ctrl Pts',(0.0937673797534969,-0.255290114448038,
0.288035430631026));
#40950=CARTESIAN_POINT('Ctrl Pts',(0.0955706858117088,-0.257858961475997,
0.285));
#40951=CARTESIAN_POINT('Origin',(0.0489687861020743,-0.277715786349443,
0.04));
#40952=CARTESIAN_POINT('',(0.0493420135926707,-0.27053717987482,0.04));
#40953=CARTESIAN_POINT('',(0.0461628389679573,-0.271097754137541,0.04));
#40954=CARTESIAN_POINT('Origin',(0.,0.,0.04));
#40955=CARTESIAN_POINT('',(0.0467113597924042,-0.264913285560284,0.04));
#40956=CARTESIAN_POINT('',(0.0581198666828298,-0.289302749894933,0.04));
#40957=CARTESIAN_POINT('',(0.0467113597924042,-0.264913285560284,0.04));
#40958=CARTESIAN_POINT('Origin',(0.0467113597924042,-0.264913285560284,
0.04));
#40959=CARTESIAN_POINT('',(0.0461628389679573,-0.271097754137541,0.285));
#40960=CARTESIAN_POINT('',(0.0461628389679573,-0.271097754137541,0.1425));
#40961=CARTESIAN_POINT('',(0.0467113597924042,-0.264913285560284,0.291));
#40962=CARTESIAN_POINT('',(0.0467113597924042,-0.264913285560284,0.04));
#40963=CARTESIAN_POINT('Ctrl Pts',(0.0461628389679573,-0.271097754137541,
0.285));
#40964=CARTESIAN_POINT('Ctrl Pts',(0.0464401243112015,-0.26797141432363,
0.288035430631177));
#40965=CARTESIAN_POINT('Ctrl Pts',(0.0467113597924042,-0.264913285560284,
0.291));
#40966=CARTESIAN_POINT('Origin',(0.0581198666828298,-0.289302749894933,
0.04));
#40967=CARTESIAN_POINT('',(0.0493420135926707,-0.27053717987482,0.285));
#40968=CARTESIAN_POINT('',(0.0493420135926707,-0.27053717987482,0.1425));
#40969=CARTESIAN_POINT('Ctrl Pts',(0.0467113597924042,-0.264913285560284,
0.291));
#40970=CARTESIAN_POINT('Ctrl Pts',(0.0480121794105309,-0.267694218594452,
0.288035430631183));
#40971=CARTESIAN_POINT('Ctrl Pts',(0.0493420135926707,-0.27053717987482,
0.285));
#40972=CARTESIAN_POINT('Origin',(-4.85722573273506E-17,-0.282,0.04));
#40973=CARTESIAN_POINT('',(0.00161410925888288,-0.274995262961565,0.04));
#40974=CARTESIAN_POINT('',(-0.00161410925888299,-0.274995262961565,0.04));
#40975=CARTESIAN_POINT('Origin',(0.,0.,0.04));
#40976=CARTESIAN_POINT('',(-6.24500451351651E-17,-0.269,0.04));
#40977=CARTESIAN_POINT('',(0.00699999999999995,-0.295,0.04));
#40978=CARTESIAN_POINT('',(-6.24500451351651E-17,-0.269,0.04));
#40979=CARTESIAN_POINT('Origin',(-6.24500451351651E-17,-0.269,0.04));
#40980=CARTESIAN_POINT('',(-0.00161410925888297,-0.274995262961565,0.285));
#40981=CARTESIAN_POINT('',(-0.00161410925888297,-0.274995262961565,0.1425));
#40982=CARTESIAN_POINT('',(-6.2450045135165E-17,-0.269,0.291));
#40983=CARTESIAN_POINT('',(-6.24500451351651E-17,-0.269,0.04));
#40984=CARTESIAN_POINT('Ctrl Pts',(-0.00161410925888296,-0.274995262961565,
0.285));
#40985=CARTESIAN_POINT('Ctrl Pts',(-0.000798153291622722,-0.271964569368884,
0.288035430631116));
#40986=CARTESIAN_POINT('Ctrl Pts',(-6.24500451351651E-17,-0.269,0.291));
#40987=CARTESIAN_POINT('Origin',(0.00699999999999995,-0.295,0.04));
#40988=CARTESIAN_POINT('',(0.00161410925888286,-0.274995262961565,0.285));
#40989=CARTESIAN_POINT('',(0.00161410925888286,-0.274995262961565,0.1425));
#40990=CARTESIAN_POINT('Ctrl Pts',(-6.2450045135165E-17,-0.269,0.291));
#40991=CARTESIAN_POINT('Ctrl Pts',(0.000798153291617013,-0.271964569368863,
0.288035430631137));
#40992=CARTESIAN_POINT('Ctrl Pts',(0.00161410925888284,-0.274995262961565,
0.285));
#40993=CARTESIAN_POINT('Origin',(-0.0489687861020744,-0.277715786349443,
0.04));
#40994=CARTESIAN_POINT('',(-0.0461628389679574,-0.271097754137541,0.04));
#40995=CARTESIAN_POINT('',(-0.0493420135926708,-0.27053717987482,0.04));
#40996=CARTESIAN_POINT('Origin',(0.,0.,0.04));
#40997=CARTESIAN_POINT('',(-0.0467113597924043,-0.264913285560284,0.04));
#40998=CARTESIAN_POINT('',(-0.044332558140659,-0.29173382438227,0.04));
#40999=CARTESIAN_POINT('',(-0.0467113597924043,-0.264913285560284,0.04));
#41000=CARTESIAN_POINT('Origin',(-0.0467113597924043,-0.264913285560284,
0.04));
#41001=CARTESIAN_POINT('',(-0.0493420135926708,-0.27053717987482,0.285));
#41002=CARTESIAN_POINT('',(-0.0493420135926708,-0.27053717987482,0.1425));
#41003=CARTESIAN_POINT('',(-0.0467113597924043,-0.264913285560284,0.291));
#41004=CARTESIAN_POINT('',(-0.0467113597924043,-0.264913285560284,0.04));
#41005=CARTESIAN_POINT('Ctrl Pts',(-0.0493420135926708,-0.27053717987482,
0.285));
#41006=CARTESIAN_POINT('Ctrl Pts',(-0.0480121794105265,-0.267694218594442,
0.288035430631193));
#41007=CARTESIAN_POINT('Ctrl Pts',(-0.0467113597924043,-0.264913285560284,
0.291));
#41008=CARTESIAN_POINT('Origin',(-0.044332558140659,-0.29173382438227,0.04));
#41009=CARTESIAN_POINT('',(-0.0461628389679574,-0.271097754137541,0.285));
#41010=CARTESIAN_POINT('',(-0.0461628389679574,-0.271097754137541,0.1425));
#41011=CARTESIAN_POINT('Ctrl Pts',(-0.0467113597924043,-0.264913285560284,
0.291));
#41012=CARTESIAN_POINT('Ctrl Pts',(-0.046440124311189,-0.267971414323772,
0.288035430631039));
#41013=CARTESIAN_POINT('Ctrl Pts',(-0.0461628389679575,-0.271097754137541,
0.285));
#41014=CARTESIAN_POINT('Origin',(-0.0964496804178388,-0.264993319061626,
0.04));
#41015=CARTESIAN_POINT('',(-0.0925371526922802,-0.25896307723613,0.04));
#41016=CARTESIAN_POINT('',(-0.0955706858117092,-0.257858961475997,0.04));
#41017=CARTESIAN_POINT('Origin',(0.,0.,0.04));
#41018=CARTESIAN_POINT('',(-0.0920034185546051,-0.252777314991409,0.04));
#41019=CARTESIAN_POINT('',(-0.0943180939355711,-0.279603464135123,0.04));
#41020=CARTESIAN_POINT('',(-0.0920034185546051,-0.252777314991409,0.04));
#41021=CARTESIAN_POINT('Origin',(-0.0920034185546051,-0.252777314991409,
0.04));
#41022=CARTESIAN_POINT('',(-0.0955706858117092,-0.257858961475997,0.285));
#41023=CARTESIAN_POINT('',(-0.0955706858117092,-0.257858961475997,0.1425));
#41024=CARTESIAN_POINT('',(-0.0920034185546051,-0.252777314991409,0.291));
#41025=CARTESIAN_POINT('',(-0.0920034185546051,-0.252777314991409,0.04));
#41026=CARTESIAN_POINT('Ctrl Pts',(-0.0955706858117091,-0.257858961475997,
0.285));
#41027=CARTESIAN_POINT('Ctrl Pts',(-0.0937673797534664,-0.255290114447994,
0.288035430631078));
#41028=CARTESIAN_POINT('Ctrl Pts',(-0.0920034185546051,-0.252777314991409,
0.291));
#41029=CARTESIAN_POINT('Origin',(-0.0943180939355711,-0.279603464135123,
0.04));
#41030=CARTESIAN_POINT('',(-0.0925371526922802,-0.25896307723613,0.285));
#41031=CARTESIAN_POINT('',(-0.0925371526922802,-0.25896307723613,0.1425));
#41032=CARTESIAN_POINT('Ctrl Pts',(-0.0920034185546051,-0.252777314991409,
0.291));
#41033=CARTESIAN_POINT('Ctrl Pts',(-0.0922673422366578,-0.255836083454375,
0.288035430631095));
#41034=CARTESIAN_POINT('Ctrl Pts',(-0.0925371526922802,-0.25896307723613,
0.285));
#41035=CARTESIAN_POINT('Origin',(-0.141,-0.244219163867212,0.04));
#41036=CARTESIAN_POINT('',(-0.136099771858106,-0.238959938274539,0.04));
#41037=CARTESIAN_POINT('',(-0.138895491103459,-0.237345829015656,0.04));
#41038=CARTESIAN_POINT('Origin',(0.,0.,0.04));
#41039=CARTESIAN_POINT('',(-0.1345,-0.232960833618014,0.04));
#41040=CARTESIAN_POINT('',(-0.141437822173509,-0.258977494116409,0.04));
#41041=CARTESIAN_POINT('',(-0.1345,-0.232960833618014,0.04));
#41042=CARTESIAN_POINT('Origin',(-0.1345,-0.232960833618014,0.04));
#41043=CARTESIAN_POINT('',(-0.138895491103459,-0.237345829015656,0.285));
#41044=CARTESIAN_POINT('',(-0.138895491103459,-0.237345829015656,0.1425));
#41045=CARTESIAN_POINT('',(-0.1345,-0.232960833618014,0.291));
#41046=CARTESIAN_POINT('',(-0.1345,-0.232960833618014,0.04));
#41047=CARTESIAN_POINT('Ctrl Pts',(-0.138895491103459,-0.237345829015656,
0.285));
#41048=CARTESIAN_POINT('Ctrl Pts',(-0.136673505711122,-0.235129149356958,
0.288035430631088));
#41049=CARTESIAN_POINT('Ctrl Pts',(-0.1345,-0.232960833618014,0.291));
#41050=CARTESIAN_POINT('Origin',(-0.141437822173509,-0.258977494116409,
0.04));
#41051=CARTESIAN_POINT('',(-0.136099771858106,-0.238959938274539,0.285));
#41052=CARTESIAN_POINT('',(-0.136099771858106,-0.238959938274539,0.1425));
#41053=CARTESIAN_POINT('Ctrl Pts',(-0.1345,-0.232960833618014,0.291));
#41054=CARTESIAN_POINT('Ctrl Pts',(-0.135291063657789,-0.235927302648582,
0.288035430631094));
#41055=CARTESIAN_POINT('Ctrl Pts',(-0.136099771858106,-0.238959938274539,
0.285));
#41056=CARTESIAN_POINT('Origin',(-0.181266105931604,-0.216024532959552,
0.04));
#41057=CARTESIAN_POINT('',(-0.175527068325832,-0.211696122508039,0.04));
#41058=CARTESIAN_POINT('',(-0.17800002718254,-0.209621063643459,0.04));
#41059=CARTESIAN_POINT('Origin',(0.,0.,0.04));
#41060=CARTESIAN_POINT('',(-0.172909867005679,-0.206065955199005,0.04));
#41061=CARTESIAN_POINT('',(-0.184260033755696,-0.230482623987904,0.04));
#41062=CARTESIAN_POINT('',(-0.172909867005679,-0.206065955199005,0.04));
#41063=CARTESIAN_POINT('Origin',(-0.172909867005679,-0.206065955199005,
0.04));
#41064=CARTESIAN_POINT('',(-0.17800002718254,-0.209621063643459,0.285));
#41065=CARTESIAN_POINT('',(-0.17800002718254,-0.209621063643459,0.1425));
#41066=CARTESIAN_POINT('',(-0.172909867005679,-0.206065955199005,0.291));
#41067=CARTESIAN_POINT('',(-0.172909867005679,-0.206065955199005,0.04));
#41068=CARTESIAN_POINT('Ctrl Pts',(-0.17800002718254,-0.209621063643459,
0.285));
#41069=CARTESIAN_POINT('Ctrl Pts',(-0.175426876357765,-0.207823904043728,
0.288035430631226));
#41070=CARTESIAN_POINT('Ctrl Pts',(-0.172909867005679,-0.206065955199005,
0.291));
#41071=CARTESIAN_POINT('Origin',(-0.184260033755696,-0.230482623987904,
0.04));
#41072=CARTESIAN_POINT('',(-0.175527068325832,-0.211696122508039,0.285));
#41073=CARTESIAN_POINT('',(-0.175527068325832,-0.211696122508039,0.1425));
#41074=CARTESIAN_POINT('Ctrl Pts',(-0.172909867005679,-0.206065955199005,
0.291));
#41075=CARTESIAN_POINT('Ctrl Pts',(-0.174204034570293,-0.208849990136858,
0.288035430631017));
#41076=CARTESIAN_POINT('Ctrl Pts',(-0.175527068325832,-0.211696122508039,
0.285));
#41077=CARTESIAN_POINT('Origin',(-0.216024532959552,-0.181266105931604,
0.04));
#41078=CARTESIAN_POINT('',(-0.209621063643459,-0.17800002718254,0.04));
#41079=CARTESIAN_POINT('',(-0.211696122508039,-0.175527068325832,0.04));
#41080=CARTESIAN_POINT('Origin',(0.,0.,0.04));
#41081=CARTESIAN_POINT('',(-0.206065955199005,-0.172909867005679,0.04));
#41082=CARTESIAN_POINT('',(-0.221483597452293,-0.194984655959362,0.04));
#41083=CARTESIAN_POINT('',(-0.206065955199005,-0.172909867005679,0.04));
#41084=CARTESIAN_POINT('Origin',(-0.206065955199005,-0.172909867005679,
0.04));
#41085=CARTESIAN_POINT('',(-0.211696122508039,-0.175527068325832,0.285));
#41086=CARTESIAN_POINT('',(-0.211696122508039,-0.175527068325832,0.1425));
#41087=CARTESIAN_POINT('',(-0.206065955199005,-0.172909867005679,0.291));
#41088=CARTESIAN_POINT('',(-0.206065955199005,-0.172909867005679,0.04));
#41089=CARTESIAN_POINT('Ctrl Pts',(-0.211696122508039,-0.175527068325832,
0.285));
#41090=CARTESIAN_POINT('Ctrl Pts',(-0.208849990136656,-0.174204034570199,
0.288035430631232));
#41091=CARTESIAN_POINT('Ctrl Pts',(-0.206065955199005,-0.172909867005679,
0.291));
#41092=CARTESIAN_POINT('Origin',(-0.221483597452293,-0.194984655959362,
0.04));
#41093=CARTESIAN_POINT('',(-0.209621063643459,-0.17800002718254,0.285));
#41094=CARTESIAN_POINT('',(-0.209621063643459,-0.17800002718254,0.1425));
#41095=CARTESIAN_POINT('Ctrl Pts',(-0.206065955199005,-0.172909867005679,
0.291));
#41096=CARTESIAN_POINT('Ctrl Pts',(-0.207823904043843,-0.175426876357928,
0.288035430631034));
#41097=CARTESIAN_POINT('Ctrl Pts',(-0.209621063643459,-0.17800002718254,
0.285));
#41098=CARTESIAN_POINT('Origin',(-0.244219163867212,-0.141,0.04));
#41099=CARTESIAN_POINT('',(-0.237345829015656,-0.138895491103459,0.04));
#41100=CARTESIAN_POINT('',(-0.238959938274539,-0.136099771858106,0.04));
#41101=CARTESIAN_POINT('Origin',(0.,0.,0.04));
#41102=CARTESIAN_POINT('',(-0.232960833618014,-0.1345,0.04));
#41103=CARTESIAN_POINT('',(-0.25197749411641,-0.153562177826491,0.04));
#41104=CARTESIAN_POINT('',(-0.232960833618014,-0.1345,0.04));
#41105=CARTESIAN_POINT('Origin',(-0.232960833618014,-0.1345,0.04));
#41106=CARTESIAN_POINT('',(-0.238959938274539,-0.136099771858106,0.285));
#41107=CARTESIAN_POINT('',(-0.238959938274539,-0.136099771858106,0.1425));
#41108=CARTESIAN_POINT('',(-0.232960833618014,-0.1345,0.291));
#41109=CARTESIAN_POINT('',(-0.232960833618014,-0.1345,0.04));
#41110=CARTESIAN_POINT('Ctrl Pts',(-0.238959938274539,-0.136099771858106,
0.285));
#41111=CARTESIAN_POINT('Ctrl Pts',(-0.23592730264851,-0.135291063657769,
0.288035430631166));
#41112=CARTESIAN_POINT('Ctrl Pts',(-0.232960833618014,-0.1345,0.291));
#41113=CARTESIAN_POINT('Origin',(-0.25197749411641,-0.153562177826491,0.04));
#41114=CARTESIAN_POINT('',(-0.237345829015656,-0.138895491103459,0.285));
#41115=CARTESIAN_POINT('',(-0.237345829015656,-0.138895491103459,0.1425));
#41116=CARTESIAN_POINT('Ctrl Pts',(-0.232960833618014,-0.1345,0.291));
#41117=CARTESIAN_POINT('Ctrl Pts',(-0.235129149356959,-0.136673505711123,
0.288035430631086));
#41118=CARTESIAN_POINT('Ctrl Pts',(-0.237345829015656,-0.138895491103459,
0.285));
#41119=CARTESIAN_POINT('Origin',(-0.264993319061626,-0.0964496804178386,
0.04));
#41120=CARTESIAN_POINT('',(-0.257858961475997,-0.095570685811709,0.04));
#41121=CARTESIAN_POINT('',(-0.25896307723613,-0.09253715269228,0.04));
#41122=CARTESIAN_POINT('Origin',(0.,0.,0.04));
#41123=CARTESIAN_POINT('',(-0.252777314991409,-0.0920034185546049,0.04));
#41124=CARTESIAN_POINT('',(-0.274815182128563,-0.107473790626574,0.04));
#41125=CARTESIAN_POINT('',(-0.252777314991409,-0.0920034185546049,0.04));
#41126=CARTESIAN_POINT('Origin',(-0.252777314991409,-0.0920034185546049,
0.04));
#41127=CARTESIAN_POINT('',(-0.25896307723613,-0.09253715269228,0.285));
#41128=CARTESIAN_POINT('',(-0.25896307723613,-0.09253715269228,0.1425));
#41129=CARTESIAN_POINT('',(-0.252777314991409,-0.0920034185546049,0.291));
#41130=CARTESIAN_POINT('',(-0.252777314991409,-0.0920034185546049,0.04));
#41131=CARTESIAN_POINT('Ctrl Pts',(-0.25896307723613,-0.09253715269228,
0.285));
#41132=CARTESIAN_POINT('Ctrl Pts',(-0.255836083454338,-0.0922673422366543,
0.288035430631132));
#41133=CARTESIAN_POINT('Ctrl Pts',(-0.252777314991409,-0.0920034185546049,
0.291));
#41134=CARTESIAN_POINT('Origin',(-0.274815182128563,-0.107473790626574,
0.04));
#41135=CARTESIAN_POINT('',(-0.257858961475997,-0.095570685811709,0.285));
#41136=CARTESIAN_POINT('',(-0.257858961475997,-0.095570685811709,0.1425));
#41137=CARTESIAN_POINT('Ctrl Pts',(-0.252777314991409,-0.0920034185546049,
0.291));
#41138=CARTESIAN_POINT('Ctrl Pts',(-0.255290114448016,-0.0937673797534821,
0.288035430631051));
#41139=CARTESIAN_POINT('Ctrl Pts',(-0.257858961475997,-0.0955706858117089,
0.285));
#41140=CARTESIAN_POINT('Origin',(-0.277715786349443,-0.0489687861020743,
0.04));
#41141=CARTESIAN_POINT('',(-0.27053717987482,-0.0493420135926707,0.04));
#41142=CARTESIAN_POINT('',(-0.271097754137541,-0.0461628389679573,0.04));
#41143=CARTESIAN_POINT('Origin',(0.,0.,0.04));
#41144=CARTESIAN_POINT('',(-0.264913285560284,-0.0467113597924042,0.04));
#41145=CARTESIAN_POINT('',(-0.289302749894933,-0.0581198666828298,0.04));
#41146=CARTESIAN_POINT('',(-0.264913285560284,-0.0467113597924042,0.04));
#41147=CARTESIAN_POINT('Origin',(-0.264913285560284,-0.0467113597924042,
0.04));
#41148=CARTESIAN_POINT('',(-0.271097754137541,-0.0461628389679573,0.285));
#41149=CARTESIAN_POINT('',(-0.271097754137541,-0.0461628389679573,0.1425));
#41150=CARTESIAN_POINT('',(-0.264913285560284,-0.0467113597924042,0.291));
#41151=CARTESIAN_POINT('',(-0.264913285560284,-0.0467113597924042,0.04));
#41152=CARTESIAN_POINT('Ctrl Pts',(-0.271097754137541,-0.0461628389679573,
0.285));
#41153=CARTESIAN_POINT('Ctrl Pts',(-0.267971414323669,-0.0464401243111981,
0.288035430631139));
#41154=CARTESIAN_POINT('Ctrl Pts',(-0.264913285560284,-0.0467113597924042,
0.291));
#41155=CARTESIAN_POINT('Origin',(-0.289302749894933,-0.0581198666828298,
0.04));
#41156=CARTESIAN_POINT('',(-0.27053717987482,-0.0493420135926707,0.285));
#41157=CARTESIAN_POINT('',(-0.27053717987482,-0.0493420135926707,0.1425));
#41158=CARTESIAN_POINT('Ctrl Pts',(-0.264913285560284,-0.0467113597924042,
0.291));
#41159=CARTESIAN_POINT('Ctrl Pts',(-0.2676942185945,-0.0480121794105537,
0.288035430631131));
#41160=CARTESIAN_POINT('Ctrl Pts',(-0.27053717987482,-0.0493420135926707,
0.285));
#41161=CARTESIAN_POINT('Origin',(-0.282,2.77555756156289E-17,0.04));
#41162=CARTESIAN_POINT('',(-0.274995262961565,-0.0016141092588829,0.04));
#41163=CARTESIAN_POINT('',(-0.275,-3.36777869765522E-17,0.04));
#41164=CARTESIAN_POINT('Origin',(0.,0.,0.04));
#41165=CARTESIAN_POINT('',(-0.269,4.16333634234434E-17,0.04));
#41166=CARTESIAN_POINT('',(-0.295,-0.00699999999999998,0.04));
#41167=CARTESIAN_POINT('',(-0.274995262961565,0.00161410925888296,0.04));
#41168=CARTESIAN_POINT('',(-0.269,4.16333634234434E-17,0.04));
#41169=CARTESIAN_POINT('Origin',(0.,0.,0.04));
#41170=CARTESIAN_POINT('Origin',(-0.269,4.16333634234434E-17,0.04));
#41171=CARTESIAN_POINT('',(-0.274995262961565,0.00161410925888297,0.285));
#41172=CARTESIAN_POINT('',(-0.274995262961565,0.00161410925888297,0.1425));
#41173=CARTESIAN_POINT('',(-0.269,4.16333634234434E-17,0.291));
#41174=CARTESIAN_POINT('',(-0.269,4.16333634234434E-17,0.04));
#41175=CARTESIAN_POINT('Ctrl Pts',(-0.274995262961565,0.00161410925888294,
0.285));
#41176=CARTESIAN_POINT('Ctrl Pts',(-0.271964569368884,0.000798153291622702,
0.288035430631116));
#41177=CARTESIAN_POINT('Ctrl Pts',(-0.269,4.16333634234434E-17,0.291));
#41178=CARTESIAN_POINT('Origin',(-0.295,-0.00699999999999998,0.04));
#41179=CARTESIAN_POINT('',(-0.274995262961565,-0.0016141092588829,0.285));
#41180=CARTESIAN_POINT('',(-0.274995262961565,-0.0016141092588829,0.1425));
#41181=CARTESIAN_POINT('Ctrl Pts',(-0.269,4.16333634234434E-17,0.291));
#41182=CARTESIAN_POINT('Ctrl Pts',(-0.271964569368901,-0.000798153291627193,
0.288035430631099));
#41183=CARTESIAN_POINT('Ctrl Pts',(-0.274995262961565,-0.00161410925888289,
0.285));
#41184=CARTESIAN_POINT('Origin',(-0.277715786349443,0.0489687861020745,
0.04));
#41185=CARTESIAN_POINT('',(-0.271097754137541,0.0461628389679575,0.04));
#41186=CARTESIAN_POINT('',(-0.27053717987482,0.0493420135926709,0.04));
#41187=CARTESIAN_POINT('Origin',(0.,0.,0.04));
#41188=CARTESIAN_POINT('',(-0.264913285560284,0.0467113597924044,0.04));
#41189=CARTESIAN_POINT('',(-0.29173382438227,0.0443325581406591,0.04));
#41190=CARTESIAN_POINT('',(-0.264913285560284,0.0467113597924044,0.04));
#41191=CARTESIAN_POINT('Origin',(-0.264913285560284,0.0467113597924044,
0.04));
#41192=CARTESIAN_POINT('',(-0.27053717987482,0.0493420135926709,0.285));
#41193=CARTESIAN_POINT('',(-0.27053717987482,0.0493420135926709,0.1425));
#41194=CARTESIAN_POINT('',(-0.264913285560284,0.0467113597924044,0.291));
#41195=CARTESIAN_POINT('',(-0.264913285560284,0.0467113597924044,0.04));
#41196=CARTESIAN_POINT('Ctrl Pts',(-0.27053717987482,0.0493420135926709,
0.285));
#41197=CARTESIAN_POINT('Ctrl Pts',(-0.267694218594536,0.0480121794105704,
0.288035430631093));
#41198=CARTESIAN_POINT('Ctrl Pts',(-0.264913285560284,0.0467113597924044,
0.291));
#41199=CARTESIAN_POINT('Origin',(-0.29173382438227,0.0443325581406591,0.04));
#41200=CARTESIAN_POINT('',(-0.271097754137541,0.0461628389679575,0.285));
#41201=CARTESIAN_POINT('',(-0.271097754137541,0.0461628389679575,0.1425));
#41202=CARTESIAN_POINT('Ctrl Pts',(-0.264913285560284,0.0467113597924044,
0.291));
#41203=CARTESIAN_POINT('Ctrl Pts',(-0.267971414323744,0.0464401243111915,
0.288035430631066));
#41204=CARTESIAN_POINT('Ctrl Pts',(-0.271097754137541,0.0461628389679575,
0.285));
#41205=CARTESIAN_POINT('Origin',(-0.264993319061626,0.0964496804178386,
0.04));
#41206=CARTESIAN_POINT('',(-0.25896307723613,0.09253715269228,0.04));
#41207=CARTESIAN_POINT('',(-0.257858961475997,0.095570685811709,0.04));
#41208=CARTESIAN_POINT('Origin',(0.,0.,0.04));
#41209=CARTESIAN_POINT('',(-0.252777314991409,0.0920034185546049,0.04));
#41210=CARTESIAN_POINT('',(-0.279603464135123,0.094318093935571,0.04));
#41211=CARTESIAN_POINT('',(-0.252777314991409,0.0920034185546049,0.04));
#41212=CARTESIAN_POINT('Origin',(-0.252777314991409,0.0920034185546049,
0.04));
#41213=CARTESIAN_POINT('',(-0.257858961475997,0.095570685811709,0.285));
#41214=CARTESIAN_POINT('',(-0.257858961475997,0.095570685811709,0.1425));
#41215=CARTESIAN_POINT('',(-0.252777314991409,0.0920034185546049,0.291));
#41216=CARTESIAN_POINT('',(-0.252777314991409,0.0920034185546049,0.04));
#41217=CARTESIAN_POINT('Ctrl Pts',(-0.257858961475997,0.095570685811709,
0.285));
#41218=CARTESIAN_POINT('Ctrl Pts',(-0.255290114447956,0.0937673797534397,
0.288035430631122));
#41219=CARTESIAN_POINT('Ctrl Pts',(-0.252777314991409,0.0920034185546049,
0.291));
#41220=CARTESIAN_POINT('Origin',(-0.279603464135123,0.094318093935571,0.04));
#41221=CARTESIAN_POINT('',(-0.25896307723613,0.09253715269228,0.285));
#41222=CARTESIAN_POINT('',(-0.25896307723613,0.09253715269228,0.1425));
#41223=CARTESIAN_POINT('Ctrl Pts',(-0.252777314991409,0.0920034185546049,
0.291));
#41224=CARTESIAN_POINT('Ctrl Pts',(-0.255836083454369,0.0922673422366571,
0.288035430631101));
#41225=CARTESIAN_POINT('Ctrl Pts',(-0.25896307723613,0.09253715269228,0.285));
#41226=CARTESIAN_POINT('Origin',(-0.244219163867212,0.141,0.04));
#41227=CARTESIAN_POINT('',(-0.238959938274539,0.136099771858106,0.04));
#41228=CARTESIAN_POINT('',(-0.237345829015656,0.138895491103459,0.04));
#41229=CARTESIAN_POINT('Origin',(0.,0.,0.04));
#41230=CARTESIAN_POINT('',(-0.232960833618014,0.1345,0.04));
#41231=CARTESIAN_POINT('',(-0.25897749411641,0.141437822173509,0.04));
#41232=CARTESIAN_POINT('',(-0.232960833618014,0.1345,0.04));
#41233=CARTESIAN_POINT('Origin',(-0.232960833618014,0.1345,0.04));
#41234=CARTESIAN_POINT('',(-0.237345829015656,0.138895491103459,0.285));
#41235=CARTESIAN_POINT('',(-0.237345829015656,0.138895491103459,0.1425));
#41236=CARTESIAN_POINT('',(-0.232960833618014,0.1345,0.291));
#41237=CARTESIAN_POINT('',(-0.232960833618014,0.1345,0.04));
#41238=CARTESIAN_POINT('Ctrl Pts',(-0.237345829015656,0.138895491103459,
0.285));
#41239=CARTESIAN_POINT('Ctrl Pts',(-0.23512914935695,0.136673505711114,
0.288035430631098));
#41240=CARTESIAN_POINT('Ctrl Pts',(-0.232960833618014,0.1345,0.291));
#41241=CARTESIAN_POINT('Origin',(-0.25897749411641,0.141437822173509,0.04));
#41242=CARTESIAN_POINT('',(-0.238959938274539,0.136099771858106,0.285));
#41243=CARTESIAN_POINT('',(-0.238959938274539,0.136099771858106,0.1425));
#41244=CARTESIAN_POINT('Ctrl Pts',(-0.232960833618014,0.1345,0.291));
#41245=CARTESIAN_POINT('Ctrl Pts',(-0.235927302648541,0.135291063657777,
0.288035430631136));
#41246=CARTESIAN_POINT('Ctrl Pts',(-0.238959938274539,0.136099771858106,
0.285));
#41247=CARTESIAN_POINT('Origin',(-0.216024532959552,0.181266105931604,0.04));
#41248=CARTESIAN_POINT('',(-0.211696122508039,0.175527068325832,0.04));
#41249=CARTESIAN_POINT('',(-0.209621063643459,0.17800002718254,0.04));
#41250=CARTESIAN_POINT('Origin',(0.,0.,0.04));
#41251=CARTESIAN_POINT('',(-0.206065955199005,0.172909867005679,0.04));
#41252=CARTESIAN_POINT('',(-0.230482623987904,0.184260033755696,0.04));
#41253=CARTESIAN_POINT('',(-0.206065955199005,0.172909867005679,0.04));
#41254=CARTESIAN_POINT('Origin',(-0.206065955199005,0.172909867005679,0.04));
#41255=CARTESIAN_POINT('',(-0.209621063643459,0.17800002718254,0.285));
#41256=CARTESIAN_POINT('',(-0.209621063643459,0.17800002718254,0.1425));
#41257=CARTESIAN_POINT('',(-0.206065955199005,0.172909867005679,0.291));
#41258=CARTESIAN_POINT('',(-0.206065955199005,0.172909867005679,0.04));
#41259=CARTESIAN_POINT('Ctrl Pts',(-0.209621063643459,0.17800002718254,
0.285));
#41260=CARTESIAN_POINT('Ctrl Pts',(-0.207823904043728,0.175426876357765,
0.288035430631226));
#41261=CARTESIAN_POINT('Ctrl Pts',(-0.206065955199005,0.172909867005679,
0.291));
#41262=CARTESIAN_POINT('Origin',(-0.230482623987904,0.184260033755696,0.04));
#41263=CARTESIAN_POINT('',(-0.211696122508039,0.175527068325832,0.285));
#41264=CARTESIAN_POINT('',(-0.211696122508039,0.175527068325832,0.1425));
#41265=CARTESIAN_POINT('Ctrl Pts',(-0.206065955199005,0.172909867005679,
0.291));
#41266=CARTESIAN_POINT('Ctrl Pts',(-0.208849990136858,0.174204034570293,
0.288035430631017));
#41267=CARTESIAN_POINT('Ctrl Pts',(-0.211696122508039,0.175527068325832,
0.285));
#41268=CARTESIAN_POINT('Origin',(-0.181266105931604,0.216024532959552,0.04));
#41269=CARTESIAN_POINT('',(-0.17800002718254,0.209621063643459,0.04));
#41270=CARTESIAN_POINT('',(-0.175527068325832,0.211696122508039,0.04));
#41271=CARTESIAN_POINT('Origin',(0.,0.,0.04));
#41272=CARTESIAN_POINT('',(-0.172909867005679,0.206065955199005,0.04));
#41273=CARTESIAN_POINT('',(-0.194984655959362,0.221483597452293,0.04));
#41274=CARTESIAN_POINT('',(-0.172909867005679,0.206065955199005,0.04));
#41275=CARTESIAN_POINT('Origin',(-0.172909867005679,0.206065955199005,0.04));
#41276=CARTESIAN_POINT('',(-0.175527068325832,0.211696122508039,0.285));
#41277=CARTESIAN_POINT('',(-0.175527068325832,0.211696122508039,0.1425));
#41278=CARTESIAN_POINT('',(-0.172909867005679,0.206065955199005,0.291));
#41279=CARTESIAN_POINT('',(-0.172909867005679,0.206065955199005,0.04));
#41280=CARTESIAN_POINT('Ctrl Pts',(-0.175527068325832,0.211696122508039,
0.285));
#41281=CARTESIAN_POINT('Ctrl Pts',(-0.174204034570238,0.208849990136741,
0.288035430631142));
#41282=CARTESIAN_POINT('Ctrl Pts',(-0.172909867005679,0.206065955199005,
0.291));
#41283=CARTESIAN_POINT('Origin',(-0.194984655959362,0.221483597452293,0.04));
#41284=CARTESIAN_POINT('',(-0.17800002718254,0.209621063643459,0.285));
#41285=CARTESIAN_POINT('',(-0.17800002718254,0.209621063643459,0.1425));
#41286=CARTESIAN_POINT('Ctrl Pts',(-0.172909867005679,0.206065955199005,
0.291));
#41287=CARTESIAN_POINT('Ctrl Pts',(-0.175426876357856,0.207823904043792,
0.288035430631119));
#41288=CARTESIAN_POINT('Ctrl Pts',(-0.17800002718254,0.209621063643459,
0.285));
#41289=CARTESIAN_POINT('Origin',(-0.141,0.244219163867212,0.04));
#41290=CARTESIAN_POINT('',(-0.138895491103459,0.237345829015656,0.04));
#41291=CARTESIAN_POINT('',(-0.136099771858106,0.238959938274539,0.04));
#41292=CARTESIAN_POINT('Origin',(0.,0.,0.04));
#41293=CARTESIAN_POINT('',(-0.1345,0.232960833618014,0.04));
#41294=CARTESIAN_POINT('',(-0.153562177826491,0.25197749411641,0.04));
#41295=CARTESIAN_POINT('',(-0.1345,0.232960833618014,0.04));
#41296=CARTESIAN_POINT('Origin',(-0.1345,0.232960833618014,0.04));
#41297=CARTESIAN_POINT('',(-0.136099771858106,0.238959938274539,0.285));
#41298=CARTESIAN_POINT('',(-0.136099771858106,0.238959938274539,0.1425));
#41299=CARTESIAN_POINT('',(-0.1345,0.232960833618014,0.291));
#41300=CARTESIAN_POINT('',(-0.1345,0.232960833618014,0.04));
#41301=CARTESIAN_POINT('Ctrl Pts',(-0.136099771858106,0.238959938274539,
0.285));
#41302=CARTESIAN_POINT('Ctrl Pts',(-0.135291063657772,0.235927302648521,
0.288035430631155));
#41303=CARTESIAN_POINT('Ctrl Pts',(-0.1345,0.232960833618014,0.291));
#41304=CARTESIAN_POINT('Origin',(-0.153562177826491,0.25197749411641,0.04));
#41305=CARTESIAN_POINT('',(-0.138895491103459,0.237345829015656,0.285));
#41306=CARTESIAN_POINT('',(-0.138895491103459,0.237345829015656,0.1425));
#41307=CARTESIAN_POINT('Ctrl Pts',(-0.1345,0.232960833618014,0.291));
#41308=CARTESIAN_POINT('Ctrl Pts',(-0.13667350571114,0.235129149356976,
0.288035430631063));
#41309=CARTESIAN_POINT('Ctrl Pts',(-0.138895491103459,0.237345829015656,
0.285));
#41310=CARTESIAN_POINT('Origin',(-0.0964496804178386,0.264993319061626,
0.04));
#41311=CARTESIAN_POINT('',(-0.095570685811709,0.257858961475997,0.04));
#41312=CARTESIAN_POINT('',(-0.09253715269228,0.25896307723613,0.04));
#41313=CARTESIAN_POINT('Origin',(0.,0.,0.04));
#41314=CARTESIAN_POINT('',(-0.0920034185546049,0.252777314991409,0.04));
#41315=CARTESIAN_POINT('',(-0.107473790626574,0.274815182128563,0.04));
#41316=CARTESIAN_POINT('',(-0.0920034185546049,0.252777314991409,0.04));
#41317=CARTESIAN_POINT('Origin',(-0.0920034185546049,0.252777314991409,
0.04));
#41318=CARTESIAN_POINT('',(-0.09253715269228,0.25896307723613,0.285));
#41319=CARTESIAN_POINT('',(-0.09253715269228,0.25896307723613,0.1425));
#41320=CARTESIAN_POINT('',(-0.0920034185546049,0.252777314991409,0.291));
#41321=CARTESIAN_POINT('',(-0.0920034185546049,0.252777314991409,0.04));
#41322=CARTESIAN_POINT('Ctrl Pts',(-0.09253715269228,0.25896307723613,0.285));
#41323=CARTESIAN_POINT('Ctrl Pts',(-0.0922673422366543,0.255836083454338,
0.288035430631132));
#41324=CARTESIAN_POINT('Ctrl Pts',(-0.0920034185546049,0.252777314991409,
0.291));
#41325=CARTESIAN_POINT('Origin',(-0.107473790626574,0.274815182128563,0.04));
#41326=CARTESIAN_POINT('',(-0.095570685811709,0.257858961475997,0.285));
#41327=CARTESIAN_POINT('',(-0.095570685811709,0.257858961475997,0.1425));
#41328=CARTESIAN_POINT('Ctrl Pts',(-0.0920034185546049,0.252777314991409,
0.291));
#41329=CARTESIAN_POINT('Ctrl Pts',(-0.0937673797534821,0.255290114448016,
0.288035430631051));
#41330=CARTESIAN_POINT('Ctrl Pts',(-0.0955706858117089,0.257858961475997,
0.285));
#41331=CARTESIAN_POINT('Origin',(-0.0489687861020744,0.277715786349443,
0.04));
#41332=CARTESIAN_POINT('',(-0.0493420135926708,0.27053717987482,0.04));
#41333=CARTESIAN_POINT('',(-0.0461628389679574,0.271097754137541,0.04));
#41334=CARTESIAN_POINT('Origin',(0.,0.,0.04));
#41335=CARTESIAN_POINT('',(-0.0467113597924043,0.264913285560284,0.04));
#41336=CARTESIAN_POINT('',(-0.0581198666828299,0.289302749894933,0.04));
#41337=CARTESIAN_POINT('',(-0.0467113597924043,0.264913285560284,0.04));
#41338=CARTESIAN_POINT('Origin',(-0.0467113597924043,0.264913285560284,
0.04));
#41339=CARTESIAN_POINT('',(-0.0461628389679574,0.271097754137541,0.285));
#41340=CARTESIAN_POINT('',(-0.0461628389679574,0.271097754137541,0.1425));
#41341=CARTESIAN_POINT('',(-0.0467113597924043,0.264913285560284,0.291));
#41342=CARTESIAN_POINT('',(-0.0467113597924043,0.264913285560284,0.04));
#41343=CARTESIAN_POINT('Ctrl Pts',(-0.0461628389679575,0.271097754137541,
0.285));
#41344=CARTESIAN_POINT('Ctrl Pts',(-0.0464401243112017,0.267971414323629,
0.288035430631178));
#41345=CARTESIAN_POINT('Ctrl Pts',(-0.0467113597924043,0.264913285560284,
0.291));
#41346=CARTESIAN_POINT('Origin',(-0.0581198666828299,0.289302749894933,
0.04));
#41347=CARTESIAN_POINT('',(-0.0493420135926708,0.27053717987482,0.285));
#41348=CARTESIAN_POINT('',(-0.0493420135926708,0.27053717987482,0.1425));
#41349=CARTESIAN_POINT('Ctrl Pts',(-0.0467113597924043,0.264913285560284,
0.291));
#41350=CARTESIAN_POINT('Ctrl Pts',(-0.0480121794105643,0.267694218594523,
0.288035430631107));
#41351=CARTESIAN_POINT('Ctrl Pts',(-0.0493420135926707,0.27053717987482,
0.285));
#41352=CARTESIAN_POINT('Origin',(1.38777878078145E-17,0.282,0.04));
#41353=CARTESIAN_POINT('',(-0.0016141092588829,0.274995262961565,0.04));
#41354=CARTESIAN_POINT('',(0.00161410925888293,0.274995262961565,0.04));
#41355=CARTESIAN_POINT('Origin',(0.,0.,0.04));
#41356=CARTESIAN_POINT('',(2.08166817117217E-17,0.269,0.04));
#41357=CARTESIAN_POINT('',(-0.00699999999999999,0.295,0.04));
#41358=CARTESIAN_POINT('',(2.08166817117217E-17,0.269,0.04));
#41359=CARTESIAN_POINT('Origin',(2.08166817117217E-17,0.269,0.04));
#41360=CARTESIAN_POINT('',(0.00161410925888295,0.274995262961565,0.285));
#41361=CARTESIAN_POINT('',(0.00161410925888295,0.274995262961565,0.1425));
#41362=CARTESIAN_POINT('',(2.08166817117217E-17,0.269,0.291));
#41363=CARTESIAN_POINT('',(2.08166817117217E-17,0.269,0.04));
#41364=CARTESIAN_POINT('Ctrl Pts',(0.00161410925888293,0.274995262961565,
0.285));
#41365=CARTESIAN_POINT('Ctrl Pts',(0.000798153291618306,0.271964569368868,
0.288035430631132));
#41366=CARTESIAN_POINT('Ctrl Pts',(2.08166817117217E-17,0.269,0.291));
#41367=CARTESIAN_POINT('Origin',(-0.00699999999999999,0.295,0.04));
#41368=CARTESIAN_POINT('',(-0.00161410925888292,0.274995262961565,0.285));
#41369=CARTESIAN_POINT('',(-0.00161410925888292,0.274995262961565,0.1425));
#41370=CARTESIAN_POINT('Ctrl Pts',(2.08166817117217E-17,0.269,0.291));
#41371=CARTESIAN_POINT('Ctrl Pts',(-0.000798153291634971,0.27196456936893,
0.28803543063107));
#41372=CARTESIAN_POINT('Ctrl Pts',(-0.00161410925888289,0.274995262961565,
0.285));
#41373=CARTESIAN_POINT('Origin',(0.0489687861020744,0.277715786349443,0.04));
#41374=CARTESIAN_POINT('',(0.0461628389679574,0.271097754137541,0.04));
#41375=CARTESIAN_POINT('',(0.0493420135926708,0.27053717987482,0.04));
#41376=CARTESIAN_POINT('Origin',(0.,0.,0.04));
#41377=CARTESIAN_POINT('',(0.0467113597924043,0.264913285560284,0.04));
#41378=CARTESIAN_POINT('',(0.044332558140659,0.29173382438227,0.04));
#41379=CARTESIAN_POINT('',(0.0467113597924043,0.264913285560284,0.04));
#41380=CARTESIAN_POINT('Origin',(0.0467113597924043,0.264913285560284,0.04));
#41381=CARTESIAN_POINT('',(0.0493420135926708,0.27053717987482,0.285));
#41382=CARTESIAN_POINT('',(0.0493420135926708,0.27053717987482,0.1425));
#41383=CARTESIAN_POINT('',(0.0467113597924043,0.264913285560284,0.291));
#41384=CARTESIAN_POINT('',(0.0467113597924043,0.264913285560284,0.04));
#41385=CARTESIAN_POINT('Ctrl Pts',(0.0493420135926708,0.27053717987482,
0.285));
#41386=CARTESIAN_POINT('Ctrl Pts',(0.048012179410518,0.267694218594424,
0.288035430631212));
#41387=CARTESIAN_POINT('Ctrl Pts',(0.0467113597924043,0.264913285560284,
0.291));
#41388=CARTESIAN_POINT('Origin',(0.044332558140659,0.29173382438227,0.04));
#41389=CARTESIAN_POINT('',(0.0461628389679575,0.271097754137541,0.285));
#41390=CARTESIAN_POINT('',(0.0461628389679575,0.271097754137541,0.1425));
#41391=CARTESIAN_POINT('Ctrl Pts',(0.0467113597924043,0.264913285560284,
0.291));
#41392=CARTESIAN_POINT('Ctrl Pts',(0.0464401243111968,0.267971414323684,
0.288035430631124));
#41393=CARTESIAN_POINT('Ctrl Pts',(0.0461628389679575,0.271097754137541,
0.285));
#41394=CARTESIAN_POINT('Origin',(0.0964496804178386,0.264993319061626,0.04));
#41395=CARTESIAN_POINT('',(0.09253715269228,0.25896307723613,0.04));
#41396=CARTESIAN_POINT('',(0.095570685811709,0.257858961475997,0.04));
#41397=CARTESIAN_POINT('Origin',(0.,0.,0.04));
#41398=CARTESIAN_POINT('',(0.0920034185546049,0.252777314991409,0.04));
#41399=CARTESIAN_POINT('',(0.094318093935571,0.279603464135123,0.04));
#41400=CARTESIAN_POINT('',(0.0920034185546049,0.252777314991409,0.04));
#41401=CARTESIAN_POINT('Origin',(0.0920034185546049,0.252777314991409,0.04));
#41402=CARTESIAN_POINT('',(0.095570685811709,0.257858961475997,0.285));
#41403=CARTESIAN_POINT('',(0.095570685811709,0.257858961475997,0.1425));
#41404=CARTESIAN_POINT('',(0.0920034185546049,0.252777314991409,0.291));
#41405=CARTESIAN_POINT('',(0.0920034185546049,0.252777314991409,0.04));
#41406=CARTESIAN_POINT('Ctrl Pts',(0.095570685811709,0.257858961475997,
0.285));
#41407=CARTESIAN_POINT('Ctrl Pts',(0.0937673797534397,0.255290114447956,
0.288035430631122));
#41408=CARTESIAN_POINT('Ctrl Pts',(0.0920034185546049,0.252777314991409,
0.291));
#41409=CARTESIAN_POINT('Origin',(0.094318093935571,0.279603464135123,0.04));
#41410=CARTESIAN_POINT('',(0.09253715269228,0.25896307723613,0.285));
#41411=CARTESIAN_POINT('',(0.09253715269228,0.25896307723613,0.1425));
#41412=CARTESIAN_POINT('Ctrl Pts',(0.0920034185546049,0.252777314991409,
0.291));
#41413=CARTESIAN_POINT('Ctrl Pts',(0.0922673422366571,0.255836083454369,
0.288035430631101));
#41414=CARTESIAN_POINT('Ctrl Pts',(0.09253715269228,0.25896307723613,0.285));
#41415=CARTESIAN_POINT('Origin',(0.141,0.244219163867212,0.04));
#41416=CARTESIAN_POINT('',(0.136099771858106,0.238959938274539,0.04));
#41417=CARTESIAN_POINT('',(0.138895491103459,0.237345829015656,0.04));
#41418=CARTESIAN_POINT('Origin',(0.,0.,0.04));
#41419=CARTESIAN_POINT('',(0.1345,0.232960833618014,0.04));
#41420=CARTESIAN_POINT('',(0.141437822173509,0.258977494116409,0.04));
#41421=CARTESIAN_POINT('',(0.1345,0.232960833618014,0.04));
#41422=CARTESIAN_POINT('Origin',(0.1345,0.232960833618014,0.04));
#41423=CARTESIAN_POINT('',(0.138895491103459,0.237345829015656,0.285));
#41424=CARTESIAN_POINT('',(0.138895491103459,0.237345829015656,0.1425));
#41425=CARTESIAN_POINT('',(0.1345,0.232960833618014,0.291));
#41426=CARTESIAN_POINT('',(0.1345,0.232960833618014,0.04));
#41427=CARTESIAN_POINT('Ctrl Pts',(0.138895491103459,0.237345829015656,
0.285));
#41428=CARTESIAN_POINT('Ctrl Pts',(0.136673505711127,0.235129149356963,
0.288035430631081));
#41429=CARTESIAN_POINT('Ctrl Pts',(0.1345,0.232960833618014,0.291));
#41430=CARTESIAN_POINT('Origin',(0.141437822173509,0.258977494116409,0.04));
#41431=CARTESIAN_POINT('',(0.136099771858106,0.238959938274539,0.285));
#41432=CARTESIAN_POINT('',(0.136099771858106,0.238959938274539,0.1425));
#41433=CARTESIAN_POINT('Ctrl Pts',(0.1345,0.232960833618014,0.291));
#41434=CARTESIAN_POINT('Ctrl Pts',(0.1352910636578,0.235927302648627,0.28803543063105));
#41435=CARTESIAN_POINT('Ctrl Pts',(0.136099771858106,0.238959938274539,
0.285));
#41436=CARTESIAN_POINT('Origin',(0.181266105931604,0.216024532959552,0.04));
#41437=CARTESIAN_POINT('',(0.175527068325832,0.211696122508039,0.04));
#41438=CARTESIAN_POINT('',(0.17800002718254,0.209621063643459,0.04));
#41439=CARTESIAN_POINT('Origin',(0.,0.,0.04));
#41440=CARTESIAN_POINT('',(0.172909867005679,0.206065955199005,0.04));
#41441=CARTESIAN_POINT('',(0.184260033755696,0.230482623987904,0.04));
#41442=CARTESIAN_POINT('',(0.172909867005679,0.206065955199005,0.04));
#41443=CARTESIAN_POINT('Origin',(0.172909867005679,0.206065955199005,0.04));
#41444=CARTESIAN_POINT('',(0.17800002718254,0.209621063643459,0.285));
#41445=CARTESIAN_POINT('',(0.17800002718254,0.209621063643459,0.1425));
#41446=CARTESIAN_POINT('',(0.172909867005679,0.206065955199005,0.291));
#41447=CARTESIAN_POINT('',(0.172909867005679,0.206065955199005,0.04));
#41448=CARTESIAN_POINT('Ctrl Pts',(0.17800002718254,0.209621063643459,0.285));
#41449=CARTESIAN_POINT('Ctrl Pts',(0.175426876357847,0.207823904043786,
0.28803543063113));
#41450=CARTESIAN_POINT('Ctrl Pts',(0.172909867005679,0.206065955199005,
0.291));
#41451=CARTESIAN_POINT('Origin',(0.184260033755696,0.230482623987904,0.04));
#41452=CARTESIAN_POINT('',(0.175527068325832,0.211696122508039,0.285));
#41453=CARTESIAN_POINT('',(0.175527068325832,0.211696122508039,0.1425));
#41454=CARTESIAN_POINT('Ctrl Pts',(0.172909867005679,0.206065955199005,
0.291));
#41455=CARTESIAN_POINT('Ctrl Pts',(0.174204034570257,0.208849990136781,
0.288035430631099));
#41456=CARTESIAN_POINT('Ctrl Pts',(0.175527068325832,0.211696122508039,
0.285));
#41457=CARTESIAN_POINT('Origin',(0.216024532959552,0.181266105931604,0.04));
#41458=CARTESIAN_POINT('',(0.209621063643459,0.17800002718254,0.04));
#41459=CARTESIAN_POINT('',(0.211696122508039,0.175527068325832,0.04));
#41460=CARTESIAN_POINT('Origin',(0.,0.,0.04));
#41461=CARTESIAN_POINT('',(0.206065955199005,0.172909867005679,0.04));
#41462=CARTESIAN_POINT('',(0.221483597452293,0.194984655959362,0.04));
#41463=CARTESIAN_POINT('',(0.206065955199005,0.172909867005679,0.04));
#41464=CARTESIAN_POINT('Origin',(0.206065955199005,0.172909867005679,0.04));
#41465=CARTESIAN_POINT('',(0.211696122508039,0.175527068325832,0.285));
#41466=CARTESIAN_POINT('',(0.211696122508039,0.175527068325832,0.1425));
#41467=CARTESIAN_POINT('',(0.206065955199005,0.172909867005679,0.291));
#41468=CARTESIAN_POINT('',(0.206065955199005,0.172909867005679,0.04));
#41469=CARTESIAN_POINT('Ctrl Pts',(0.211696122508039,0.175527068325832,
0.285));
#41470=CARTESIAN_POINT('Ctrl Pts',(0.208849990136656,0.174204034570199,
0.288035430631232));
#41471=CARTESIAN_POINT('Ctrl Pts',(0.206065955199005,0.172909867005679,
0.291));
#41472=CARTESIAN_POINT('Origin',(0.221483597452293,0.194984655959362,0.04));
#41473=CARTESIAN_POINT('',(0.209621063643459,0.17800002718254,0.285));
#41474=CARTESIAN_POINT('',(0.209621063643459,0.17800002718254,0.1425));
#41475=CARTESIAN_POINT('Ctrl Pts',(0.206065955199005,0.172909867005679,
0.291));
#41476=CARTESIAN_POINT('Ctrl Pts',(0.207823904043843,0.175426876357928,
0.288035430631034));
#41477=CARTESIAN_POINT('Ctrl Pts',(0.209621063643459,0.17800002718254,0.285));
#41478=CARTESIAN_POINT('Origin',(0.244219163867212,0.141,0.04));
#41479=CARTESIAN_POINT('',(0.237345829015656,0.138895491103459,0.04));
#41480=CARTESIAN_POINT('',(0.238959938274539,0.136099771858106,0.04));
#41481=CARTESIAN_POINT('Origin',(0.,0.,0.04));
#41482=CARTESIAN_POINT('',(0.232960833618014,0.1345,0.04));
#41483=CARTESIAN_POINT('',(0.25197749411641,0.153562177826491,0.04));
#41484=CARTESIAN_POINT('',(0.232960833618014,0.1345,0.04));
#41485=CARTESIAN_POINT('Origin',(0.232960833618014,0.1345,0.04));
#41486=CARTESIAN_POINT('',(0.238959938274539,0.136099771858106,0.285));
#41487=CARTESIAN_POINT('',(0.238959938274539,0.136099771858106,0.1425));
#41488=CARTESIAN_POINT('',(0.232960833618014,0.1345,0.291));
#41489=CARTESIAN_POINT('',(0.232960833618014,0.1345,0.04));
#41490=CARTESIAN_POINT('Ctrl Pts',(0.238959938274539,0.136099771858106,
0.285));
#41491=CARTESIAN_POINT('Ctrl Pts',(0.235927302648562,0.135291063657783,
0.288035430631114));
#41492=CARTESIAN_POINT('Ctrl Pts',(0.232960833618014,0.1345,0.291));
#41493=CARTESIAN_POINT('Origin',(0.25197749411641,0.153562177826491,0.04));
#41494=CARTESIAN_POINT('',(0.237345829015656,0.138895491103459,0.285));
#41495=CARTESIAN_POINT('',(0.237345829015656,0.138895491103459,0.1425));
#41496=CARTESIAN_POINT('Ctrl Pts',(0.232960833618014,0.1345,0.291));
#41497=CARTESIAN_POINT('Ctrl Pts',(0.235129149356992,0.136673505711156,
0.288035430631041));
#41498=CARTESIAN_POINT('Ctrl Pts',(0.237345829015656,0.138895491103459,
0.285));
#41499=CARTESIAN_POINT('Origin',(0.264993319061626,0.0964496804178386,0.04));
#41500=CARTESIAN_POINT('',(0.257858961475997,0.095570685811709,0.04));
#41501=CARTESIAN_POINT('',(0.25896307723613,0.09253715269228,0.04));
#41502=CARTESIAN_POINT('Origin',(0.,0.,0.04));
#41503=CARTESIAN_POINT('',(0.252777314991409,0.0920034185546049,0.04));
#41504=CARTESIAN_POINT('',(0.274815182128563,0.107473790626574,0.04));
#41505=CARTESIAN_POINT('',(0.252777314991409,0.0920034185546049,0.04));
#41506=CARTESIAN_POINT('Origin',(0.252777314991409,0.0920034185546049,0.04));
#41507=CARTESIAN_POINT('',(0.25896307723613,0.09253715269228,0.285));
#41508=CARTESIAN_POINT('',(0.25896307723613,0.09253715269228,0.1425));
#41509=CARTESIAN_POINT('',(0.252777314991409,0.0920034185546049,0.291));
#41510=CARTESIAN_POINT('',(0.252777314991409,0.0920034185546049,0.04));
#41511=CARTESIAN_POINT('Ctrl Pts',(0.25896307723613,0.09253715269228,0.285));
#41512=CARTESIAN_POINT('Ctrl Pts',(0.255836083454338,0.0922673422366543,
0.288035430631132));
#41513=CARTESIAN_POINT('Ctrl Pts',(0.252777314991409,0.0920034185546049,
0.291));
#41514=CARTESIAN_POINT('Origin',(0.274815182128563,0.107473790626574,0.04));
#41515=CARTESIAN_POINT('',(0.257858961475997,0.095570685811709,0.285));
#41516=CARTESIAN_POINT('',(0.257858961475997,0.095570685811709,0.1425));
#41517=CARTESIAN_POINT('Ctrl Pts',(0.252777314991409,0.0920034185546049,
0.291));
#41518=CARTESIAN_POINT('Ctrl Pts',(0.255290114448016,0.0937673797534821,
0.288035430631051));
#41519=CARTESIAN_POINT('Ctrl Pts',(0.257858961475997,0.0955706858117089,
0.285));
#41520=CARTESIAN_POINT('Origin',(0.277715786349443,0.0489687861020744,0.04));
#41521=CARTESIAN_POINT('',(0.27053717987482,0.0493420135926708,0.04));
#41522=CARTESIAN_POINT('',(0.271097754137541,0.0461628389679574,0.04));
#41523=CARTESIAN_POINT('Origin',(0.,0.,0.04));
#41524=CARTESIAN_POINT('',(0.264913285560284,0.0467113597924043,0.04));
#41525=CARTESIAN_POINT('',(0.289302749894933,0.0581198666828299,0.04));
#41526=CARTESIAN_POINT('',(0.264913285560284,0.0467113597924043,0.04));
#41527=CARTESIAN_POINT('Origin',(0.264913285560284,0.0467113597924043,0.04));
#41528=CARTESIAN_POINT('',(0.271097754137541,0.0461628389679574,0.285));
#41529=CARTESIAN_POINT('',(0.271097754137541,0.0461628389679574,0.1425));
#41530=CARTESIAN_POINT('',(0.264913285560284,0.0467113597924043,0.291));
#41531=CARTESIAN_POINT('',(0.264913285560284,0.0467113597924043,0.04));
#41532=CARTESIAN_POINT('Ctrl Pts',(0.271097754137541,0.0461628389679574,
0.285));
#41533=CARTESIAN_POINT('Ctrl Pts',(0.267971414323704,0.0464401243111951,
0.288035430631105));
#41534=CARTESIAN_POINT('Ctrl Pts',(0.264913285560284,0.0467113597924043,
0.291));
#41535=CARTESIAN_POINT('Origin',(0.289302749894933,0.0581198666828299,0.04));
#41536=CARTESIAN_POINT('',(0.27053717987482,0.0493420135926708,0.285));
#41537=CARTESIAN_POINT('',(0.27053717987482,0.0493420135926708,0.1425));
#41538=CARTESIAN_POINT('Ctrl Pts',(0.264913285560284,0.0467113597924043,
0.291));
#41539=CARTESIAN_POINT('Ctrl Pts',(0.26769421859449,0.0480121794105489,
0.288035430631142));
#41540=CARTESIAN_POINT('Ctrl Pts',(0.27053717987482,0.0493420135926708,
0.285));
#41541=CARTESIAN_POINT('Origin',(0.,0.,0.1425));
#41542=CARTESIAN_POINT('Origin',(0.,0.,0.285));
#41543=CARTESIAN_POINT('Origin',(0.,0.,0.285));
#41544=CARTESIAN_POINT('Origin',(0.,0.,0.285));
#41545=CARTESIAN_POINT('Origin',(0.,0.,0.285));
#41546=CARTESIAN_POINT('Origin',(0.,0.,0.285));
#41547=CARTESIAN_POINT('Origin',(0.,0.,0.285));
#41548=CARTESIAN_POINT('Origin',(0.,0.,0.285));
#41549=CARTESIAN_POINT('Origin',(0.,0.,0.285));
#41550=CARTESIAN_POINT('Origin',(0.,0.,0.285));
#41551=CARTESIAN_POINT('Origin',(0.,0.,0.285));
#41552=CARTESIAN_POINT('Origin',(0.,0.,0.285));
#41553=CARTESIAN_POINT('Origin',(0.,0.,0.285));
#41554=CARTESIAN_POINT('Origin',(0.,0.,0.285));
#41555=CARTESIAN_POINT('Origin',(0.,0.,0.285));
#41556=CARTESIAN_POINT('Origin',(0.,0.,0.285));
#41557=CARTESIAN_POINT('Origin',(0.,0.,0.285));
#41558=CARTESIAN_POINT('Origin',(0.,0.,0.285));
#41559=CARTESIAN_POINT('',(-0.275,-3.36777869765522E-17,0.));
#41560=CARTESIAN_POINT('',(-0.275,-3.36777869765522E-17,0.1425));
#41561=CARTESIAN_POINT('Origin',(0.,0.,0.));
#41562=CARTESIAN_POINT('Origin',(0.,0.,0.285));
#41563=CARTESIAN_POINT('Origin',(0.,0.,0.285));
#41564=CARTESIAN_POINT('Origin',(0.,0.,0.285));
#41565=CARTESIAN_POINT('Origin',(0.,0.,0.285));
#41566=CARTESIAN_POINT('Origin',(0.,0.,0.285));
#41567=CARTESIAN_POINT('Origin',(0.,0.,0.285));
#41568=CARTESIAN_POINT('Origin',(0.,0.,0.285));
#41569=CARTESIAN_POINT('Origin',(0.,0.,0.285));
#41570=CARTESIAN_POINT('Origin',(0.,0.,0.285));
#41571=CARTESIAN_POINT('Origin',(0.,0.,0.285));
#41572=CARTESIAN_POINT('Origin',(0.,0.,0.285));
#41573=CARTESIAN_POINT('Origin',(0.,0.,0.285));
#41574=CARTESIAN_POINT('Origin',(0.,0.,0.285));
#41575=CARTESIAN_POINT('Origin',(0.,0.,0.285));
#41576=CARTESIAN_POINT('Origin',(0.,0.,0.285));
#41577=CARTESIAN_POINT('Origin',(0.,0.,0.285));
#41578=CARTESIAN_POINT('Origin',(0.,0.,0.285));
#41579=CARTESIAN_POINT('',(0.274995262961565,0.00161410925888293,0.285));
#41580=CARTESIAN_POINT('Origin',(0.,0.,0.285));
#41581=CARTESIAN_POINT('',(0.274995262961565,0.00161410925888293,0.04));
#41582=CARTESIAN_POINT('',(0.274995262961565,0.00161410925888293,0.1425));
#41583=CARTESIAN_POINT('',(0.274995262961565,-0.00161410925888293,0.04));
#41584=CARTESIAN_POINT('Origin',(0.,0.,0.04));
#41585=CARTESIAN_POINT('',(0.274995262961565,-0.00161410925888293,0.285));
#41586=CARTESIAN_POINT('',(0.274995262961565,-0.00161410925888293,0.1425));
#41587=CARTESIAN_POINT('Origin',(0.,0.,0.285));
#41588=CARTESIAN_POINT('Origin',(0.269,0.,0.04));
#41589=CARTESIAN_POINT('',(0.269,0.,0.04));
#41590=CARTESIAN_POINT('',(0.269,0.,0.04));
#41591=CARTESIAN_POINT('',(0.269,0.,0.291));
#41592=CARTESIAN_POINT('',(0.269,0.,0.04));
#41593=CARTESIAN_POINT('Ctrl Pts',(0.274995262961565,-0.00161410925888293,
0.285));
#41594=CARTESIAN_POINT('Ctrl Pts',(0.271964569368838,-0.000798153291610108,
0.288035430631162));
#41595=CARTESIAN_POINT('Ctrl Pts',(0.269,0.,0.291));
#41596=CARTESIAN_POINT('Origin',(0.295,0.007,0.04));
#41597=CARTESIAN_POINT('Ctrl Pts',(0.269,0.,0.291));
#41598=CARTESIAN_POINT('Ctrl Pts',(0.27196456936891,0.000798153291629561,
0.28803543063109));
#41599=CARTESIAN_POINT('Ctrl Pts',(0.274995262961565,0.00161410925888293,
0.285));
#41600=CARTESIAN_POINT('',(0.295,0.007,0.04));
#41601=CARTESIAN_POINT('Origin',(0.282,0.,0.04));
#41602=CARTESIAN_POINT('Origin',(0.,0.,0.2925));
#41603=CARTESIAN_POINT('',(-0.26,-3.18408167778312E-17,0.3));
#41604=CARTESIAN_POINT('Origin',(0.,0.,0.3));
#41605=CARTESIAN_POINT('',(-0.2675,-3.27593018771917E-17,0.2925));
#41606=CARTESIAN_POINT('Origin',(0.,0.,0.134415608175648));
#41607=CARTESIAN_POINT('',(0.,0.,0.0978312163512968));
#41608=CARTESIAN_POINT('',(-0.113891921086774,1.39477376607661E-17,0.17));
#41609=CARTESIAN_POINT('',(-0.0577350269189626,-7.07050159149938E-18,0.134415608175648));
#41610=CARTESIAN_POINT('Origin',(0.,0.,0.17));
#41611=CARTESIAN_POINT('Origin',(0.,0.144337567297406,0.3));
#41612=CARTESIAN_POINT('',(8.83812698937423E-18,0.144337567297406,0.3));
#41613=CARTESIAN_POINT('',(0.125,0.0721687836487032,0.3));
#41614=CARTESIAN_POINT('',(0.03125,0.126295371385231,0.3));
#41615=CARTESIAN_POINT('',(1.38777878078145E-17,0.144337567297406,0.17));
#41616=CARTESIAN_POINT('',(8.83812698937423E-18,0.144337567297406,0.3));
#41617=CARTESIAN_POINT('',(0.125,0.0721687836487032,0.17));
#41618=CARTESIAN_POINT('',(0.125,0.0721687836487032,0.17));
#41619=CARTESIAN_POINT('',(0.125,0.0721687836487032,0.3));
#41620=CARTESIAN_POINT('Origin',(-0.125,0.0721687836487032,0.3));
#41621=CARTESIAN_POINT('',(-0.125,0.0721687836487032,0.3));
#41622=CARTESIAN_POINT('',(-0.09375,0.090210979560879,0.3));
#41623=CARTESIAN_POINT('',(-0.125,0.0721687836487032,0.17));
#41624=CARTESIAN_POINT('',(-0.125,0.0721687836487032,0.3));
#41625=CARTESIAN_POINT('',(8.83812698937423E-18,0.144337567297406,0.17));
#41626=CARTESIAN_POINT('Origin',(-0.125,-0.0721687836487032,0.3));
#41627=CARTESIAN_POINT('',(-0.125,-0.0721687836487032,0.3));
#41628=CARTESIAN_POINT('',(-0.125,-0.0360843918243516,0.3));
#41629=CARTESIAN_POINT('',(-0.125,-0.0721687836487032,0.17));
#41630=CARTESIAN_POINT('',(-0.125,-0.0721687836487032,0.3));
#41631=CARTESIAN_POINT('',(-0.125,0.0721687836487032,0.17));
#41632=CARTESIAN_POINT('Origin',(-2.77555756156289E-17,-0.144337567297406,
0.3));
#41633=CARTESIAN_POINT('',(-2.65143809681227E-17,-0.144337567297406,0.3));
#41634=CARTESIAN_POINT('',(-0.03125,-0.126295371385231,0.3));
#41635=CARTESIAN_POINT('',(-2.77555756156289E-17,-0.144337567297406,0.17));
#41636=CARTESIAN_POINT('',(-2.65143809681227E-17,-0.144337567297406,0.3));
#41637=CARTESIAN_POINT('',(-0.125,-0.0721687836487032,0.17));
#41638=CARTESIAN_POINT('Origin',(0.125,-0.0721687836487033,0.3));
#41639=CARTESIAN_POINT('',(0.125,-0.0721687836487033,0.3));
#41640=CARTESIAN_POINT('',(0.09375,-0.0902109795608791,0.3));
#41641=CARTESIAN_POINT('',(0.125,-0.0721687836487033,0.17));
#41642=CARTESIAN_POINT('',(0.125,-0.0721687836487033,0.3));
#41643=CARTESIAN_POINT('',(-2.65143809681227E-17,-0.144337567297406,0.17));
#41644=CARTESIAN_POINT('Origin',(0.125,0.0721687836487032,0.3));
#41645=CARTESIAN_POINT('',(0.125,0.0360843918243516,0.3));
#41646=CARTESIAN_POINT('',(0.125,-0.0721687836487033,0.17));
#41647=CARTESIAN_POINT('Origin',(0.,0.,0.17));
#41648=CARTESIAN_POINT('Origin',(0.114,0.,-0.8));
#41649=CARTESIAN_POINT('',(-0.114,-1.39609735102798E-17,-0.8));
#41650=CARTESIAN_POINT('Origin',(0.,0.,-0.8));
#41651=CARTESIAN_POINT('Origin',(0.,0.,-0.782));
#41652=CARTESIAN_POINT('',(-0.132,-1.61653377487451E-17,-0.782));
#41653=CARTESIAN_POINT('Origin',(0.,0.,-0.387));
#41654=CARTESIAN_POINT('Origin',(0.,0.,-0.01365));
#41655=CARTESIAN_POINT('Origin',(0.,0.,-0.005));
#41656=CARTESIAN_POINT('',(-0.16,-1.95943487863577E-17,-2.60208521396521E-18));
#41657=CARTESIAN_POINT('Origin',(0.,0.,0.));
#41658=CARTESIAN_POINT('',(-0.155,-1.8982025386784E-17,-0.005));
#41659=CARTESIAN_POINT('Origin',(0.275,0.,0.));
#41660=CARTESIAN_POINT('Origin',(0.,0.,0.3));
#53629=UNCERTAINTY_MEASURE_WITH_UNIT(LENGTH_MEASURE(0.001),#53651,
'DISTANCE_ACCURACY_VALUE',
'Maximum model space distance between geometric entities at asserted c
onnectivities');
#53632=UNCERTAINTY_MEASURE_WITH_UNIT(LENGTH_MEASURE(0.001),#53651,
'DISTANCE_ACCURACY_VALUE',
'Maximum model space distance between geometric entities at asserted c
onnectivities');
#53647=(
GEOMETRIC_REPRESENTATION_CONTEXT(3)
GLOBAL_UNCERTAINTY_ASSIGNED_CONTEXT((#53629))
GLOBAL_UNIT_ASSIGNED_CONTEXT((#53651,#53653,#53654))
REPRESENTATION_CONTEXT('','3D')
);
#53650=(
GEOMETRIC_REPRESENTATION_CONTEXT(3)
GLOBAL_UNCERTAINTY_ASSIGNED_CONTEXT((#53632))
GLOBAL_UNIT_ASSIGNED_CONTEXT((#53651,#53653,#53654))
REPRESENTATION_CONTEXT('','3D')
);
#53651=(
LENGTH_UNIT()
NAMED_UNIT(*)
SI_UNIT(.CENTI.,.METRE.)
);
#53653=(
NAMED_UNIT(*)
PLANE_ANGLE_UNIT()
SI_UNIT($,.RADIAN.)
);
#53654=(
NAMED_UNIT(*)
SI_UNIT($,.STERADIAN.)
SOLID_ANGLE_UNIT()
);
#53669=SHAPE_DEFINITION_REPRESENTATION(#53686,#53737);
#53686=PRODUCT_DEFINITION_SHAPE('',$,#53755);
#53737=SHAPE_REPRESENTATION('',(#24795),#53647);
#53740=PRODUCT_DEFINITION_CONTEXT('part definition',#53793,'design');
#53755=PRODUCT_DEFINITION('2026-10-18-22-45-05-226',
'14_ISO_4762_M3x8_A2',#53772,#53740);
#53772=PRODUCT_DEFINITION_FORMATION('',$,#53809);
#53793=APPLICATION_CONTEXT(
'Core Data for Automotive Mechanical Design Process');
#53794=PRODUCT_CONTEXT('part definition',#53793,'mechanical');
#53809=PRODUCT('2026-10-18-22-45-05-226','14_ISO_4762_M3x8_A2',$,(#53794));
#53959=COLOUR_RGB('Black',0.12,0.14,0.17);
#53960=FILL_AREA_STYLE_COLOUR('',#53959);
#53961=FILL_AREA_STYLE('',(#53960));
#53962=SURFACE_STYLE_FILL_AREA(#53961);
#53963=SURFACE_SIDE_STYLE('',(#53962));
#53964=SURFACE_STYLE_USAGE(.BOTH.,#53963);
#53965=PRESENTATION_STYLE_ASSIGNMENT((#53964));
ENDSEC;
END-ISO-10303-21;
